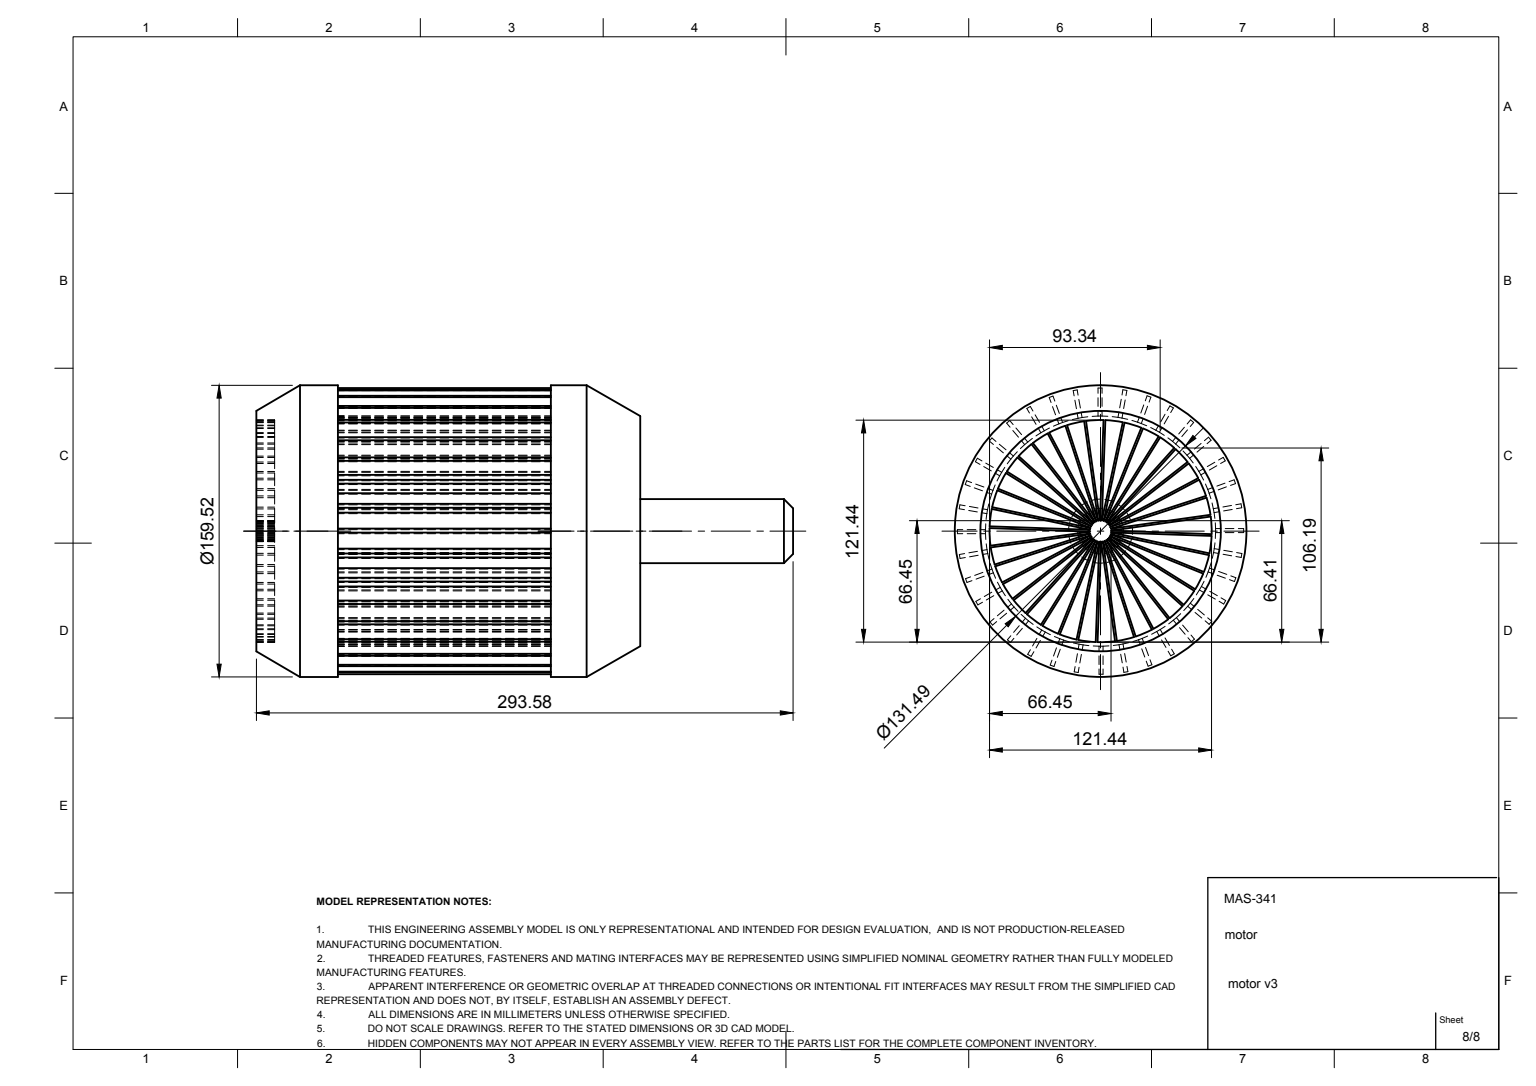
ISO-10303-21;
HEADER;
FILE_DESCRIPTION (('STEP AP214'),
    '1' );
FILE_NAME ('MOTOR.step',
    '2026-10-08T00:39:10',
    ( '' ),
    ( '' ),
    'SwSTEP 2.0',
    'SolidWorks 2025',
    '' );
FILE_SCHEMA (( 'AUTOMOTIVE_DESIGN' ));
ENDSEC;

DATA;
#1=VERTEX_POINT ( 'NONE', #4469 ) ;
#3=DIRECTION ( 'NONE',  ( 0.000000000000000000, 0.000000000000000000, 1.000000000000000000 ) ) ;
#6=EDGE_CURVE ( 'NONE', #9325, #3604, #16957, .T. ) ;
#8=AXIS2_PLACEMENT_3D ( 'NONE', #20241, #7754, #6443 ) ;
#11=LINE ( 'NONE', #3084, #15099 ) ;
#13=DIRECTION ( 'NONE',  ( 1.000000000000000000, 0.000000000000000000, 0.000000000000000000 ) ) ;
#14=CARTESIAN_POINT ( 'NONE',  ( 1.379293853801755176, -58.69016442926522359, 112.7772637782949943 ) ) ;
#17=VERTEX_POINT ( 'NONE', #1406 ) ;
#18=LINE ( 'NONE', #19855, #18549 ) ;
#19=CARTESIAN_POINT ( 'NONE',  ( -47.56244194535165803, -37.78198917157333625, 283.5832628385307999 ) ) ;
#20=ORIENTED_EDGE ( 'NONE', *, *, #18426, .T. ) ;
#21=ORIENTED_EDGE ( 'NONE', *, *, #3297, .T. ) ;
#23=EDGE_CURVE ( 'NONE', #17780, #6819, #12333, .T. ) ;
#27=FACE_BOUND ( 'NONE', #13868, .T. ) ;
#28=ORIENTED_EDGE ( 'NONE', *, *, #7214, .F. ) ;
#34=EDGE_CURVE ( 'NONE', #17780, #13430, #14084, .T. ) ;
#36=DIRECTION ( 'NONE',  ( 1.000000000000000000, 0.000000000000000000, 0.000000000000000000 ) ) ;
#37=EDGE_CURVE ( 'NONE', #15836, #9172, #3251, .T. ) ;
#40=DIRECTION ( 'NONE',  ( -0.9396926207859104263, 0.3420201433256630508, 0.000000000000000000 ) ) ;
#43=ADVANCED_FACE ( 'NONE', ( #7739 ), #8149, .F. ) ;
#45=VECTOR ( 'NONE', #980, 1000.000000000000000 ) ;
#48=VERTEX_POINT ( 'NONE', #12848 ) ;
#50=ORIENTED_EDGE ( 'NONE', *, *, #6042, .F. ) ;
#52=CYLINDRICAL_SURFACE ( 'NONE', #15157, 62.91752772691707207 ) ;
#53=CARTESIAN_POINT ( 'NONE',  ( 19.23677882349201695, -57.61823435390814296, 283.5832628385307999 ) ) ;
#54=DIRECTION ( 'NONE',  ( -0.3747554100459959403, -0.9271237148521535021, 0.000000000000000000 ) ) ;
#55=VERTEX_POINT ( 'NONE', #19106 ) ;
#60=DIRECTION ( 'NONE',  ( -0.000000000000000000, -0.000000000000000000, 1.000000000000000000 ) ) ;
#61=EDGE_CURVE ( 'NONE', #5572, #2811, #1813, .T. ) ;
#67=ORIENTED_EDGE ( 'NONE', *, *, #294, .F. ) ;
#71=ORIENTED_EDGE ( 'NONE', *, *, #11636, .F. ) ;
#72=PLANE ( 'NONE',  #545 ) ;
#73=DIRECTION ( 'NONE',  ( 1.000000000000000000, 0.000000000000000000, 0.000000000000000000 ) ) ;
#75=LINE ( 'NONE', #4042, #2106 ) ;
#77=ORIENTED_EDGE ( 'NONE', *, *, #15533, .T. ) ;
#79=LINE ( 'NONE', #15635, #4891 ) ;
#81=UNCERTAINTY_MEASURE_WITH_UNIT (LENGTH_MEASURE( 1.000000000000000082E-05 ), #12072, 'distance_accuracy_value', 'NONE');
#91=ORIENTED_EDGE ( 'NONE', *, *, #10595, .F. ) ;
#93=VERTEX_POINT ( 'NONE', #12647 ) ;
#94=VECTOR ( 'NONE', #4205, 1000.000000000000000 ) ;
#96=FACE_OUTER_BOUND ( 'NONE', #8145, .T. ) ;
#97=EDGE_CURVE ( 'NONE', #13695, #10750, #5094, .T. ) ;
#99=FACE_OUTER_BOUND ( 'NONE', #15672, .T. ) ;
#101=ORIENTED_EDGE ( 'NONE', *, *, #14389, .F. ) ;
#103=CARTESIAN_POINT ( 'NONE',  ( 0.000000000000000000, 0.000000000000000000, 283.5832628385307999 ) ) ;
#108=VERTEX_POINT ( 'NONE', #3347 ) ;
#109=CARTESIAN_POINT ( 'NONE',  ( 79.75827554147308263, 0.000000000000000000, 112.9440587442963562 ) ) ;
#110=CYLINDRICAL_SURFACE ( 'NONE', #6774, 62.91752772691707207 ) ;
#113=ORIENTED_EDGE ( 'NONE', *, *, #2779, .F. ) ;
#116=AXIS2_PLACEMENT_3D ( 'NONE', #3572, #14207, #6645 ) ;
#118=EDGE_LOOP ( 'NONE', ( #19896, #4440, #15908, #1948 ) ) ;
#122=AXIS2_PLACEMENT_3D ( 'NONE', #14861, #16210, #14669 ) ;
#123=EDGE_LOOP ( 'NONE', ( #19058, #8519, #18483, #4308 ) ) ;
#124=ADVANCED_FACE ( 'NONE', ( #3050 ), #72, .T. ) ;
#125=CARTESIAN_POINT ( 'NONE',  ( 28.06680738835026290, -53.87178215532764369, 293.5832628385307999 ) ) ;
#126=LINE ( 'NONE', #5341, #13935 ) ;
#129=FACE_OUTER_BOUND ( 'NONE', #6146, .T. ) ;
#133=LINE ( 'NONE', #6488, #17538 ) ;
#137=VECTOR ( 'NONE', #8001, 1000.000000000000000 ) ;
#139=PLANE ( 'NONE',  #10813 ) ;
#142=DIRECTION ( 'NONE',  ( -0.000000000000000000, -0.000000000000000000, 1.000000000000000000 ) ) ;
#144=ORIENTED_EDGE ( 'NONE', *, *, #11299, .F. ) ;
#145=EDGE_CURVE ( 'NONE', #10155, #5152, #9485, .T. ) ;
#146=ADVANCED_FACE ( 'NONE', ( #6627 ), #17167, .F. ) ;
#148=ADVANCED_FACE ( 'NONE', ( #7839 ), #6224, .F. ) ;
#151=AXIS2_PLACEMENT_3D ( 'NONE', #5744, #3184, #10529 ) ;
#154=LINE ( 'NONE', #15601, #13008 ) ;
#155=DIRECTION ( 'NONE',  ( 0.000000000000000000, 0.000000000000000000, 1.000000000000000000 ) ) ;
#157=EDGE_CURVE ( 'NONE', #11944, #5361, #6437, .T. ) ;
#158=LINE ( 'NONE', #9470, #15417 ) ;
#159=DIRECTION ( 'NONE',  ( -0.000000000000000000, -0.000000000000000000, 1.000000000000000000 ) ) ;
#161=AXIS2_PLACEMENT_3D ( 'NONE', #19945, #4400, #6050 ) ;
#162=CARTESIAN_POINT ( 'NONE',  ( 0.000000000000000000, 0.000000000000000000, 283.5832628385307999 ) ) ;
#163=ORIENTED_EDGE ( 'NONE', *, *, #16525, .F. ) ;
#168=EDGE_CURVE ( 'NONE', #13542, #6667, #19206, .T. ) ;
#169=ORIENTED_EDGE ( 'NONE', *, *, #10850, .T. ) ;
#170=LINE ( 'NONE', #6528, #17757 ) ;
#171=ORIENTED_EDGE ( 'NONE', *, *, #16914, .T. ) ;
#172=CARTESIAN_POINT ( 'NONE',  ( 51.23821591265094355, 28.63313560863489471, 132.4711112102474146 ) ) ;
#174=EDGE_CURVE ( 'NONE', #2962, #5478, #10345, .T. ) ;
#175=DIRECTION ( 'NONE',  ( -0.000000000000000000, -0.000000000000000000, 1.000000000000000000 ) ) ;
#177=CARTESIAN_POINT ( 'NONE',  ( 44.79940644582654841, -41.02350267428983699, 293.5832628385307999 ) ) ;
#179=ORIENTED_EDGE ( 'NONE', *, *, #8168, .F. ) ;
#181=CARTESIAN_POINT ( 'NONE',  ( -57.92514141135452377, -18.28503710798565152, 293.5832628385307999 ) ) ;
#182=VERTEX_POINT ( 'NONE', #8245 ) ;
#184=DIRECTION ( 'NONE',  ( -0.000000000000000000, -0.000000000000000000, 1.000000000000000000 ) ) ;
#185=VECTOR ( 'NONE', #17338, 999.9999999999998863 ) ;
#186=DIRECTION ( 'NONE',  ( 0.4999999999999978906, 0.8660254037844397068, 0.000000000000000000 ) ) ;
#192=ORIENTED_EDGE ( 'NONE', *, *, #7035, .T. ) ;
#194=DIRECTION ( 'NONE',  ( 0.000000000000000000, 0.000000000000000000, -1.000000000000000000 ) ) ;
#195=VERTEX_POINT ( 'NONE', #2590 ) ;
#197=DIRECTION ( 'NONE',  ( -0.000000000000000000, -0.000000000000000000, 1.000000000000000000 ) ) ;
#198=CARTESIAN_POINT ( 'NONE',  ( 25.99419088092191643, -73.82206860051539365, 248.9926560891072143 ) ) ;
#199=EDGE_LOOP ( 'NONE', ( #8551, #11635, #6168 ) ) ;
#200=DIRECTION ( 'NONE',  ( 0.000000000000000000, 0.000000000000000000, 1.000000000000000000 ) ) ;
#201=DIRECTION ( 'NONE',  ( -0.000000000000000000, -0.000000000000000000, 1.000000000000000000 ) ) ;
#202=DIRECTION ( 'NONE',  ( -0.6427876096865458022, 0.7660444431189726844, 0.000000000000000000 ) ) ;
#203=LINE ( 'NONE', #14432, #8189 ) ;
#207=FACE_OUTER_BOUND ( 'NONE', #7256, .T. ) ;
#209=LINE ( 'NONE', #17715, #417 ) ;
#210=ORIENTED_EDGE ( 'NONE', *, *, #884, .F. ) ;
#211=VECTOR ( 'NONE', #4896, 1000.000000000000114 ) ;
#214=ORIENTED_EDGE ( 'NONE', *, *, #634, .F. ) ;
#216=VECTOR ( 'NONE', #7323, 999.9999999999998863 ) ;
#217=ORIENTED_EDGE ( 'NONE', *, *, #13252, .T. ) ;
#219=VERTEX_POINT ( 'NONE', #7381 ) ;
#221=LINE ( 'NONE', #125, #3582 ) ;
#223=ORIENTED_EDGE ( 'NONE', *, *, #17123, .T. ) ;
#229=FACE_OUTER_BOUND ( 'NONE', #16622, .T. ) ;
#233=CIRCLE ( 'NONE', #865, 60.74260934110282051 ) ;
#234=EDGE_CURVE ( 'NONE', #6701, #18758, #15059, .T. ) ;
#238=PLANE ( 'NONE',  #10473 ) ;
#241=VERTEX_POINT ( 'NONE', #4112 ) ;
#243=CARTESIAN_POINT ( 'NONE',  ( -55.43188410062182925, -19.30071112029661151, 248.9926560891072143 ) ) ;
#244=VERTEX_POINT ( 'NONE', #16407 ) ;
#246=ORIENTED_EDGE ( 'NONE', *, *, #6218, .F. ) ;
#247=EDGE_CURVE ( 'NONE', #18829, #4599, #4215, .T. ) ;
#249=AXIS2_PLACEMENT_3D ( 'NONE', #15715, #7622, #7927 ) ;
#252=CARTESIAN_POINT ( 'NONE',  ( 0.000000000000000000, 0.000000000000000000, 293.5832628385307999 ) ) ;
#253=CARTESIAN_POINT ( 'NONE',  ( -3.911853314815645799, 4.196299268919075232, 293.5832628385307999 ) ) ;
#255=DIRECTION ( 'NONE',  ( 1.000000000000000000, 0.000000000000000000, 0.000000000000000000 ) ) ;
#256=DIRECTION ( 'NONE',  ( -0.000000000000000000, -0.000000000000000000, 1.000000000000000000 ) ) ;
#257=FACE_OUTER_BOUND ( 'NONE', #10692, .T. ) ;
#261=AXIS2_PLACEMENT_3D ( 'NONE', #5388, #13050, #3942 ) ;
#263=ORIENTED_EDGE ( 'NONE', *, *, #10525, .T. ) ;
#264=AXIS2_PLACEMENT_3D ( 'NONE', #15615, #1602, #16694 ) ;
#268=ORIENTED_EDGE ( 'NONE', *, *, #10367, .T. ) ;
#271=DIRECTION ( 'NONE',  ( -0.9511061040868794558, -0.3088643371590157338, 0.000000000000000000 ) ) ;
#273=VECTOR ( 'NONE', #15752, 1000.000000000000000 ) ;
#274=VERTEX_POINT ( 'NONE', #2392 ) ;
#276=VECTOR ( 'NONE', #14469, 1000.000000000000000 ) ;
#279=PLANE ( 'NONE',  #19707 ) ;
#280=CARTESIAN_POINT ( 'NONE',  ( 57.61823435390807902, 19.23677882349220880, 293.5832628385307999 ) ) ;
#285=CARTESIAN_POINT ( 'NONE',  ( -0.8220851292435327196, -62.91215678473957240, 132.4711112102474146 ) ) ;
#286=DIRECTION ( 'NONE',  ( -0.8660254037844345998, -0.5000000000000069944, 0.000000000000000000 ) ) ;
#288=CARTESIAN_POINT ( 'NONE',  ( 62.09913334491125170, 10.11498556985180208, 132.4711112102474146 ) ) ;
#289=LINE ( 'NONE', #19024, #1463 ) ;
#290=CARTESIAN_POINT ( 'NONE',  ( 55.43188410062170135, 19.30071112029698455, 248.9926560891072143 ) ) ;
#292=FACE_OUTER_BOUND ( 'NONE', #9039, .T. ) ;
#294=EDGE_CURVE ( 'NONE', #11013, #2211, #842, .T. ) ;
#296=VECTOR ( 'NONE', #6808, 1000.000000000000114 ) ;
#297=DIRECTION ( 'NONE',  ( 1.000000000000000000, 0.000000000000000000, 0.000000000000000000 ) ) ;
#298=ORIENTED_EDGE ( 'NONE', *, *, #10704, .T. ) ;
#299=ORIENTED_EDGE ( 'NONE', *, *, #9841, .T. ) ;
#305=EDGE_LOOP ( 'NONE', ( #2327, #8715, #1443, #6118 ) ) ;
#311=LINE ( 'NONE', #12579, #10853 ) ;
#312=CARTESIAN_POINT ( 'NONE',  ( 57.61823435390807902, 19.23677882349220880, 293.5832628385307999 ) ) ;
#319=AXIS2_PLACEMENT_3D ( 'NONE', #17195, #12465, #6453 ) ;
#320=VECTOR ( 'NONE', #3029, 1000.000000000000000 ) ;
#321=VERTEX_POINT ( 'NONE', #7094 ) ;
#325=CARTESIAN_POINT ( 'NONE',  ( -19.23614321207235278, 57.61627707419557964, 283.5832628385307999 ) ) ;
#327=ORIENTED_EDGE ( 'NONE', *, *, #9501, .F. ) ;
#329=DIRECTION ( 'NONE',  ( -0.3420201433256601087, -0.9396926207859114255, 0.000000000000000000 ) ) ;
#332=CIRCLE ( 'NONE', #12417, 60.74260934110282051 ) ;
#337=LINE ( 'NONE', #14255, #1684 ) ;
#338=DIRECTION ( 'NONE',  ( 1.000000000000000000, 0.000000000000000000, 0.000000000000000000 ) ) ;
#340=EDGE_CURVE ( 'NONE', #18152, #7860, #943, .T. ) ;
#341=ORIENTED_EDGE ( 'NONE', *, *, #8132, .T. ) ;
#342=DIRECTION ( 'NONE',  ( -0.000000000000000000, -0.000000000000000000, 1.000000000000000000 ) ) ;
#343=ORIENTED_EDGE ( 'NONE', *, *, #631, .F. ) ;
#347=VERTEX_POINT ( 'NONE', #3651 ) ;
#348=EDGE_CURVE ( 'NONE', #14755, #3199, #18041, .T. ) ;
#350=LINE ( 'NONE', #4765, #14650 ) ;
#351=DIRECTION ( 'NONE',  ( -0.000000000000000000, -0.000000000000000000, 1.000000000000000000 ) ) ;
#355=CARTESIAN_POINT ( 'NONE',  ( 68.18670162478805707, 38.41834839689404646, 248.9926560891072143 ) ) ;
#357=CARTESIAN_POINT ( 'NONE',  ( 44.79787735033391272, -41.02212542604626577, 293.5832628385307999 ) ) ;
#360=EDGE_CURVE ( 'NONE', #2215, #19198, #19663, .T. ) ;
#361=ORIENTED_EDGE ( 'NONE', *, *, #7399, .T. ) ;
#363=DIRECTION ( 'NONE',  ( -0.9511061040868794558, -0.3088643371590157338, 0.000000000000000000 ) ) ;
#364=ORIENTED_EDGE ( 'NONE', *, *, #5614, .T. ) ;
#366=ORIENTED_EDGE ( 'NONE', *, *, #2785, .T. ) ;
#369=VECTOR ( 'NONE', #15962, 1000.000000000000000 ) ;
#370=EDGE_CURVE ( 'NONE', #6318, #12537, #20174, .T. ) ;
#374=AXIS2_PLACEMENT_3D ( 'NONE', #8108, #8211, #6887 ) ;
#376=EDGE_CURVE ( 'NONE', #12874, #17522, #10545, .T. ) ;
#382=CARTESIAN_POINT ( 'NONE',  ( -61.81362617575094021, 11.73417718768112294, 132.4711112102474146 ) ) ;
#384=CARTESIAN_POINT ( 'NONE',  ( 54.07248341783252954, -32.16802499836759921, 293.5832628385307999 ) ) ;
#385=CARTESIAN_POINT ( 'NONE',  ( 0.000000000000000000, 0.000000000000000000, 112.9440587442963562 ) ) ;
#386=DIRECTION ( 'NONE',  ( 1.000000000000000000, 0.000000000000000000, 0.000000000000000000 ) ) ;
#391=CARTESIAN_POINT ( 'NONE',  ( 0.000000000000000000, 0.000000000000000000, 283.5832628385307999 ) ) ;
#396=ORIENTED_EDGE ( 'NONE', *, *, #18390, .F. ) ;
#399=VERTEX_POINT ( 'NONE', #1458 ) ;
#400=ADVANCED_FACE ( 'NONE', ( #1248, #13721, #13823, #16903, #5862, #12074, #18338, #2794, #5963, #1667, #7484, #27, #3201, #9331, #6177, #16802, #18542, #15470, #12492, #4312, #4420, #19964, #12394, #18653, #4632, #18756, #12183, #7687, #7894, #10650, #10757, #18441, #7798, #9121, #15363, #1355, #7582 ), #17011, .F. ) ;
#401=EDGE_CURVE ( 'NONE', #5555, #4348, #6279, .T. ) ;
#404=ORIENTED_EDGE ( 'NONE', *, *, #17763, .T. ) ;
#407=DIRECTION ( 'NONE',  ( 0.5300553768524375320, 0.8479630283625697595, 0.000000000000000000 ) ) ;
#408=CARTESIAN_POINT ( 'NONE',  ( 49.07263256785952876, -39.37628763770437956, 248.9926560891072143 ) ) ;
#412=DIRECTION ( 'NONE',  ( 0.3420201433256790380, -0.9396926207859046531, 0.000000000000000000 ) ) ;
#413=ORIENTED_EDGE ( 'NONE', *, *, #34, .T. ) ;
#416=CARTESIAN_POINT ( 'NONE',  ( -11.73417718768092399, -61.81362617575098994, 132.4711112102474146 ) ) ;
#417=VECTOR ( 'NONE', #16178, 1000.000000000000227 ) ;
#421=ORIENTED_EDGE ( 'NONE', *, *, #14487, .F. ) ;
#425=ORIENTED_EDGE ( 'NONE', *, *, #14850, .T. ) ;
#426=ORIENTED_EDGE ( 'NONE', *, *, #9892, .F. ) ;
#430=EDGE_CURVE ( 'NONE', #13898, #11413, #14350, .T. ) ;
#432=CARTESIAN_POINT ( 'NONE',  ( -68.18670162478832708, -38.41834839689356329, 248.9926560891072143 ) ) ;
#434=ORIENTED_EDGE ( 'NONE', *, *, #4227, .F. ) ;
#439=VECTOR ( 'NONE', #2770, 1000.000000000000114 ) ;
#444=VECTOR ( 'NONE', #7066, 1000.000000000000000 ) ;
#445=VECTOR ( 'NONE', #5247, 1000.000000000000000 ) ;
#449=ORIENTED_EDGE ( 'NONE', *, *, #634, .T. ) ;
#452=ORIENTED_EDGE ( 'NONE', *, *, #4347, .T. ) ;
#454=ORIENTED_EDGE ( 'NONE', *, *, #3182, .F. ) ;
#457=EDGE_CURVE ( 'NONE', #4545, #10038, #17552, .T. ) ;
#459=LINE ( 'NONE', #2301, #5504 ) ;
#461=CARTESIAN_POINT ( 'NONE',  ( -47.66508197439445382, 41.06890862491522398, 132.4711112102474146 ) ) ;
#462=CARTESIAN_POINT ( 'NONE',  ( 22.81000261549368346, -58.63718168490493099, 132.4711112102474146 ) ) ;
#463=DIRECTION ( 'NONE',  ( -0.000000000000000000, -0.000000000000000000, 1.000000000000000000 ) ) ;
#467=FACE_OUTER_BOUND ( 'NONE', #12951, .T. ) ;
#468=ORIENTED_EDGE ( 'NONE', *, *, #8040, .F. ) ;
#469=ADVANCED_FACE ( 'NONE', ( #4843 ), #3306, .F. ) ;
#470=DIRECTION ( 'NONE',  ( 0.000000000000000000, 0.000000000000000000, 1.000000000000000000 ) ) ;
#472=EDGE_LOOP ( 'NONE', ( #15073, #6600, #4290, #1623 ) ) ;
#474=ORIENTED_EDGE ( 'NONE', *, *, #16234, .F. ) ;
#475=VECTOR ( 'NONE', #10571, 1000.000000000000114 ) ;
#477=DIRECTION ( 'NONE',  ( 0.000000000000000000, 0.000000000000000000, -1.000000000000000000 ) ) ;
#479=LINE ( 'NONE', #10910, #17442 ) ;
#480=EDGE_CURVE ( 'NONE', #10080, #12789, #2077, .T. ) ;
#481=CARTESIAN_POINT ( 'NONE',  ( 39.84224160888901167, 67.36461649554546227, 110.9660488491356887 ) ) ;
#486=ORIENTED_EDGE ( 'NONE', *, *, #8858, .T. ) ;
#487=CARTESIAN_POINT ( 'NONE',  ( 0.000000000000000000, 0.000000000000000000, 293.5832628385307999 ) ) ;
#488=CARTESIAN_POINT ( 'NONE',  ( 12.78021302872850562, -77.21438937758507848, 112.0427633081291816 ) ) ;
#490=DIRECTION ( 'NONE',  ( 0.000000000000000000, 0.000000000000000000, -1.000000000000000000 ) ) ;
#492=EDGE_CURVE ( 'NONE', #11539, #4753, #17531, .T. ) ;
#493=EDGE_CURVE ( 'NONE', #14511, #9172, #1973, .T. ) ;
#495=DIRECTION ( 'NONE',  ( -0.000000000000000000, -0.000000000000000000, 1.000000000000000000 ) ) ;
#498=EDGE_CURVE ( 'NONE', #18312, #4139, #126, .T. ) ;
#499=FACE_OUTER_BOUND ( 'NONE', #8497, .T. ) ;
#500=ORIENTED_EDGE ( 'NONE', *, *, #7011, .T. ) ;
#503=CARTESIAN_POINT ( 'NONE',  ( 0.000000000000000000, 0.000000000000000000, 132.4711112102474146 ) ) ;
#506=EDGE_CURVE ( 'NONE', #2560, #13065, #10425, .T. ) ;
#507=CARTESIAN_POINT ( 'NONE',  ( 1.379293853801755176, -78.26059000578311498, 112.7772637782949943 ) ) ;
#508=EDGE_CURVE ( 'NONE', #5829, #10038, #8601, .T. ) ;
#509=CARTESIAN_POINT ( 'NONE',  ( 0.000000000000000000, 0.000000000000000000, 283.5832628385307999 ) ) ;
#512=DIRECTION ( 'NONE',  ( 0.000000000000000000, 0.000000000000000000, 1.000000000000000000 ) ) ;
#515=AXIS2_PLACEMENT_3D ( 'NONE', #5608, #10400, #8772 ) ;
#516=DIRECTION ( 'NONE',  ( -0.000000000000000000, -0.000000000000000000, 1.000000000000000000 ) ) ;
#518=FACE_OUTER_BOUND ( 'NONE', #7990, .T. ) ;
#521=CARTESIAN_POINT ( 'NONE',  ( 0.000000000000000000, 0.000000000000000000, 283.5832628385307999 ) ) ;
#522=LINE ( 'NONE', #8082, #10202 ) ;
#523=ADVANCED_FACE ( 'NONE', ( #18020 ), #15040, .F. ) ;
#524=ORIENTED_EDGE ( 'NONE', *, *, #19307, .F. ) ;
#525=EDGE_CURVE ( 'NONE', #10391, #7427, #10330, .T. ) ;
#526=DIRECTION ( 'NONE',  ( 0.000000000000000000, 1.000000000000000000, 0.000000000000000000 ) ) ;
#530=EDGE_LOOP ( 'NONE', ( #18918, #10030, #2836 ) ) ;
#534=LINE ( 'NONE', #13094, #8143 ) ;
#535=EDGE_CURVE ( 'NONE', #93, #1238, #12637, .T. ) ;
#537=EDGE_LOOP ( 'NONE', ( #14888, #16258 ) ) ;
#539=DIRECTION ( 'NONE',  ( 0.9396926207859082059, 0.3420201433256694901, 0.000000000000000000 ) ) ;
#542=AXIS2_PLACEMENT_3D ( 'NONE', #2718, #18574, #10474 ) ;
#543=DIRECTION ( 'NONE',  ( 0.1390141521205946196, -0.9902903945359624593, 0.000000000000000000 ) ) ;
#544=DIRECTION ( 'NONE',  ( -0.6692498792541777819, -0.7430374143461878633, 0.000000000000000000 ) ) ;
#545=AXIS2_PLACEMENT_3D ( 'NONE', #9683, #1507, #12750 ) ;
#547=EDGE_CURVE ( 'NONE', #14566, #10313, #13391, .T. ) ;
#549=CARTESIAN_POINT ( 'NONE',  ( 47.56406379474552182, 37.78325588002191893, 293.5832628385307999 ) ) ;
#550=CARTESIAN_POINT ( 'NONE',  ( 0.000000000000000000, 0.000000000000000000, 293.5832628385307999 ) ) ;
#551=FACE_OUTER_BOUND ( 'NONE', #9374, .T. ) ;
#553=AXIS2_PLACEMENT_3D ( 'NONE', #18898, #14285, #12937 ) ;
#554=CARTESIAN_POINT ( 'NONE',  ( -41.06890862491505345, -47.66508197439457462, 248.9926560891072143 ) ) ;
#558=EDGE_LOOP ( 'NONE', ( #486, #1812, #16928, #3761 ) ) ;
#559=AXIS2_PLACEMENT_3D ( 'NONE', #821, #3898, #19644 ) ;
#560=ORIENTED_EDGE ( 'NONE', *, *, #15092, .F. ) ;
#561=AXIS2_PLACEMENT_3D ( 'NONE', #312, #4936, #6361 ) ;
#563=CARTESIAN_POINT ( 'NONE',  ( 59.51724408343574879, -12.14957802882732452, 283.5832628385307999 ) ) ;
#569=LINE ( 'NONE', #8032, #16267 ) ;
#570=ORIENTED_EDGE ( 'NONE', *, *, #11345, .F. ) ;
#572=AXIS2_PLACEMENT_3D ( 'NONE', #19392, #3830, #12091 ) ;
#574=ORIENTED_EDGE ( 'NONE', *, *, #37, .T. ) ;
#576=DIRECTION ( 'NONE',  ( -0.6427876096865328126, -0.7660444431189835646, 0.000000000000000000 ) ) ;
#577=DIRECTION ( 'NONE',  ( -0.5000000000000101030, 0.8660254037844328234, 0.000000000000000000 ) ) ;
#579=ORIENTED_EDGE ( 'NONE', *, *, #19467, .F. ) ;
#580=LINE ( 'NONE', #2325, #4763 ) ;
#581=LINE ( 'NONE', #8155, #8466 ) ;
#585=LINE ( 'NONE', #17782, #14674 ) ;
#586=DIRECTION ( 'NONE',  ( 1.000000000000000000, 0.000000000000000000, 0.000000000000000000 ) ) ;
#587=LINE ( 'NONE', #10456, #10288 ) ;
#589=LINE ( 'NONE', #11628, #17406 ) ;
#591=ORIENTED_EDGE ( 'NONE', *, *, #10844, .T. ) ;
#594=ORIENTED_EDGE ( 'NONE', *, *, #16874, .F. ) ;
#595=AXIS2_PLACEMENT_3D ( 'NONE', #1167, #16828, #19689 ) ;
#596=ORIENTED_EDGE ( 'NONE', *, *, #14234, .T. ) ;
#597=LINE ( 'NONE', #3867, #11838 ) ;
#601=EDGE_CURVE ( 'NONE', #16327, #219, #6106, .T. ) ;
#603=ADVANCED_FACE ( 'NONE', ( #10043 ), #11851, .T. ) ;
#604=CARTESIAN_POINT ( 'NONE',  ( 0.000000000000000000, 0.000000000000000000, 132.4711112102474146 ) ) ;
#605=EDGE_CURVE ( 'NONE', #13307, #14163, #11759, .T. ) ;
#606=CARTESIAN_POINT ( 'NONE',  ( -45.46712722958807973, 40.27908801170008957, 283.5832628385307999 ) ) ;
#607=DIRECTION ( 'NONE',  ( -0.3420201433256601642, -0.9396926207859114255, 0.000000000000000000 ) ) ;
#611=VECTOR ( 'NONE', #4918, 1000.000000000000000 ) ;
#617=DIRECTION ( 'NONE',  ( 1.000000000000000000, 0.000000000000000000, 0.000000000000000000 ) ) ;
#621=LINE ( 'NONE', #8495, #13010 ) ;
#623=ORIENTED_EDGE ( 'NONE', *, *, #12748, .F. ) ;
#624=EDGE_LOOP ( 'NONE', ( #7544, #7506, #16288, #12643 ) ) ;
#627=VECTOR ( 'NONE', #3562, 1000.000000000000000 ) ;
#628=AXIS2_PLACEMENT_3D ( 'NONE', #13240, #7026, #19693 ) ;
#629=DIRECTION ( 'NONE',  ( -0.9511061040868804550, -0.3088643371590125697, 0.000000000000000000 ) ) ;
#630=VECTOR ( 'NONE', #14767, 1000.000000000000114 ) ;
#631=EDGE_CURVE ( 'NONE', #14818, #6254, #14743, .T. ) ;
#633=EDGE_LOOP ( 'NONE', ( #11208, #14397, #3955, #8739 ) ) ;
#634=EDGE_CURVE ( 'NONE', #17381, #14953, #13488, .T. ) ;
#635=LINE ( 'NONE', #17826, #1419 ) ;
#636=CARTESIAN_POINT ( 'NONE',  ( 60.68773558783009747, -2.629322876227576433, 283.5832628385307999 ) ) ;
#639=EDGE_CURVE ( 'NONE', #4730, #9351, #19739, .T. ) ;
#644=CARTESIAN_POINT ( 'NONE',  ( -0.8220851292435327196, -78.26059000578311498, 248.9926560891072143 ) ) ;
#646=LINE ( 'NONE', #6889, #1478 ) ;
#647=VECTOR ( 'NONE', #10889, 1000.000000000000114 ) ;
#651=ORIENTED_EDGE ( 'NONE', *, *, #11384, .F. ) ;
#652=ORIENTED_EDGE ( 'NONE', *, *, #1769, .F. ) ;
#653=ORIENTED_EDGE ( 'NONE', *, *, #1354, .F. ) ;
#658=CARTESIAN_POINT ( 'NONE',  ( -20.84572577951200500, -54.86954475316249358, 132.4711112102474146 ) ) ;
#661=ORIENTED_EDGE ( 'NONE', *, *, #1097, .F. ) ;
#662=DIRECTION ( 'NONE',  ( -0.000000000000000000, -0.000000000000000000, 1.000000000000000000 ) ) ;
#665=PLANE ( 'NONE',  #18608 ) ;
#667=PLANE ( 'NONE',  #2202 ) ;
#673=ORIENTED_EDGE ( 'NONE', *, *, #8391, .F. ) ;
#675=VERTEX_POINT ( 'NONE', #13593 ) ;
#677=DIRECTION ( 'NONE',  ( -0.9848077530122097967, 0.1736481776669207000, 0.000000000000000000 ) ) ;
#678=AXIS2_PLACEMENT_3D ( 'NONE', #19949, #2979, #9000 ) ;
#680=DIRECTION ( 'NONE',  ( -1.000000000000000000, 0.000000000000000000, 0.000000000000000000 ) ) ;
#683=LINE ( 'NONE', #6927, #6077 ) ;
#684=CARTESIAN_POINT ( 'NONE',  ( 39.84224160888901167, 67.36461649554546227, 132.4711112102474146 ) ) ;
#685=EDGE_CURVE ( 'NONE', #3831, #739, #15136, .T. ) ;
#687=DIRECTION ( 'NONE',  ( -0.3420201433256757073, 0.9396926207859057634, 0.000000000000000000 ) ) ;
#688=LINE ( 'NONE', #5693, #18512 ) ;
#689=DIRECTION ( 'NONE',  ( -0.000000000000000000, -0.000000000000000000, 1.000000000000000000 ) ) ;
#690=DIRECTION ( 'NONE',  ( -0.000000000000000000, -0.000000000000000000, 1.000000000000000000 ) ) ;
#693=DIRECTION ( 'NONE',  ( -0.03505990758545545621, -0.9993852124581888985, 0.000000000000000000 ) ) ;
#694=ORIENTED_EDGE ( 'NONE', *, *, #7836, .T. ) ;
#695=VECTOR ( 'NONE', #18044, 1000.000000000000114 ) ;
#697=ORIENTED_EDGE ( 'NONE', *, *, #18645, .T. ) ;
#703=PLANE ( 'NONE',  #4090 ) ;
#704=LINE ( 'NONE', #17603, #2792 ) ;
#705=EDGE_CURVE ( 'NONE', #182, #6905, #10519, .T. ) ;
#707=LINE ( 'NONE', #5926, #14264 ) ;
#709=DIRECTION ( 'NONE',  ( 0.1736481776669273336, 0.9848077530122085754, 0.000000000000000000 ) ) ;
#710=CARTESIAN_POINT ( 'NONE',  ( 54.86954475316255042, -20.84572577951183092, 111.4180192758974499 ) ) ;
#712=CARTESIAN_POINT ( 'NONE',  ( 51.24245927909996112, -32.62092819947974220, 293.5832628385307999 ) ) ;
#715=CARTESIAN_POINT ( 'NONE',  ( 3.123743752084377601, -4.811834253409482010, 293.5832628385307999 ) ) ;
#716=ORIENTED_EDGE ( 'NONE', *, *, #9383, .F. ) ;
#717=ADVANCED_FACE ( 'NONE', ( #15338 ), #19942, .F. ) ;
#719=LINE ( 'NONE', #8496, #5976 ) ;
#720=VERTEX_POINT ( 'NONE', #7362 ) ;
#721=ORIENTED_EDGE ( 'NONE', *, *, #8886, .T. ) ;
#723=DIRECTION ( 'NONE',  ( 0.7660444431189707970, 0.6427876096865481337, 0.000000000000000000 ) ) ;
#726=VECTOR ( 'NONE', #11409, 999.9999999999998863 ) ;
#728=CARTESIAN_POINT ( 'NONE',  ( 58.63718168490485283, 22.81000261549389307, 248.9926560891072143 ) ) ;
#730=ORIENTED_EDGE ( 'NONE', *, *, #1243, .F. ) ;
#731=EDGE_CURVE ( 'NONE', #19514, #5793, #7459, .T. ) ;
#736=CARTESIAN_POINT ( 'NONE',  ( -31.86742755225479584, 24.93940645478156526, 248.9926560891072143 ) ) ;
#739=VERTEX_POINT ( 'NONE', #18318 ) ;
#744=VECTOR ( 'NONE', #7674, 1000.000000000000114 ) ;
#750=EDGE_CURVE ( 'NONE', #5911, #17872, #1330, .T. ) ;
#756=DIRECTION ( 'NONE',  ( 0.9396926207859114255, -0.3420201433256601642, 0.000000000000000000 ) ) ;
#758=VECTOR ( 'NONE', #990, 1000.000000000000000 ) ;
#761=EDGE_LOOP ( 'NONE', ( #20006, #19054, #13041 ) ) ;
#763=EDGE_CURVE ( 'NONE', #9877, #8052, #9249, .T. ) ;
#764=EDGE_CURVE ( 'NONE', #14186, #1114, #6047, .T. ) ;
#765=ORIENTED_EDGE ( 'NONE', *, *, #6498, .T. ) ;
#767=ORIENTED_EDGE ( 'NONE', *, *, #1905, .T. ) ;
#769=CARTESIAN_POINT ( 'NONE',  ( 14.39940464655707331, 76.92888220842492331, 112.0427633081292953 ) ) ;
#770=EDGE_LOOP ( 'NONE', ( #15637, #2166, #12568, #2461 ) ) ;
#772=EDGE_CURVE ( 'NONE', #1021, #8910, #10828, .T. ) ;
#774=CARTESIAN_POINT ( 'NONE',  ( -36.99387960884161686, 48.17797692984174773, 283.5832628385307999 ) ) ;
#779=PLANE ( 'NONE',  #17644 ) ;
#782=PLANE ( 'NONE',  #19179 ) ;
#783=DIRECTION ( 'NONE',  ( 1.000000000000000000, 0.000000000000000000, 0.000000000000000000 ) ) ;
#784=AXIS2_PLACEMENT_3D ( 'NONE', #1960, #6363, #6465 ) ;
#785=LINE ( 'NONE', #7034, #12769 ) ;
#786=EDGE_CURVE ( 'NONE', #18064, #15547, #13824, .T. ) ;
#787=CARTESIAN_POINT ( 'NONE',  ( 2.240720816136066773, -5.281164089014820817, 293.5832628385307999 ) ) ;
#788=DIRECTION ( 'NONE',  ( -0.8660254037844328234, -0.5000000000000101030, 0.000000000000000000 ) ) ;
#791=VECTOR ( 'NONE', #6303, 1000.000000000000000 ) ;
#793=ADVANCED_FACE ( 'NONE', ( #9201 ), #15445, .T. ) ;
#794=ORIENTED_EDGE ( 'NONE', *, *, #4681, .F. ) ;
#795=DIRECTION ( 'NONE',  ( -0.000000000000000000, -0.000000000000000000, 1.000000000000000000 ) ) ;
#802=ORIENTED_EDGE ( 'NONE', *, *, #15206, .F. ) ;
#805=CARTESIAN_POINT ( 'NONE',  ( 60.72279549541555355, -1.629937663769388090, 293.5832628385307999 ) ) ;
#806=LINE ( 'NONE', #906, #1790 ) ;
#809=CARTESIAN_POINT ( 'NONE',  ( 56.12853591711344592, -23.22718332831461652, 283.5832628385307999 ) ) ;
#812=PLANE ( 'NONE',  #20001 ) ;
#814=PLANE ( 'NONE',  #7143 ) ;
#816=ORIENTED_EDGE ( 'NONE', *, *, #10481, .T. ) ;
#819=ORIENTED_EDGE ( 'NONE', *, *, #12411, .T. ) ;
#820=DIRECTION ( 'NONE',  ( 1.000000000000000000, 0.000000000000000000, -0.000000000000000000 ) ) ;
#821=CARTESIAN_POINT ( 'NONE',  ( 0.000000000000000000, 0.000000000000000000, 283.5832628385307999 ) ) ;
#822=ORIENTED_EDGE ( 'NONE', *, *, #13054, .T. ) ;
#828=CARTESIAN_POINT ( 'NONE',  ( 0.000000000000000000, 0.000000000000000000, 283.5832628385307999 ) ) ;
#829=CARTESIAN_POINT ( 'NONE',  ( 51.51682027493064453, -28.15057869795607459, 110.9660488491357455 ) ) ;
#832=DIRECTION ( 'NONE',  ( -0.000000000000000000, -0.000000000000000000, 1.000000000000000000 ) ) ;
#835=CARTESIAN_POINT ( 'NONE',  ( -28.94886449118902760, 53.40063514825087765, 293.5832628385307999 ) ) ;
#837=( GEOMETRIC_REPRESENTATION_CONTEXT ( 3 ) GLOBAL_UNCERTAINTY_ASSIGNED_CONTEXT ( ( #2726 ) ) GLOBAL_UNIT_ASSIGNED_CONTEXT ( ( #7973, #15755, #14217 ) ) REPRESENTATION_CONTEXT ( 'NONE', 'WORKASPACE' ) );
#838=EDGE_CURVE ( 'NONE', #12583, #959, #9515, .T. ) ;
#841=ADVANCED_FACE ( 'NONE', ( #8070 ), #14323, .T. ) ;
#842=LINE ( 'NONE', #11976, #13920 ) ;
#843=ORIENTED_EDGE ( 'NONE', *, *, #14946, .T. ) ;
#844=EDGE_CURVE ( 'NONE', #15222, #12174, #8270, .T. ) ;
#846=LINE ( 'NONE', #3630, #15499 ) ;
#848=LINE ( 'NONE', #17748, #13020 ) ;
#849=ADVANCED_FACE ( 'NONE', ( #11448 ), #1947, .T. ) ;
#852=CARTESIAN_POINT ( 'NONE',  ( 59.30917539369505675, -13.12769224524051559, 293.5832628385307999 ) ) ;
#854=VECTOR ( 'NONE', #363, 1000.000000000000114 ) ;
#857=DIRECTION ( 'NONE',  ( 0.9902903945359623483, 0.1390141521205945918, 0.000000000000000000 ) ) ;
#858=VERTEX_POINT ( 'NONE', #1838 ) ;
#859=VECTOR ( 'NONE', #3356, 1000.000000000000000 ) ;
#860=EDGE_CURVE ( 'NONE', #1086, #5730, #18086, .T. ) ;
#861=ORIENTED_EDGE ( 'NONE', *, *, #5577, .F. ) ;
#864=EDGE_LOOP ( 'NONE', ( #14206, #12029, #8456, #17907 ) ) ;
#865=AXIS2_PLACEMENT_3D ( 'NONE', #9927, #3687, #11837 ) ;
#867=DIRECTION ( 'NONE',  ( -0.5300553768524375320, -0.8479630283625697595, 0.000000000000000000 ) ) ;
#868=DIRECTION ( 'NONE',  ( -0.000000000000000000, -0.000000000000000000, 1.000000000000000000 ) ) ;
#872=DIRECTION ( 'NONE',  ( -0.000000000000000000, -0.000000000000000000, 1.000000000000000000 ) ) ;
#873=CARTESIAN_POINT ( 'NONE',  ( 49.07263256785952166, -39.37628763770437956, 132.4711112102474146 ) ) ;
#874=EDGE_CURVE ( 'NONE', #11852, #7829, #14215, .T. ) ;
#876=DIRECTION ( 'NONE',  ( 1.000000000000000000, 0.000000000000000000, -0.000000000000000000 ) ) ;
#877=DIRECTION ( 'NONE',  ( 0.1736481776669307198, -0.9848077530122080203, -0.000000000000000000 ) ) ;
#878=DIRECTION ( 'NONE',  ( -1.000000000000000000, -3.491481338843133355E-15, 0.000000000000000000 ) ) ;
#879=PLANE ( 'NONE',  #11470 ) ;
#880=VECTOR ( 'NONE', #8878, 1000.000000000000114 ) ;
#884=EDGE_CURVE ( 'NONE', #6667, #10541, #9611, .T. ) ;
#887=ORIENTED_EDGE ( 'NONE', *, *, #9369, .T. ) ;
#890=ORIENTED_EDGE ( 'NONE', *, *, #13792, .T. ) ;
#892=CARTESIAN_POINT ( 'NONE',  ( -67.36461649554505016, 39.84224160888970800, 248.9926560891072143 ) ) ;
#898=PLANE ( 'NONE',  #9640 ) ;
#901=ADVANCED_FACE ( 'NONE', ( #16065 ), #3476, .F. ) ;
#903=CARTESIAN_POINT ( 'NONE',  ( 0.000000000000000000, 0.000000000000000000, 283.5832628385307999 ) ) ;
#905=CARTESIAN_POINT ( 'NONE',  ( 59.42266395395790823, -50.93469132750283279, 132.4711112102474146 ) ) ;
#906=CARTESIAN_POINT ( 'NONE',  ( 57.92709869106709419, 18.28567271940532990, 293.5832628385307999 ) ) ;
#910=DIRECTION ( 'NONE',  ( 0.1736481776669273336, 0.9848077530122085754, 0.000000000000000000 ) ) ;
#911=VECTOR ( 'NONE', #6305, 1000.000000000000114 ) ;
#914=DIRECTION ( 'NONE',  ( 0.9902903945359623483, 0.1390141521205945918, 0.000000000000000000 ) ) ;
#915=DIRECTION ( 'NONE',  ( -0.000000000000000000, -0.000000000000000000, 1.000000000000000000 ) ) ;
#917=ORIENTED_EDGE ( 'NONE', *, *, #11590, .T. ) ;
#920=DIRECTION ( 'NONE',  ( 1.000000000000000000, 0.000000000000000000, 0.000000000000000000 ) ) ;
#921=ORIENTED_EDGE ( 'NONE', *, *, #3637, .F. ) ;
#924=DIRECTION ( 'NONE',  ( 1.000000000000000000, 0.000000000000000000, 0.000000000000000000 ) ) ;
#925=AXIS2_PLACEMENT_3D ( 'NONE', #4318, #13517, #1146 ) ;
#926=CIRCLE ( 'NONE', #13326, 62.91752772691707207 ) ;
#927=AXIS2_PLACEMENT_3D ( 'NONE', #5331, #11563, #17816 ) ;
#930=LINE ( 'NONE', #5643, #11229 ) ;
#932=CARTESIAN_POINT ( 'NONE',  ( -14.39940464655760799, -76.92888220842480962, 112.0427633081292385 ) ) ;
#934=VERTEX_POINT ( 'NONE', #19618 ) ;
#937=VERTEX_POINT ( 'NONE', #7048 ) ;
#938=AXIS2_PLACEMENT_3D ( 'NONE', #11223, #184, #17485 ) ;
#939=AXIS2_PLACEMENT_3D ( 'NONE', #7315, #2621, #4246 ) ;
#940=VECTOR ( 'NONE', #2427, 1000.000000000000000 ) ;
#942=ORIENTED_EDGE ( 'NONE', *, *, #18405, .T. ) ;
#943=LINE ( 'NONE', #5760, #13587 ) ;
#944=ORIENTED_EDGE ( 'NONE', *, *, #13641, .T. ) ;
#945=DIRECTION ( 'NONE',  ( -0.5000000000000069944, 0.8660254037844344888, 0.000000000000000000 ) ) ;
#946=LINE ( 'NONE', #10255, #14428 ) ;
#947=DIRECTION ( 'NONE',  ( -0.000000000000000000, -0.000000000000000000, 1.000000000000000000 ) ) ;
#948=CARTESIAN_POINT ( 'NONE',  ( -2.629322876227788264, -60.68773558783006905, 293.5832628385307999 ) ) ;
#950=AXIS2_PLACEMENT_3D ( 'NONE', #14173, #155, #18468 ) ;
#951=ADVANCED_FACE ( 'NONE', ( #19331 ), #19432, .T. ) ;
#952=PLANE ( 'NONE',  #2586 ) ;
#955=DIRECTION ( 'NONE',  ( -0.000000000000000000, -0.000000000000000000, 1.000000000000000000 ) ) ;
#957=CARTESIAN_POINT ( 'NONE',  ( -51.23821591265114961, -28.63313560863453944, 132.4711112102474146 ) ) ;
#959=VERTEX_POINT ( 'NONE', #5412 ) ;
#963=ORIENTED_EDGE ( 'NONE', *, *, #10639, .F. ) ;
#966=CARTESIAN_POINT ( 'NONE',  ( 0.8220851292435327196, 58.69016442926522359, 132.4711112102474146 ) ) ;
#967=CARTESIAN_POINT ( 'NONE',  ( 58.83691981461634413, -22.28973221005101735, 132.4711112102474146 ) ) ;
#968=FACE_OUTER_BOUND ( 'NONE', #199, .T. ) ;
#971=CARTESIAN_POINT ( 'NONE',  ( 0.000000000000000000, 0.000000000000000000, 293.5832628385307999 ) ) ;
#972=ADVANCED_FACE ( 'NONE', ( #2343 ), #3769, .F. ) ;
#974=PLANE ( 'NONE',  #11706 ) ;
#978=VECTOR ( 'NONE', #19555, 1000.000000000000114 ) ;
#980=DIRECTION ( 'NONE',  ( -0.000000000000000000, -0.000000000000000000, 1.000000000000000000 ) ) ;
#982=DIRECTION ( 'NONE',  ( 0.9396926207859092051, -0.3420201433256662704, 0.000000000000000000 ) ) ;
#985=CARTESIAN_POINT ( 'NONE',  ( 76.92888220842486646, -14.39940464655733976, 248.9926560891072143 ) ) ;
#988=EDGE_LOOP ( 'NONE', ( #14488, #4292, #13951, #14059 ) ) ;
#989=EDGE_CURVE ( 'NONE', #321, #1451, #11869, .T. ) ;
#990=DIRECTION ( 'NONE',  ( -0.000000000000000000, -0.000000000000000000, 1.000000000000000000 ) ) ;
#991=ORIENTED_EDGE ( 'NONE', *, *, #1968, .F. ) ;
#993=AXIS2_PLACEMENT_3D ( 'NONE', #10794, #3035, #4454 ) ;
#995=DIRECTION ( 'NONE',  ( 0.6155349844899687950, -0.7881095627315619634, 0.000000000000000000 ) ) ;
#997=CARTESIAN_POINT ( 'NONE',  ( -38.41834839689332171, 68.18670162478844077, 110.9660488491356887 ) ) ;
#998=VERTEX_POINT ( 'NONE', #10205 ) ;
#999=EDGE_CURVE ( 'NONE', #17522, #8815, #1085, .T. ) ;
#1000=FACE_OUTER_BOUND ( 'NONE', #8542, .T. ) ;
#1001=FACE_OUTER_BOUND ( 'NONE', #11846, .T. ) ;
#1004=VECTOR ( 'NONE', #8659, 1000.000000000000114 ) ;
#1005=DIRECTION ( 'NONE',  ( -0.000000000000000000, -0.000000000000000000, 1.000000000000000000 ) ) ;
#1006=DIRECTION ( 'NONE',  ( 0.1736481776669172583, 0.9848077530122103518, 0.000000000000000000 ) ) ;
#1007=AXIS2_PLACEMENT_3D ( 'NONE', #5673, #3929, #11694 ) ;
#1013=ADVANCED_FACE ( 'NONE', ( #13365 ), #20019, .F. ) ;
#1014=EDGE_LOOP ( 'NONE', ( #1546, #3324, #12514, #214 ) ) ;
#1016=ADVANCED_FACE ( 'NONE', ( #6021 ), #16749, .T. ) ;
#1019=DIRECTION ( 'NONE',  ( 0.3747554100459959958, 0.9271237148521535021, 0.000000000000000000 ) ) ;
#1020=CARTESIAN_POINT ( 'NONE',  ( 5.485913980968211590, -1.678175111358135130, 293.5832628385307999 ) ) ;
#1021=VERTEX_POINT ( 'NONE', #1409 ) ;
#1022=DIRECTION ( 'NONE',  ( 1.000000000000000000, 0.000000000000000000, 0.000000000000000000 ) ) ;
#1025=FACE_OUTER_BOUND ( 'NONE', #18895, .T. ) ;
#1026=PLANE ( 'NONE',  #15842 ) ;
#1027=CARTESIAN_POINT ( 'NONE',  ( 0.000000000000000000, 0.000000000000000000, 248.9926560891072143 ) ) ;
#1029=CARTESIAN_POINT ( 'NONE',  ( 56.12662799072089115, -23.22641211976270270, 283.5832628385307999 ) ) ;
#1031=FACE_OUTER_BOUND ( 'NONE', #3018, .T. ) ;
#1034=VERTEX_POINT ( 'NONE', #19814 ) ;
#1035=ORIENTED_EDGE ( 'NONE', *, *, #16277, .T. ) ;
#1037=ORIENTED_EDGE ( 'NONE', *, *, #15249, .T. ) ;
#1042=DIRECTION ( 'NONE',  ( 0.9396926207859093161, -0.3420201433256663259, 0.000000000000000000 ) ) ;
#1044=CARTESIAN_POINT ( 'NONE',  ( -19.30071112029641967, 55.43188410062188609, 132.4711112102474146 ) ) ;
#1049=AXIS2_PLACEMENT_3D ( 'NONE', #3014, #142, #17237 ) ;
#1050=DIRECTION ( 'NONE',  ( 1.000000000000000000, 0.000000000000000000, 0.000000000000000000 ) ) ;
#1053=ORIENTED_EDGE ( 'NONE', *, *, #2363, .T. ) ;
#1055=CARTESIAN_POINT ( 'NONE',  ( 19.23614321207236699, -57.61627707419557964, 283.5832628385307999 ) ) ;
#1057=ORIENTED_EDGE ( 'NONE', *, *, #1482, .T. ) ;
#1058=ORIENTED_EDGE ( 'NONE', *, *, #376, .F. ) ;
#1059=VERTEX_POINT ( 'NONE', #16959 ) ;
#1062=DIRECTION ( 'NONE',  ( -0.2080686897406911207, -0.9781142164131917394, 0.000000000000000000 ) ) ;
#1064=ORIENTED_EDGE ( 'NONE', *, *, #6051, .F. ) ;
#1068=ORIENTED_EDGE ( 'NONE', *, *, #13216, .T. ) ;
#1076=FACE_OUTER_BOUND ( 'NONE', #1916, .T. ) ;
#1077=ORIENTED_EDGE ( 'NONE', *, *, #6165, .F. ) ;
#1078=ORIENTED_EDGE ( 'NONE', *, *, #10747, .F. ) ;
#1082=DIRECTION ( 'NONE',  ( 0.000000000000000000, 0.000000000000000000, 1.000000000000000000 ) ) ;
#1083=EDGE_CURVE ( 'NONE', #7829, #10900, #7741, .T. ) ;
#1085=CIRCLE ( 'NONE', #9280, 60.74260934110282051 ) ;
#1086=VERTEX_POINT ( 'NONE', #8151 ) ;
#1087=ORIENTED_EDGE ( 'NONE', *, *, #9983, .T. ) ;
#1089=CYLINDRICAL_SURFACE ( 'NONE', #11995, 60.74260934110282051 ) ;
#1090=ORIENTED_EDGE ( 'NONE', *, *, #6919, .F. ) ;
#1093=ORIENTED_EDGE ( 'NONE', *, *, #4109, .F. ) ;
#1095=DIRECTION ( 'NONE',  ( 1.000000000000000000, 0.000000000000000000, 0.000000000000000000 ) ) ;
#1097=EDGE_CURVE ( 'NONE', #12671, #18381, #3555, .T. ) ;
#1098=AXIS2_PLACEMENT_3D ( 'NONE', #19361, #16095, #3508 ) ;
#1101=ORIENTED_EDGE ( 'NONE', *, *, #14424, .T. ) ;
#1103=CARTESIAN_POINT ( 'NONE',  ( 48.17797692984161984, 36.99387960884179449, 283.5832628385307999 ) ) ;
#1106=ORIENTED_EDGE ( 'NONE', *, *, #7531, .F. ) ;
#1109=ORIENTED_EDGE ( 'NONE', *, *, #3534, .T. ) ;
#1111=EDGE_CURVE ( 'NONE', #10388, #2638, #12548, .T. ) ;
#1112=DIRECTION ( 'NONE',  ( -0.000000000000000000, -0.000000000000000000, 1.000000000000000000 ) ) ;
#1114=VERTEX_POINT ( 'NONE', #14495 ) ;
#1115=DIRECTION ( 'NONE',  ( 1.000000000000000000, 0.000000000000000000, -0.000000000000000000 ) ) ;
#1116=DIRECTION ( 'NONE',  ( -0.9993852124581887875, 0.03505990758545545621, 0.000000000000000000 ) ) ;
#1117=AXIS2_PLACEMENT_3D ( 'NONE', #16706, #4119, #16807 ) ;
#1118=EDGE_LOOP ( 'NONE', ( #11292, #9512, #14988, #2323 ) ) ;
#1119=CARTESIAN_POINT ( 'NONE',  ( 20.84572577951164618, 54.86954475316263569, 132.4711112102474146 ) ) ;
#1120=DIRECTION ( 'NONE',  ( -0.000000000000000000, -0.000000000000000000, 1.000000000000000000 ) ) ;
#1122=ADVANCED_FACE ( 'NONE', ( #11215 ), #16037, .T. ) ;
#1125=FACE_OUTER_BOUND ( 'NONE', #123, .T. ) ;
#1127=ADVANCED_FACE ( 'NONE', ( #14298 ), #279, .T. ) ;
#1128=FACE_OUTER_BOUND ( 'NONE', #10179, .T. ) ;
#1130=DIRECTION ( 'NONE',  ( 0.7660444431189835646, -0.6427876096865328126, 0.000000000000000000 ) ) ;
#1132=LINE ( 'NONE', #4304, #3995 ) ;
#1135=FACE_OUTER_BOUND ( 'NONE', #17367, .T. ) ;
#1137=ORIENTED_EDGE ( 'NONE', *, *, #1083, .F. ) ;
#1139=( NAMED_UNIT ( * ) SI_UNIT ( $, .STERADIAN. ) SOLID_ANGLE_UNIT ( ) );
#1143=ORIENTED_EDGE ( 'NONE', *, *, #23, .T. ) ;
#1145=DIRECTION ( 'NONE',  ( -0.000000000000000000, -0.000000000000000000, 1.000000000000000000 ) ) ;
#1146=DIRECTION ( 'NONE',  ( 1.000000000000000000, 0.000000000000000000, 0.000000000000000000 ) ) ;
#1148=CARTESIAN_POINT ( 'NONE',  ( -12.14957802882752524, -59.51724408343569905, 283.5832628385307999 ) ) ;
#1149=CARTESIAN_POINT ( 'NONE',  ( 5.111158570922254896, -2.605298826210304064, 283.5832628385307999 ) ) ;
#1156=DIRECTION ( 'NONE',  ( -0.000000000000000000, -0.000000000000000000, 1.000000000000000000 ) ) ;
#1158=ADVANCED_FACE ( 'NONE', ( #10912 ), #12853, .F. ) ;
#1159=ORIENTED_EDGE ( 'NONE', *, *, #15092, .T. ) ;
#1162=ORIENTED_EDGE ( 'NONE', *, *, #10042, .F. ) ;
#1163=VECTOR ( 'NONE', #5970, 1000.000000000000000 ) ;
#1166=CARTESIAN_POINT ( 'NONE',  ( 13.12726406102079224, 59.30716253403178939, 293.5832628385307999 ) ) ;
#1167=CARTESIAN_POINT ( 'NONE',  ( 0.8220851292435327196, 78.26059000578311498, 112.7772637782949943 ) ) ;
#1169=CARTESIAN_POINT ( 'NONE',  ( 0.000000000000000000, 0.000000000000000000, 293.5832628385307999 ) ) ;
#1171=ORIENTED_EDGE ( 'NONE', *, *, #13037, .F. ) ;
#1176=VECTOR ( 'NONE', #16733, 1000.000000000000000 ) ;
#1183=ORIENTED_EDGE ( 'NONE', *, *, #97, .F. ) ;
#1185=DIRECTION ( 'NONE',  ( 0.000000000000000000, 0.000000000000000000, -1.000000000000000000 ) ) ;
#1188=ORIENTED_EDGE ( 'NONE', *, *, #12282, .T. ) ;
#1190=LINE ( 'NONE', #5606, #6171 ) ;
#1196=DIRECTION ( 'NONE',  ( -0.000000000000000000, -0.000000000000000000, 1.000000000000000000 ) ) ;
#1201=EDGE_CURVE ( 'NONE', #10024, #16800, #75, .T. ) ;
#1202=FACE_OUTER_BOUND ( 'NONE', #10914, .T. ) ;
#1204=CARTESIAN_POINT ( 'NONE',  ( 51.24245927909996112, -32.62092819947974220, 293.5832628385307999 ) ) ;
#1205=CARTESIAN_POINT ( 'NONE',  ( 51.24245927909996112, -32.62092819947974220, 283.5832628385307999 ) ) ;
#1207=ORIENTED_EDGE ( 'NONE', *, *, #3241, .F. ) ;
#1210=CARTESIAN_POINT ( 'NONE',  ( -73.25972925305609351, 27.53920554013712874, 132.4711112102474146 ) ) ;
#1211=ORIENTED_EDGE ( 'NONE', *, *, #9158, .T. ) ;
#1213=VERTEX_POINT ( 'NONE', #19208 ) ;
#1216=ADVANCED_FACE ( 'NONE', ( #5483 ), #2122, .F. ) ;
#1218=EDGE_CURVE ( 'NONE', #8668, #14953, #17771, .T. ) ;
#1219=EDGE_LOOP ( 'NONE', ( #8699, #14779, #11738, #17366 ) ) ;
#1221=PLANE ( 'NONE',  #11085 ) ;
#1226=CIRCLE ( 'NONE', #9067, 60.74260934110282051 ) ;
#1227=ADVANCED_FACE ( 'NONE', ( #11615 ), #14692, .F. ) ;
#1233=LINE ( 'NONE', #18432, #11402 ) ;
#1237=CARTESIAN_POINT ( 'NONE',  ( -23.22718332831480481, -56.12853591711337486, 293.5832628385307999 ) ) ;
#1238=VERTEX_POINT ( 'NONE', #14592 ) ;
#1239=ORIENTED_EDGE ( 'NONE', *, *, #8863, .T. ) ;
#1241=ADVANCED_FACE ( 'NONE', ( #13235 ), #3941, .F. ) ;
#1243=EDGE_CURVE ( 'NONE', #1901, #16780, #3744, .T. ) ;
#1245=ORIENTED_EDGE ( 'NONE', *, *, #7902, .F. ) ;
#1246=ADVANCED_FACE ( 'NONE', ( #16335 ), #2419, .F. ) ;
#1248=FACE_BOUND ( 'NONE', #5298, .T. ) ;
#1251=DIRECTION ( 'NONE',  ( -0.7660444431189707970, -0.6427876096865481337, 0.000000000000000000 ) ) ;
#1252=PLANE ( 'NONE',  #7327 ) ;
#1259=EDGE_CURVE ( 'NONE', #7835, #16054, #5293, .T. ) ;
#1267=ORIENTED_EDGE ( 'NONE', *, *, #13772, .F. ) ;
#1268=AXIS2_PLACEMENT_3D ( 'NONE', #8457, #16834, #9263 ) ;
#1269=CARTESIAN_POINT ( 'NONE',  ( 5.281164089014827923, 2.240720816136096083, 293.5832628385307999 ) ) ;
#1272=EDGE_CURVE ( 'NONE', #19563, #3694, #14883, .T. ) ;
#1273=EDGE_CURVE ( 'NONE', #14920, #11567, #3842, .T. ) ;
#1274=VERTEX_POINT ( 'NONE', #7120 ) ;
#1276=EDGE_CURVE ( 'NONE', #9351, #9578, #12949, .T. ) ;
#1280=AXIS2_PLACEMENT_3D ( 'NONE', #7644, #4795, #12243 ) ;
#1281=CARTESIAN_POINT ( 'NONE',  ( 59.51724408343574879, -12.14957802882732452, 293.5832628385307999 ) ) ;
#1282=CARTESIAN_POINT ( 'NONE',  ( 53.78543575132128751, 32.64570716507559922, 248.9926560891072143 ) ) ;
#1283=ORIENTED_EDGE ( 'NONE', *, *, #13160, .T. ) ;
#1285=PLANE ( 'NONE',  #17322 ) ;
#1287=DIRECTION ( 'NONE',  ( 1.000000000000000000, 0.000000000000000000, 0.000000000000000000 ) ) ;
#1288=LINE ( 'NONE', #13756, #1176 ) ;
#1292=CARTESIAN_POINT ( 'NONE',  ( 9.381844291199747943, -57.94128254008187184, 132.4711112102474146 ) ) ;
#1293=DIRECTION ( 'NONE',  ( 0.6427876096865404731, -0.7660444431189771253, 0.000000000000000000 ) ) ;
#1295=VECTOR ( 'NONE', #19771, 1000.000000000000114 ) ;
#1297=EDGE_LOOP ( 'NONE', ( #8065, #1927, #6457, #944 ) ) ;
#1298=CARTESIAN_POINT ( 'NONE',  ( 0.000000000000000000, 0.000000000000000000, 283.5832628385307999 ) ) ;
#1302=VERTEX_POINT ( 'NONE', #11799 ) ;
#1303=VERTEX_POINT ( 'NONE', #18065 ) ;
#1309=AXIS2_PLACEMENT_3D ( 'NONE', #17020, #1571, #5973 ) ;
#1310=FACE_OUTER_BOUND ( 'NONE', #18191, .T. ) ;
#1312=ORIENTED_EDGE ( 'NONE', *, *, #4808, .T. ) ;
#1314=FACE_OUTER_BOUND ( 'NONE', #4391, .T. ) ;
#1315=DIRECTION ( 'NONE',  ( 0.6427876096865353661, 0.7660444431189813441, 0.000000000000000000 ) ) ;
#1318=LINE ( 'NONE', #12252, #18375 ) ;
#1320=VECTOR ( 'NONE', #18741, 1000.000000000000000 ) ;
#1322=DIRECTION ( 'NONE',  ( -0.6692498792541753394, -0.7430374143461900838, 0.000000000000000000 ) ) ;
#1325=ORIENTED_EDGE ( 'NONE', *, *, #10747, .T. ) ;
#1330=LINE ( 'NONE', #18727, #3389 ) ;
#1333=CARTESIAN_POINT ( 'NONE',  ( -51.23821591265114961, -28.63313560863453944, 248.9926560891072143 ) ) ;
#1337=CARTESIAN_POINT ( 'NONE',  ( -61.70726652483826058, -12.28122767885825084, 132.4711112102474146 ) ) ;
#1341=DIRECTION ( 'NONE',  ( 0.6427876096865458022, -0.7660444431189726844, 0.000000000000000000 ) ) ;
#1342=CARTESIAN_POINT ( 'NONE',  ( -5.485913980968087245, 1.678175111358129801, 283.5832628385307999 ) ) ;
#1344=ORIENTED_EDGE ( 'NONE', *, *, #17094, .T. ) ;
#1346=CARTESIAN_POINT ( 'NONE',  ( -12.14957802882752524, -59.51724408343569905, 293.5832628385307999 ) ) ;
#1347=DIRECTION ( 'NONE',  ( -0.000000000000000000, -0.000000000000000000, 1.000000000000000000 ) ) ;
#1348=ORIENTED_EDGE ( 'NONE', *, *, #401, .F. ) ;
#1350=ORIENTED_EDGE ( 'NONE', *, *, #2790, .T. ) ;
#1352=AXIS2_PLACEMENT_3D ( 'NONE', #11177, #3211, #9451 ) ;
#1354=EDGE_CURVE ( 'NONE', #8307, #6254, #12104, .T. ) ;
#1355=FACE_BOUND ( 'NONE', #9430, .T. ) ;
#1356=VERTEX_POINT ( 'NONE', #12005 ) ;
#1357=CARTESIAN_POINT ( 'NONE',  ( 0.000000000000000000, 0.000000000000000000, 4.999999999999948486 ) ) ;
#1359=CARTESIAN_POINT ( 'NONE',  ( 0.000000000000000000, 0.000000000000000000, 283.5832628385307999 ) ) ;
#1360=LINE ( 'NONE', #4427, #16225 ) ;
#1362=ORIENTED_EDGE ( 'NONE', *, *, #17062, .T. ) ;
#1365=EDGE_CURVE ( 'NONE', #11921, #6772, #2714, .T. ) ;
#1370=ORIENTED_EDGE ( 'NONE', *, *, #10229, .T. ) ;
#1372=FACE_OUTER_BOUND ( 'NONE', #9523, .T. ) ;
#1373=CIRCLE ( 'NONE', #19355, 60.74260934110282051 ) ;
#1374=VERTEX_POINT ( 'NONE', #5994 ) ;
#1375=VERTEX_POINT ( 'NONE', #4555 ) ;
#1379=CIRCLE ( 'NONE', #3344, 79.75827554147308263 ) ;
#1383=CARTESIAN_POINT ( 'NONE',  ( -0.2993243175131910516, 5.729042578294293975, 283.5832628385307999 ) ) ;
#1389=EDGE_CURVE ( 'NONE', #19700, #2129, #4445, .T. ) ;
#1392=CARTESIAN_POINT ( 'NONE',  ( 41.02350267428969488, 44.79940644582669051, 293.5832628385307999 ) ) ;
#1393=EDGE_CURVE ( 'NONE', #12098, #7664, #16631, .T. ) ;
#1396=ORIENTED_EDGE ( 'NONE', *, *, #13762, .T. ) ;
#1397=EDGE_LOOP ( 'NONE', ( #6065, #18802, #5539, #5111 ) ) ;
#1403=DIRECTION ( 'NONE',  ( -0.000000000000000000, -0.000000000000000000, 1.000000000000000000 ) ) ;
#1404=ADVANCED_FACE ( 'NONE', ( #16931 ), #2617, .F. ) ;
#1405=ORIENTED_EDGE ( 'NONE', *, *, #14893, .F. ) ;
#1406=CARTESIAN_POINT ( 'NONE',  ( 67.08601213326539892, 40.32479851956840378, 248.9926560891072143 ) ) ;
#1408=CARTESIAN_POINT ( 'NONE',  ( -0.4239815141812765531, 0.2650276884262135479, 283.5832628385307999 ) ) ;
#1409=CARTESIAN_POINT ( 'NONE',  ( -39.84224160888947353, -67.36461649554524911, 132.4711112102474146 ) ) ;
#1410=CARTESIAN_POINT ( 'NONE',  ( 0.000000000000000000, 0.000000000000000000, 283.5832628385307999 ) ) ;
#1412=LINE ( 'NONE', #12242, #6082 ) ;
#1413=FACE_OUTER_BOUND ( 'NONE', #530, .T. ) ;
#1414=VERTEX_POINT ( 'NONE', #10470 ) ;
#1416=CARTESIAN_POINT ( 'NONE',  ( -12.14957802882752524, -59.51724408343569905, 293.5832628385307999 ) ) ;
#1417=CARTESIAN_POINT ( 'NONE',  ( 0.000000000000000000, 0.000000000000000000, 132.4711112102474146 ) ) ;
#1419=VECTOR ( 'NONE', #19266, 999.9999999999998863 ) ;
#1420=EDGE_CURVE ( 'NONE', #1786, #11921, #13852, .T. ) ;
#1421=LINE ( 'NONE', #4278, #2460 ) ;
#1422=CARTESIAN_POINT ( 'NONE',  ( 67.36461649554532016, -39.84224160888924615, 248.9926560891072143 ) ) ;
#1426=EDGE_CURVE ( 'NONE', #4586, #15527, #20094, .T. ) ;
#1429=DIRECTION ( 'NONE',  ( 1.000000000000000000, 0.000000000000000000, 0.000000000000000000 ) ) ;
#1430=ORIENTED_EDGE ( 'NONE', *, *, #6776, .F. ) ;
#1432=LINE ( 'NONE', #7662, #6172 ) ;
#1434=LINE ( 'NONE', #7665, #9081 ) ;
#1435=DIRECTION ( 'NONE',  ( 0.000000000000000000, 0.000000000000000000, 1.000000000000000000 ) ) ;
#1436=ORIENTED_EDGE ( 'NONE', *, *, #6559, .F. ) ;
#1439=FACE_OUTER_BOUND ( 'NONE', #17566, .T. ) ;
#1442=CARTESIAN_POINT ( 'NONE',  ( 11.73417718768049056, 61.81362617575106810, 248.9926560891072143 ) ) ;
#1443=ORIENTED_EDGE ( 'NONE', *, *, #1629, .F. ) ;
#1444=FACE_OUTER_BOUND ( 'NONE', #9113, .T. ) ;
#1446=CARTESIAN_POINT ( 'NONE',  ( 12.78021302872850562, -77.21438937758507848, 248.9926560891072143 ) ) ;
#1448=ORIENTED_EDGE ( 'NONE', *, *, #3247, .F. ) ;
#1449=LINE ( 'NONE', #5852, #9070 ) ;
#1451=VERTEX_POINT ( 'NONE', #1166 ) ;
#1452=AXIS2_PLACEMENT_3D ( 'NONE', #11252, #11149, #5031 ) ;
#1453=ORIENTED_EDGE ( 'NONE', *, *, #13485, .F. ) ;
#1455=VECTOR ( 'NONE', #8627, 1000.000000000000000 ) ;
#1456=ORIENTED_EDGE ( 'NONE', *, *, #12727, .T. ) ;
#1458=CARTESIAN_POINT ( 'NONE',  ( 31.77187437101505907, 51.77076963420835654, 283.5832628385307999 ) ) ;
#1459=ORIENTED_EDGE ( 'NONE', *, *, #17351, .F. ) ;
#1460=CARTESIAN_POINT ( 'NONE',  ( 12.14914984460760827, 59.51523122377248853, 283.5832628385307999 ) ) ;
#1463=VECTOR ( 'NONE', #9695, 1000.000000000000000 ) ;
#1465=CARTESIAN_POINT ( 'NONE',  ( 0.000000000000000000, 0.000000000000000000, 293.5832628385307999 ) ) ;
#1466=DIRECTION ( 'NONE',  ( -0.000000000000000000, -0.000000000000000000, 1.000000000000000000 ) ) ;
#1469=CARTESIAN_POINT ( 'NONE',  ( -2.629250726500700353, -60.68567895461850981, 283.5832628385307999 ) ) ;
#1470=CARTESIAN_POINT ( 'NONE',  ( 4.196299268919053915, 3.911853314815666671, 293.5832628385307999 ) ) ;
#1473=ORIENTED_EDGE ( 'NONE', *, *, #16771, .T. ) ;
#1474=PRODUCT ( 'MOTOR', 'MOTOR', '', ( #6680 ) ) ;
#1475=LINE ( 'NONE', #18773, #12818 ) ;
#1477=VERTEX_POINT ( 'NONE', #16724 ) ;
#1478=VECTOR ( 'NONE', #14562, 1000.000000000000000 ) ;
#1479=VERTEX_POINT ( 'NONE', #967 ) ;
#1481=ORIENTED_EDGE ( 'NONE', *, *, #16634, .T. ) ;
#1482=EDGE_CURVE ( 'NONE', #15468, #2215, #15287, .T. ) ;
#1485=DIRECTION ( 'NONE',  ( 0.1736481776669241694, 0.9848077530122092416, -0.000000000000000000 ) ) ;
#1486=LINE ( 'NONE', #10885, #16280 ) ;
#1487=VERTEX_POINT ( 'NONE', #17141 ) ;
#1488=VECTOR ( 'NONE', #19524, 1000.000000000000000 ) ;
#1490=CARTESIAN_POINT ( 'NONE',  ( 8.939227532413712041, -60.08331549348429235, 283.5832628385307999 ) ) ;
#1491=ORIENTED_EDGE ( 'NONE', *, *, #4117, .F. ) ;
#1493=CARTESIAN_POINT ( 'NONE',  ( -58.69016442926522359, 0.8220851292433277724, 132.4711112102474146 ) ) ;
#1496=CARTESIAN_POINT ( 'NONE',  ( 18.28567271940513450, -57.92709869106715814, 283.5832628385307999 ) ) ;
#1497=ADVANCED_FACE ( 'NONE', ( #11088 ), #6603, .T. ) ;
#1499=DIRECTION ( 'NONE',  ( 0.7660444431189771253, 0.6427876096865404731, 0.000000000000000000 ) ) ;
#1503=ORIENTED_EDGE ( 'NONE', *, *, #5665, .F. ) ;
#1505=CARTESIAN_POINT ( 'NONE',  ( 5.729042578294149202, 0.2993243175132214717, 283.5832628385307999 ) ) ;
#1507=DIRECTION ( 'NONE',  ( -0.9781142164131910732, 0.2080686897406944236, 0.000000000000000000 ) ) ;
#1508=EDGE_CURVE ( 'NONE', #13730, #17780, #4871, .T. ) ;
#1510=DIRECTION ( 'NONE',  ( 0.000000000000000000, 0.000000000000000000, 1.000000000000000000 ) ) ;
#1513=LINE ( 'NONE', #10810, #17528 ) ;
#1516=ORIENTED_EDGE ( 'NONE', *, *, #8040, .T. ) ;
#1518=PRODUCT_DEFINITION_CONTEXT ( 'detailed design', #14040, 'design' ) ;
#1520=FACE_OUTER_BOUND ( 'NONE', #4411, .T. ) ;
#1521=CARTESIAN_POINT ( 'NONE',  ( 4.581103194070519358, -3.453261854573403067, 293.5832628385307999 ) ) ;
#1522=VECTOR ( 'NONE', #10585, 1000.000000000000000 ) ;
#1523=EDGE_CURVE ( 'NONE', #3549, #1972, #14271, .T. ) ;
#1526=ORIENTED_EDGE ( 'NONE', *, *, #1659, .T. ) ;
#1527=CARTESIAN_POINT ( 'NONE',  ( 0.000000000000000000, 0.000000000000000000, 132.4711112102474146 ) ) ;
#1528=ORIENTED_EDGE ( 'NONE', *, *, #8607, .T. ) ;
#1530=ORIENTED_EDGE ( 'NONE', *, *, #4656, .F. ) ;
#1531=CARTESIAN_POINT ( 'NONE',  ( -22.81000261549328911, 58.63718168490508020, 132.4711112102474146 ) ) ;
#1535=EDGE_CURVE ( 'NONE', #11442, #8543, #15600, .T. ) ;
#1537=VECTOR ( 'NONE', #15562, 1000.000000000000114 ) ;
#1538=CARTESIAN_POINT ( 'NONE',  ( 37.09555676056997697, -45.48770046196272432, 110.7293897666001214 ) ) ;
#1541=LINE ( 'NONE', #7974, #8014 ) ;
#1546=ORIENTED_EDGE ( 'NONE', *, *, #2756, .F. ) ;
#1547=FACE_OUTER_BOUND ( 'NONE', #3646, .T. ) ;
#1548=DIRECTION ( 'NONE',  ( 1.000000000000000000, 0.000000000000000000, 0.000000000000000000 ) ) ;
#1549=FACE_OUTER_BOUND ( 'NONE', #20139, .T. ) ;
#1551=VERTEX_POINT ( 'NONE', #1792 ) ;
#1554=DIRECTION ( 'NONE',  ( -0.3747554100459959403, -0.9271237148521535021, 0.000000000000000000 ) ) ;
#1555=EDGE_LOOP ( 'NONE', ( #4358, #10280, #171, #524 ) ) ;
#1556=ORIENTED_EDGE ( 'NONE', *, *, #10730, .F. ) ;
#1557=ORIENTED_EDGE ( 'NONE', *, *, #18119, .T. ) ;
#1559=ORIENTED_EDGE ( 'NONE', *, *, #10321, .T. ) ;
#1560=CARTESIAN_POINT ( 'NONE',  ( -32.62092819947992695, -51.24245927909985454, 293.5832628385307999 ) ) ;
#1563=PLANE ( 'NONE',  #16759 ) ;
#1565=DIRECTION ( 'NONE',  ( 0.03505990758545895342, 0.9993852124581886764, 0.000000000000000000 ) ) ;
#1566=VECTOR ( 'NONE', #7488, 1000.000000000000000 ) ;
#1567=AXIS2_PLACEMENT_3D ( 'NONE', #1346, #18647, #7680 ) ;
#1569=CARTESIAN_POINT ( 'NONE',  ( 12.28122767885846223, -61.70726652483821084, 132.4711112102474146 ) ) ;
#1571=DIRECTION ( 'NONE',  ( -0.000000000000000000, -0.000000000000000000, 1.000000000000000000 ) ) ;
#1574=LINE ( 'NONE', #9031, #2977 ) ;
#1575=CARTESIAN_POINT ( 'NONE',  ( 30.05702882063027914, 50.41613078340812848, 110.9660488491356887 ) ) ;
#1580=ORIENTED_EDGE ( 'NONE', *, *, #1259, .F. ) ;
#1585=DIRECTION ( 'NONE',  ( 0.3420201433256694901, -0.9396926207859082059, 0.000000000000000000 ) ) ;
#1586=DIRECTION ( 'NONE',  ( -0.9848077530122066880, -0.1736481776669374644, 0.000000000000000000 ) ) ;
#1587=ORIENTED_EDGE ( 'NONE', *, *, #12086, .F. ) ;
#1588=VECTOR ( 'NONE', #17796, 1000.000000000000000 ) ;
#1591=AXIS2_PLACEMENT_3D ( 'NONE', #18205, #10727, #2968 ) ;
#1592=AXIS2_PLACEMENT_3D ( 'NONE', #14625, #6663, #9920 ) ;
#1595=AXIS2_PLACEMENT_3D ( 'NONE', #2928, #14068, #6309 ) ;
#1596=PLANE ( 'NONE',  #15083 ) ;
#1599=DIRECTION ( 'NONE',  ( 0.3088643371590125142, -0.9511061040868803440, 0.000000000000000000 ) ) ;
#1601=EDGE_CURVE ( 'NONE', #18954, #8910, #6203, .T. ) ;
#1602=DIRECTION ( 'NONE',  ( 0.6427876096865430267, -0.7660444431189749048, 0.000000000000000000 ) ) ;
#1605=ADVANCED_FACE ( 'NONE', ( #9257 ), #52, .T. ) ;
#1606=ORIENTED_EDGE ( 'NONE', *, *, #16687, .F. ) ;
#1607=ORIENTED_EDGE ( 'NONE', *, *, #17136, .F. ) ;
#1608=VECTOR ( 'NONE', #12347, 1000.000000000000000 ) ;
#1609=CIRCLE ( 'NONE', #9455, 60.74260934110282051 ) ;
#1615=EDGE_CURVE ( 'NONE', #7758, #11142, #3427, .T. ) ;
#1618=DIRECTION ( 'NONE',  ( -0.8660254037844363761, -0.5000000000000039968, 0.000000000000000000 ) ) ;
#1619=DIRECTION ( 'NONE',  ( -0.000000000000000000, -0.000000000000000000, 1.000000000000000000 ) ) ;
#1620=ORIENTED_EDGE ( 'NONE', *, *, #8861, .F. ) ;
#1621=CARTESIAN_POINT ( 'NONE',  ( 53.40063514825076396, 28.94886449118923721, 283.5832628385307999 ) ) ;
#1623=ORIENTED_EDGE ( 'NONE', *, *, #5733, .T. ) ;
#1625=DIRECTION ( 'NONE',  ( -0.8830229359480271656, -0.4693298356057563625, 0.000000000000000000 ) ) ;
#1629=EDGE_CURVE ( 'NONE', #19246, #9958, #15910, .T. ) ;
#1631=ADVANCED_FACE ( 'NONE', ( #12521 ), #18783, .F. ) ;
#1634=VERTEX_POINT ( 'NONE', #10986 ) ;
#1635=ADVANCED_FACE ( 'NONE', ( #17245 ), #13312, .F. ) ;
#1636=DIRECTION ( 'NONE',  ( -0.1736481776669206722, -0.9848077530122096857, 0.000000000000000000 ) ) ;
#1637=EDGE_LOOP ( 'NONE', ( #6576, #3214, #91, #19853 ) ) ;
#1638=ORIENTED_EDGE ( 'NONE', *, *, #989, .T. ) ;
#1639=CARTESIAN_POINT ( 'NONE',  ( 0.000000000000000000, 0.000000000000000000, 248.9926560891072143 ) ) ;
#1646=DIRECTION ( 'NONE',  ( 1.000000000000000000, 0.000000000000000000, 0.000000000000000000 ) ) ;
#1649=ORIENTED_EDGE ( 'NONE', *, *, #15735, .T. ) ;
#1650=DIRECTION ( 'NONE',  ( 0.000000000000000000, 0.000000000000000000, -1.000000000000000000 ) ) ;
#1652=CARTESIAN_POINT ( 'NONE',  ( 0.000000000000000000, 0.000000000000000000, 293.5832628385307999 ) ) ;
#1653=EDGE_CURVE ( 'NONE', #9691, #10395, #16414, .T. ) ;
#1658=EDGE_CURVE ( 'NONE', #13976, #15168, #5364, .T. ) ;
#1659=EDGE_CURVE ( 'NONE', #7429, #1375, #8429, .T. ) ;
#1660=CARTESIAN_POINT ( 'NONE',  ( 56.50329132715945235, -22.30005961346246579, 293.5832628385307999 ) ) ;
#1662=ORIENTED_EDGE ( 'NONE', *, *, #11670, .T. ) ;
#1663=ORIENTED_EDGE ( 'NONE', *, *, #7409, .T. ) ;
#1665=EDGE_LOOP ( 'NONE', ( #14610, #8264, #5272, #7279 ) ) ;
#1667=FACE_BOUND ( 'NONE', #10726, .T. ) ;
#1669=VECTOR ( 'NONE', #12429, 1000.000000000000000 ) ;
#1677=EDGE_CURVE ( 'NONE', #17774, #1634, #12213, .T. ) ;
#1679=DIRECTION ( 'NONE',  ( 1.000000000000000000, 0.000000000000000000, 0.000000000000000000 ) ) ;
#1684=VECTOR ( 'NONE', #15696, 1000.000000000000000 ) ;
#1685=EDGE_CURVE ( 'NONE', #16315, #16184, #6704, .T. ) ;
#1689=CARTESIAN_POINT ( 'NONE',  ( 26.04958516073451236, 47.87779272208936021, 248.9926560891072143 ) ) ;
#1692=ORIENTED_EDGE ( 'NONE', *, *, #9501, .T. ) ;
#1693=DIRECTION ( 'NONE',  ( 1.000000000000000000, 0.000000000000000000, 0.000000000000000000 ) ) ;
#1701=EDGE_LOOP ( 'NONE', ( #3307, #2684, #15104 ) ) ;
#1703=EDGE_LOOP ( 'NONE', ( #9563, #5259, #2824, #1057 ) ) ;
#1705=CARTESIAN_POINT ( 'NONE',  ( -23.22718332831480481, -56.12853591711337486, 293.5832628385307999 ) ) ;
#1706=VECTOR ( 'NONE', #463, 1000.000000000000000 ) ;
#1709=DIRECTION ( 'NONE',  ( -0.7660444431189835646, 0.6427876096865328126, 0.000000000000000000 ) ) ;
#1710=DIRECTION ( 'NONE',  ( -0.5300553768524376430, -0.8479630283625698706, 0.000000000000000000 ) ) ;
#1712=ORIENTED_EDGE ( 'NONE', *, *, #11528, .F. ) ;
#1713=CARTESIAN_POINT ( 'NONE',  ( -55.16472960512350454, 30.25670013172272732, 248.9926560891072143 ) ) ;
#1714=LINE ( 'NONE', #18815, #19892 ) ;
#1717=LINE ( 'NONE', #20130, #18249 ) ;
#1718=DIRECTION ( 'NONE',  ( 1.000000000000000000, 0.000000000000000000, 0.000000000000000000 ) ) ;
#1719=VECTOR ( 'NONE', #11438, 999.9999999999998863 ) ;
#1720=DIRECTION ( 'NONE',  ( -0.000000000000000000, -0.000000000000000000, 1.000000000000000000 ) ) ;
#1723=ORIENTED_EDGE ( 'NONE', *, *, #1272, .F. ) ;
#1724=EDGE_CURVE ( 'NONE', #13875, #15125, #846, .T. ) ;
#1725=PLANE ( 'NONE',  #116 ) ;
#1726=ORIENTED_EDGE ( 'NONE', *, *, #13356, .F. ) ;
#1729=DIRECTION ( 'NONE',  ( -0.000000000000000000, -0.000000000000000000, 1.000000000000000000 ) ) ;
#1731=CYLINDRICAL_SURFACE ( 'NONE', #17927, 62.91752772691707207 ) ;
#1732=EDGE_CURVE ( 'NONE', #17702, #7714, #16013, .T. ) ;
#1734=CIRCLE ( 'NONE', #18728, 60.74260934110282051 ) ;
#1737=ADVANCED_FACE ( 'NONE', ( #3921 ), #14862, .T. ) ;
#1739=CARTESIAN_POINT ( 'NONE',  ( 0.000000000000000000, 0.000000000000000000, 293.5832628385307999 ) ) ;
#1742=AXIS2_PLACEMENT_3D ( 'NONE', #15415, #10698, #16954 ) ;
#1744=LINE ( 'NONE', #17711, #4727 ) ;
#1746=DIRECTION ( 'NONE',  ( 1.000000000000000000, 0.000000000000000000, 0.000000000000000000 ) ) ;
#1747=AXIS2_PLACEMENT_3D ( 'NONE', #1538, #15551, #12055 ) ;
#1749=CARTESIAN_POINT ( 'NONE',  ( -56.12662799072088404, 23.22641211976270625, 283.5832628385307999 ) ) ;
#1751=ORIENTED_EDGE ( 'NONE', *, *, #989, .F. ) ;
#1753=DIRECTION ( 'NONE',  ( -0.000000000000000000, -0.000000000000000000, 1.000000000000000000 ) ) ;
#1755=VECTOR ( 'NONE', #18931, 1000.000000000000000 ) ;
#1757=ORIENTED_EDGE ( 'NONE', *, *, #7286, .F. ) ;
#1758=ORIENTED_EDGE ( 'NONE', *, *, #4080, .F. ) ;
#1759=VECTOR ( 'NONE', #16906, 1000.000000000000000 ) ;
#1764=ORIENTED_EDGE ( 'NONE', *, *, #10036, .F. ) ;
#1766=LINE ( 'NONE', #6282, #14801 ) ;
#1767=LINE ( 'NONE', #18967, #10903 ) ;
#1769=EDGE_CURVE ( 'NONE', #7001, #4216, #2900, .T. ) ;
#1772=LINE ( 'NONE', #17336, #18832 ) ;
#1773=CARTESIAN_POINT ( 'NONE',  ( 25.99419088092191643, -73.82206860051539365, 132.4711112102474146 ) ) ;
#1775=PLANE ( 'NONE',  #19420 ) ;
#1776=CARTESIAN_POINT ( 'NONE',  ( 36.99514631729018532, -48.17959877923561862, 293.5832628385307999 ) ) ;
#1779=LINE ( 'NONE', #3514, #8208 ) ;
#1781=ORIENTED_EDGE ( 'NONE', *, *, #844, .F. ) ;
#1783=LINE ( 'NONE', #17548, #15777 ) ;
#1785=EDGE_LOOP ( 'NONE', ( #14903, #9584 ) ) ;
#1786=VERTEX_POINT ( 'NONE', #9126 ) ;
#1787=VERTEX_POINT ( 'NONE', #2594 ) ;
#1789=EDGE_CURVE ( 'NONE', #2612, #7835, #16170, .T. ) ;
#1790=VECTOR ( 'NONE', #8875, 1000.000000000000114 ) ;
#1791=ADVANCED_FACE ( 'NONE', ( #5662 ), #9021, .F. ) ;
#1792=CARTESIAN_POINT ( 'NONE',  ( 32.64570716507540737, -53.78543575132140830, 132.4711112102474146 ) ) ;
#1793=DIRECTION ( 'NONE',  ( -0.1736481776669207000, -0.9848077530122097967, 0.000000000000000000 ) ) ;
#1794=DIRECTION ( 'NONE',  ( 0.9848077530122091305, -0.1736481776669241417, 0.000000000000000000 ) ) ;
#1800=VECTOR ( 'NONE', #17404, 1000.000000000000114 ) ;
#1802=ORIENTED_EDGE ( 'NONE', *, *, #17084, .T. ) ;
#1804=CIRCLE ( 'NONE', #13210, 60.74260934110282051 ) ;
#1808=ORIENTED_EDGE ( 'NONE', *, *, #7146, .T. ) ;
#1812=ORIENTED_EDGE ( 'NONE', *, *, #15557, .T. ) ;
#1813=LINE ( 'NONE', #4685, #1854 ) ;
#1815=DIRECTION ( 'NONE',  ( -0.5300553768524346454, -0.8479630283625717579, 0.000000000000000000 ) ) ;
#1819=DIRECTION ( 'NONE',  ( -0.5000000000000009992, 0.8660254037844380415, 0.000000000000000000 ) ) ;
#1821=DIRECTION ( 'NONE',  ( 0.000000000000000000, 0.000000000000000000, -1.000000000000000000 ) ) ;
#1825=FACE_OUTER_BOUND ( 'NONE', #5481, .T. ) ;
#1826=FACE_OUTER_BOUND ( 'NONE', #7645, .T. ) ;
#1831=CARTESIAN_POINT ( 'NONE',  ( 49.67518383744835120, -60.47951622432767493, 110.7293897666001214 ) ) ;
#1832=ORIENTED_EDGE ( 'NONE', *, *, #3155, .F. ) ;
#1833=ORIENTED_EDGE ( 'NONE', *, *, #8359, .T. ) ;
#1834=LINE ( 'NONE', #17082, #18907 ) ;
#1835=ORIENTED_EDGE ( 'NONE', *, *, #6218, .T. ) ;
#1836=AXIS2_PLACEMENT_3D ( 'NONE', #1169, #4245, #7414 ) ;
#1837=DIRECTION ( 'NONE',  ( -0.7660444431189835646, 0.6427876096865328126, 0.000000000000000000 ) ) ;
#1838=CARTESIAN_POINT ( 'NONE',  ( 37.93579148621461883, 68.46530598706809201, 132.4711112102474146 ) ) ;
#1841=CARTESIAN_POINT ( 'NONE',  ( -9.381844291199351815, 57.94128254008192158, 112.0427633081291816 ) ) ;
#1842=ADVANCED_FACE ( 'NONE', ( #5765 ), #1252, .T. ) ;
#1844=AXIS2_PLACEMENT_3D ( 'NONE', #15301, #1293, #1499 ) ;
#1845=CARTESIAN_POINT ( 'NONE',  ( 0.8220851292435327196, 62.91215678473957240, 248.9926560891072143 ) ) ;
#1848=FACE_OUTER_BOUND ( 'NONE', #17236, .T. ) ;
#1849=CARTESIAN_POINT ( 'NONE',  ( 0.000000000000000000, 0.000000000000000000, 83.57543755549745867 ) ) ;
#1853=ORIENTED_EDGE ( 'NONE', *, *, #2497, .F. ) ;
#1854=VECTOR ( 'NONE', #18702, 1000.000000000000114 ) ;
#1855=EDGE_CURVE ( 'NONE', #858, #9602, #7389, .T. ) ;
#1860=EDGE_CURVE ( 'NONE', #11048, #19503, #12189, .T. ) ;
#1861=AXIS2_PLACEMENT_3D ( 'NONE', #16348, #17885, #10103 ) ;
#1864=LINE ( 'NONE', #325, #3263 ) ;
#1865=CARTESIAN_POINT ( 'NONE',  ( 0.000000000000000000, 0.000000000000000000, 293.5832628385307999 ) ) ;
#1866=VERTEX_POINT ( 'NONE', #8919 ) ;
#1870=EDGE_CURVE ( 'NONE', #8891, #15066, #11880, .T. ) ;
#1872=FACE_OUTER_BOUND ( 'NONE', #3737, .T. ) ;
#1875=DIRECTION ( 'NONE',  ( 1.000000000000000000, 0.000000000000000000, 0.000000000000000000 ) ) ;
#1876=DIRECTION ( 'NONE',  ( 1.000000000000000000, 0.000000000000000000, 0.000000000000000000 ) ) ;
#1879=ORIENTED_EDGE ( 'NONE', *, *, #168, .T. ) ;
#1880=EDGE_CURVE ( 'NONE', #10402, #19514, #946, .T. ) ;
#1882=ADVANCED_FACE ( 'NONE', ( #5866 ), #7198, .F. ) ;
#1883=EDGE_CURVE ( 'NONE', #17498, #9484, #13516, .T. ) ;
#1884=ORIENTED_EDGE ( 'NONE', *, *, #12889, .F. ) ;
#1886=AXIS2_PLACEMENT_3D ( 'NONE', #9686, #1923, #16038 ) ;
#1889=AXIS2_PLACEMENT_3D ( 'NONE', #8232, #4882, #12736 ) ;
#1892=CARTESIAN_POINT ( 'NONE',  ( -11.00103590902911499, -57.65577537092155325, 248.9926560891072143 ) ) ;
#1893=CARTESIAN_POINT ( 'NONE',  ( -62.91752772691707207, 8.736373289420574370E-15, 83.57543755549745867 ) ) ;
#1894=CARTESIAN_POINT ( 'NONE',  ( -14.39940464655760799, -76.92888220842476699, 132.4711112102474146 ) ) ;
#1895=EDGE_LOOP ( 'NONE', ( #421, #9874, #17551 ) ) ;
#1896=DIRECTION ( 'NONE',  ( -0.000000000000000000, -0.000000000000000000, 1.000000000000000000 ) ) ;
#1899=CARTESIAN_POINT ( 'NONE',  ( -59.30716253403183202, 13.12726406102060217, 283.5832628385307999 ) ) ;
#1901=VERTEX_POINT ( 'NONE', #18945 ) ;
#1905=EDGE_CURVE ( 'NONE', #10931, #8624, #14525, .T. ) ;
#1906=LINE ( 'NONE', #9776, #5771 ) ;
#1908=EDGE_LOOP ( 'NONE', ( #144, #18042, #3141, #15618 ) ) ;
#1909=ADVANCED_FACE ( 'NONE', ( #5227 ), #6562, .T. ) ;
#1910=ORIENTED_EDGE ( 'NONE', *, *, #6373, .F. ) ;
#1912=ORIENTED_EDGE ( 'NONE', *, *, #6675, .F. ) ;
#1913=DIRECTION ( 'NONE',  ( -0.9993852124581887875, 0.03505990758545545621, 0.000000000000000000 ) ) ;
#1916=EDGE_LOOP ( 'NONE', ( #9131, #3969, #19888, #11350 ) ) ;
#1919=AXIS2_PLACEMENT_3D ( 'NONE', #13938, #13832, #15479 ) ;
#1920=CARTESIAN_POINT ( 'NONE',  ( 51.24245927909996112, -32.62092819947974220, 293.5832628385307999 ) ) ;
#1923=DIRECTION ( 'NONE',  ( -0.1736481776669404620, 0.9848077530122062440, 0.000000000000000000 ) ) ;
#1924=VERTEX_POINT ( 'NONE', #17605 ) ;
#1927=ORIENTED_EDGE ( 'NONE', *, *, #18850, .F. ) ;
#1930=CARTESIAN_POINT ( 'NONE',  ( 0.8220851292435327196, 78.26059000578311498, 248.9926560891072143 ) ) ;
#1931=LINE ( 'NONE', #17282, #6702 ) ;
#1933=CARTESIAN_POINT ( 'NONE',  ( -2.629322876227788264, -60.68773558783006905, 293.5832628385307999 ) ) ;
#1934=CARTESIAN_POINT ( 'NONE',  ( 59.58067424803626011, -20.21777810286696564, 132.4711112102474146 ) ) ;
#1935=LINE ( 'NONE', #14410, #12622 ) ;
#1936=VECTOR ( 'NONE', #14201, 1000.000000000000000 ) ;
#1938=ORIENTED_EDGE ( 'NONE', *, *, #1997, .T. ) ;
#1939=AXIS2_PLACEMENT_3D ( 'NONE', #17249, #15813, #1693 ) ;
#1940=CARTESIAN_POINT ( 'NONE',  ( 78.26059000578312919, -0.8220851292427129309, 112.7772637782949516 ) ) ;
#1942=EDGE_CURVE ( 'NONE', #3127, #12874, #11451, .T. ) ;
#1943=VERTEX_POINT ( 'NONE', #19041 ) ;
#1947=PLANE ( 'NONE',  #2408 ) ;
#1948=ORIENTED_EDGE ( 'NONE', *, *, #15789, .F. ) ;
#1949=LINE ( 'NONE', #14425, #18148 ) ;
#1950=DIRECTION ( 'NONE',  ( -0.9902903945359624593, -0.1390141521205945918, 0.000000000000000000 ) ) ;
#1951=CIRCLE ( 'NONE', #16000, 62.91752772691707207 ) ;
#1952=AXIS2_PLACEMENT_3D ( 'NONE', #3657, #8252, #9890 ) ;
#1954=CARTESIAN_POINT ( 'NONE',  ( -54.07248341783231638, 32.16802499836798290, 132.4711112102474146 ) ) ;
#1958=DIRECTION ( 'NONE',  ( -0.9781142164131910732, 0.2080686897406944236, 0.000000000000000000 ) ) ;
#1959=CARTESIAN_POINT ( 'NONE',  ( 67.36461649554529174, -39.84224160888925326, 132.4711112102474146 ) ) ;
#1960=CARTESIAN_POINT ( 'NONE',  ( 0.000000000000000000, 0.000000000000000000, 283.5832628385307999 ) ) ;
#1961=DIRECTION ( 'NONE',  ( -0.000000000000000000, -0.000000000000000000, 1.000000000000000000 ) ) ;
#1962=EDGE_LOOP ( 'NONE', ( #15435, #18285, #9262, #7046 ) ) ;
#1965=VERTEX_POINT ( 'NONE', #6755 ) ;
#1968=EDGE_CURVE ( 'NONE', #5595, #19503, #9232, .T. ) ;
#1969=VERTEX_POINT ( 'NONE', #12679 ) ;
#1970=VERTEX_POINT ( 'NONE', #7975 ) ;
#1972=VERTEX_POINT ( 'NONE', #2153 ) ;
#1973=LINE ( 'NONE', #9940, #18862 ) ;
#1974=ORIENTED_EDGE ( 'NONE', *, *, #19282, .T. ) ;
#1977=CARTESIAN_POINT ( 'NONE',  ( 0.000000000000000000, 0.000000000000000000, 283.5832628385307999 ) ) ;
#1978=AXIS2_PLACEMENT_3D ( 'NONE', #521, #2355, #13178 ) ;
#1982=LINE ( 'NONE', #19169, #185 ) ;
#1983=CARTESIAN_POINT ( 'NONE',  ( 51.36153797460909232, -59.06449708980182578, 248.9926560891072143 ) ) ;
#1984=CARTESIAN_POINT ( 'NONE',  ( -11.54977938102048007, 57.55901709132182731, 132.4711112102474146 ) ) ;
#1985=FACE_OUTER_BOUND ( 'NONE', #19871, .T. ) ;
#1988=EDGE_LOOP ( 'NONE', ( #8084, #8409, #2017, #10586 ) ) ;
#1992=ORIENTED_EDGE ( 'NONE', *, *, #9300, .F. ) ;
#1993=VECTOR ( 'NONE', #19337, 1000.000000000000227 ) ;
#1995=ORIENTED_EDGE ( 'NONE', *, *, #2272, .F. ) ;
#1996=DIRECTION ( 'NONE',  ( 0.000000000000000000, 0.000000000000000000, -1.000000000000000000 ) ) ;
#1997=EDGE_CURVE ( 'NONE', #4838, #6246, #3584, .T. ) ;
#2001=EDGE_CURVE ( 'NONE', #10388, #19150, #8181, .T. ) ;
#2002=CARTESIAN_POINT ( 'NONE',  ( -79.75827554147308263, 9.767571684737763671E-15, 269.6944534026102360 ) ) ;
#2005=DIRECTION ( 'NONE',  ( -0.9902903945359630145, -0.1390141521205912334, 0.000000000000000000 ) ) ;
#2008=DIRECTION ( 'NONE',  ( 0.9781142164131917394, -0.2080686897406911207, 0.000000000000000000 ) ) ;
#2010=CARTESIAN_POINT ( 'NONE',  ( 60.08127757648377099, 8.938941455415205795, 283.5832628385307999 ) ) ;
#2011=VERTEX_POINT ( 'NONE', #606 ) ;
#2012=EDGE_CURVE ( 'NONE', #1477, #3588, #6661, .T. ) ;
#2013=VECTOR ( 'NONE', #3418, 1000.000000000000000 ) ;
#2016=EDGE_LOOP ( 'NONE', ( #13062, #1109, #19889, #3041 ) ) ;
#2017=ORIENTED_EDGE ( 'NONE', *, *, #9353, .T. ) ;
#2019=ORIENTED_EDGE ( 'NONE', *, *, #9001, .T. ) ;
#2020=CARTESIAN_POINT ( 'NONE',  ( 39.37628763770420903, 49.07263256785967087, 293.5832628385307999 ) ) ;
#2025=ADVANCED_FACE ( 'NONE', ( #17933 ), #16199, .F. ) ;
#2028=ADVANCED_FACE ( 'NONE', ( #16395 ), #4096, .T. ) ;
#2031=CARTESIAN_POINT ( 'NONE',  ( -53.40063514825077107, -28.94886449118923011, 293.5832628385307999 ) ) ;
#2033=DIRECTION ( 'NONE',  ( 1.000000000000000000, 0.000000000000000000, -0.000000000000000000 ) ) ;
#2039=ADVANCED_FACE ( 'NONE', ( #18524 ), #15242, .F. ) ;
#2040=DIRECTION ( 'NONE',  ( -0.000000000000000000, -0.000000000000000000, 1.000000000000000000 ) ) ;
#2041=CIRCLE ( 'NONE', #17726, 60.74260934110282051 ) ;
#2044=LINE ( 'NONE', #19612, #16763 ) ;
#2045=ORIENTED_EDGE ( 'NONE', *, *, #3986, .T. ) ;
#2048=ORIENTED_EDGE ( 'NONE', *, *, #14538, .F. ) ;
#2049=ADVANCED_FACE ( 'NONE', ( #13600 ), #19846, .F. ) ;
#2057=EDGE_CURVE ( 'NONE', #13334, #14067, #16787, .T. ) ;
#2059=CARTESIAN_POINT ( 'NONE',  ( -18.28503710798546678, 57.92514141135459482, 283.5832628385307999 ) ) ;
#2062=PLANE ( 'NONE',  #7087 ) ;
#2063=AXIS2_PLACEMENT_3D ( 'NONE', #5235, #6862, #9720 ) ;
#2065=FACE_OUTER_BOUND ( 'NONE', #633, .T. ) ;
#2067=LINE ( 'NONE', #4834, #13328 ) ;
#2070=ORIENTED_EDGE ( 'NONE', *, *, #15491, .F. ) ;
#2071=VERTEX_POINT ( 'NONE', #8804 ) ;
#2074=VECTOR ( 'NONE', #15472, 999.9999999999998863 ) ;
#2076=DIRECTION ( 'NONE',  ( -0.9902903945359624593, -0.1390141521205945918, 0.000000000000000000 ) ) ;
#2077=LINE ( 'NONE', #11065, #10031 ) ;
#2079=VECTOR ( 'NONE', #9482, 1000.000000000000000 ) ;
#2090=VERTEX_POINT ( 'NONE', #1337 ) ;
#2095=ORIENTED_EDGE ( 'NONE', *, *, #1769, .T. ) ;
#2099=CARTESIAN_POINT ( 'NONE',  ( -58.63718168490499494, -22.81000261549348807, 293.5832628385307999 ) ) ;
#2102=EDGE_CURVE ( 'NONE', #15527, #19079, #4609, .T. ) ;
#2104=CARTESIAN_POINT ( 'NONE',  ( 1.289614712049185874, -5.590028426173808462, 283.5832628385307999 ) ) ;
#2106=VECTOR ( 'NONE', #11427, 1000.000000000000114 ) ;
#2112=ADVANCED_FACE ( 'NONE', ( #1025 ), #2572, .T. ) ;
#2114=ADVANCED_FACE ( 'NONE', ( #10629 ), #7271, .T. ) ;
#2116=EDGE_LOOP ( 'NONE', ( #18057, #19985, #17004, #1580 ) ) ;
#2117=ADVANCED_FACE ( 'NONE', ( #1125 ), #12060, .F. ) ;
#2118=DIRECTION ( 'NONE',  ( 0.000000000000000000, 1.000000000000000000, 0.000000000000000000 ) ) ;
#2119=AXIS2_PLACEMENT_3D ( 'NONE', #18139, #19667, #10551 ) ;
#2120=ORIENTED_EDGE ( 'NONE', *, *, #18776, .F. ) ;
#2121=FACE_OUTER_BOUND ( 'NONE', #16081, .T. ) ;
#2122=CYLINDRICAL_SURFACE ( 'NONE', #8302, 60.74260934110282051 ) ;
#2123=CARTESIAN_POINT ( 'NONE',  ( 0.000000000000000000, 0.000000000000000000, 269.6944534026102360 ) ) ;
#2124=EDGE_LOOP ( 'NONE', ( #8641, #17677, #10547, #9555 ) ) ;
#2128=EDGE_CURVE ( 'NONE', #18905, #12093, #8842, .T. ) ;
#2129=VERTEX_POINT ( 'NONE', #6933 ) ;
#2132=AXIS2_PLACEMENT_3D ( 'NONE', #2703, #10267, #8358 ) ;
#2134=CARTESIAN_POINT ( 'NONE',  ( 47.56406379474552182, 37.78325588002191893, 283.5832628385307999 ) ) ;
#2141=ORIENTED_EDGE ( 'NONE', *, *, #4483, .F. ) ;
#2142=EDGE_CURVE ( 'NONE', #18256, #16743, #5301, .T. ) ;
#2144=ORIENTED_EDGE ( 'NONE', *, *, #8858, .F. ) ;
#2145=EDGE_CURVE ( 'NONE', #6039, #10395, #7534, .T. ) ;
#2148=ORIENTED_EDGE ( 'NONE', *, *, #2258, .F. ) ;
#2149=CARTESIAN_POINT ( 'NONE',  ( 44.43084819159276577, -38.35506425062471436, 110.7293897666001214 ) ) ;
#2153=CARTESIAN_POINT ( 'NONE',  ( 37.93579148621461172, 68.46530598706807780, 248.9926560891072143 ) ) ;
#2154=EDGE_CURVE ( 'NONE', #18469, #16270, #19417, .T. ) ;
#2160=LINE ( 'NONE', #14628, #17800 ) ;
#2162=DIRECTION ( 'NONE',  ( -0.8479630283625716469, 0.5300553768524345344, 0.000000000000000000 ) ) ;
#2166=ORIENTED_EDGE ( 'NONE', *, *, #2145, .F. ) ;
#2176=EDGE_LOOP ( 'NONE', ( #12386, #890, #5115, #11167 ) ) ;
#2178=VECTOR ( 'NONE', #8074, 1000.000000000000000 ) ;
#2180=ORIENTED_EDGE ( 'NONE', *, *, #5365, .T. ) ;
#2182=DIRECTION ( 'NONE',  ( -0.6427876096865430267, 0.7660444431189749048, 0.000000000000000000 ) ) ;
#2187=VECTOR ( 'NONE', #15931, 1000.000000000000000 ) ;
#2189=LINE ( 'NONE', #5747, #15992 ) ;
#2192=CIRCLE ( 'NONE', #12945, 62.91752772691707207 ) ;
#2196=VERTEX_POINT ( 'NONE', #288 ) ;
#2197=EDGE_CURVE ( 'NONE', #4838, #15800, #3754, .T. ) ;
#2200=CIRCLE ( 'NONE', #13267, 62.91752772691707207 ) ;
#2201=DIRECTION ( 'NONE',  ( 1.000000000000000000, 0.000000000000000000, 0.000000000000000000 ) ) ;
#2202=AXIS2_PLACEMENT_3D ( 'NONE', #11602, #11695, #16325 ) ;
#2205=CARTESIAN_POINT ( 'NONE',  ( 60.68773558783009747, -2.629322876227576433, 283.5832628385307999 ) ) ;
#2207=CARTESIAN_POINT ( 'NONE',  ( -49.67518383744793908, 60.47951622432801599, 132.4711112102474146 ) ) ;
#2208=CARTESIAN_POINT ( 'NONE',  ( 11.73417718768048701, 61.81362617575105389, 132.4711112102474146 ) ) ;
#2210=CYLINDRICAL_SURFACE ( 'NONE', #11021, 60.74260934110282051 ) ;
#2211=VERTEX_POINT ( 'NONE', #11225 ) ;
#2215=VERTEX_POINT ( 'NONE', #1930 ) ;
#2216=VECTOR ( 'NONE', #15404, 1000.000000000000000 ) ;
#2219=ADVANCED_FACE ( 'NONE', ( #8160, #3563 ), #14406, .F. ) ;
#2221=LINE ( 'NONE', #6824, #4008 ) ;
#2222=CARTESIAN_POINT ( 'NONE',  ( -58.69016442926522359, 0.8220851292433277724, 112.7772637782949516 ) ) ;
#2223=DIRECTION ( 'NONE',  ( 1.000000000000000000, 0.000000000000000000, -0.000000000000000000 ) ) ;
#2224=ORIENTED_EDGE ( 'NONE', *, *, #4993, .F. ) ;
#2225=DIRECTION ( 'NONE',  ( -0.8830229359480271656, -0.4693298356057563625, 0.000000000000000000 ) ) ;
#2226=DIRECTION ( 'NONE',  ( 0.000000000000000000, 0.000000000000000000, -1.000000000000000000 ) ) ;
#2228=DIRECTION ( 'NONE',  ( -0.9396926207859114255, 0.3420201433256601642, 0.000000000000000000 ) ) ;
#2229=ADVANCED_FACE ( 'NONE', ( #12862 ), #19118, .T. ) ;
#2230=DIRECTION ( 'NONE',  ( 0.000000000000000000, 0.000000000000000000, -1.000000000000000000 ) ) ;
#2232=DIRECTION ( 'NONE',  ( -0.000000000000000000, -0.000000000000000000, 1.000000000000000000 ) ) ;
#2236=ORIENTED_EDGE ( 'NONE', *, *, #6635, .T. ) ;
#2241=EDGE_CURVE ( 'NONE', #11142, #16800, #8256, .T. ) ;
#2244=VECTOR ( 'NONE', #7986, 1000.000000000000000 ) ;
#2248=CARTESIAN_POINT ( 'NONE',  ( -0.8220851292435327196, -58.69016442926522359, 132.4711112102474146 ) ) ;
#2249=DIRECTION ( 'NONE',  ( 1.000000000000000000, 0.000000000000000000, 0.000000000000000000 ) ) ;
#2252=LINE ( 'NONE', #7901, #9997 ) ;
#2254=VECTOR ( 'NONE', #1710, 999.9999999999998863 ) ;
#2258=EDGE_CURVE ( 'NONE', #3545, #1477, #10380, .T. ) ;
#2263=CARTESIAN_POINT ( 'NONE',  ( 59.30917539369505675, -13.12769224524051559, 293.5832628385307999 ) ) ;
#2264=CARTESIAN_POINT ( 'NONE',  ( 30.25670013172214468, 55.16472960512381718, 248.9926560891072143 ) ) ;
#2265=CARTESIAN_POINT ( 'NONE',  ( 56.12662799072089115, -23.22641211976269915, 283.5832628385307999 ) ) ;
#2266=VERTEX_POINT ( 'NONE', #2331 ) ;
#2267=CARTESIAN_POINT ( 'NONE',  ( 0.000000000000000000, 0.000000000000000000, 283.5832628385307999 ) ) ;
#2268=DIRECTION ( 'NONE',  ( 0.000000000000000000, 0.000000000000000000, 1.000000000000000000 ) ) ;
#2272=EDGE_CURVE ( 'NONE', #10094, #5816, #16345, .T. ) ;
#2275=CARTESIAN_POINT ( 'NONE',  ( 18.28567271940513450, -57.92709869106715814, 293.5832628385307999 ) ) ;
#2276=DIRECTION ( 'NONE',  ( 0.9511061040868794558, 0.3088643371590157338, 0.000000000000000000 ) ) ;
#2277=EDGE_LOOP ( 'NONE', ( #15901, #13040, #15804, #4684 ) ) ;
#2278=LINE ( 'NONE', #17634, #4022 ) ;
#2283=EDGE_CURVE ( 'NONE', #1965, #14511, #6892, .T. ) ;
#2285=DIRECTION ( 'NONE',  ( -1.000000000000000000, -3.491481338843133355E-15, 0.000000000000000000 ) ) ;
#2289=VECTOR ( 'NONE', #6610, 999.9999999999998863 ) ;
#2290=DIRECTION ( 'NONE',  ( 0.7881095627315598540, 0.6155349844899715706, 0.000000000000000000 ) ) ;
#2291=AXIS2_PLACEMENT_3D ( 'NONE', #12830, #1794, #19383 ) ;
#2296=EDGE_LOOP ( 'NONE', ( #15493, #6815, #15055 ) ) ;
#2297=VERTEX_POINT ( 'NONE', #7421 ) ;
#2299=DIRECTION ( 'NONE',  ( -0.000000000000000000, -0.000000000000000000, 1.000000000000000000 ) ) ;
#2301=CARTESIAN_POINT ( 'NONE',  ( 40.28046525994349736, 45.46865632508086463, 293.5832628385307999 ) ) ;
#2303=LINE ( 'NONE', #6999, #13247 ) ;
#2304=CARTESIAN_POINT ( 'NONE',  ( 40.32479851956816930, -67.08601213326552681, 110.9660488491356887 ) ) ;
#2305=LINE ( 'NONE', #8535, #630 ) ;
#2309=FACE_OUTER_BOUND ( 'NONE', #7114, .T. ) ;
#2310=EDGE_CURVE ( 'NONE', #6039, #2071, #7226, .T. ) ;
#2313=CIRCLE ( 'NONE', #14729, 62.91752772691707207 ) ;
#2314=ORIENTED_EDGE ( 'NONE', *, *, #5915, .F. ) ;
#2315=VERTEX_POINT ( 'NONE', #16448 ) ;
#2316=VERTEX_POINT ( 'NONE', #5797 ) ;
#2317=CARTESIAN_POINT ( 'NONE',  ( -22.28973221005119854, -58.83691981461626597, 132.4711112102474146 ) ) ;
#2318=ORIENTED_EDGE ( 'NONE', *, *, #14758, .F. ) ;
#2320=VECTOR ( 'NONE', #4053, 1000.000000000000000 ) ;
#2321=CARTESIAN_POINT ( 'NONE',  ( 0.000000000000000000, 0.000000000000000000, 283.5832628385307999 ) ) ;
#2322=LINE ( 'NONE', #6827, #10687 ) ;
#2323=ORIENTED_EDGE ( 'NONE', *, *, #16512, .F. ) ;
#2325=CARTESIAN_POINT ( 'NONE',  ( -60.08127757648377809, -8.938941455415188031, 283.5832628385307999 ) ) ;
#2326=FACE_OUTER_BOUND ( 'NONE', #14080, .T. ) ;
#2327=ORIENTED_EDGE ( 'NONE', *, *, #17123, .F. ) ;
#2329=PLANE ( 'NONE',  #11328 ) ;
#2331=CARTESIAN_POINT ( 'NONE',  ( 53.78543575132128751, 32.64570716507559212, 132.4711112102474146 ) ) ;
#2332=DIRECTION ( 'NONE',  ( -0.03505990758545895342, -0.9993852124581886764, 0.000000000000000000 ) ) ;
#2338=VECTOR ( 'NONE', #15590, 1000.000000000000000 ) ;
#2343=FACE_OUTER_BOUND ( 'NONE', #8614, .T. ) ;
#2346=EDGE_LOOP ( 'NONE', ( #12795, #11604, #8860 ) ) ;
#2347=FACE_OUTER_BOUND ( 'NONE', #11343, .T. ) ;
#2348=DIRECTION ( 'NONE',  ( 0.000000000000000000, 0.000000000000000000, -1.000000000000000000 ) ) ;
#2349=EDGE_CURVE ( 'NONE', #15754, #10590, #17356, .T. ) ;
#2350=DIRECTION ( 'NONE',  ( 0.000000000000000000, 0.000000000000000000, -1.000000000000000000 ) ) ;
#2351=DIRECTION ( 'NONE',  ( 0.000000000000000000, 0.000000000000000000, 1.000000000000000000 ) ) ;
#2352=DIRECTION ( 'NONE',  ( 1.000000000000000000, 0.000000000000000000, 0.000000000000000000 ) ) ;
#2353=VECTOR ( 'NONE', #15401, 999.9999999999998863 ) ;
#2354=DIRECTION ( 'NONE',  ( -0.000000000000000000, -0.000000000000000000, 1.000000000000000000 ) ) ;
#2355=DIRECTION ( 'NONE',  ( -0.000000000000000000, -0.000000000000000000, 1.000000000000000000 ) ) ;
#2358=FACE_OUTER_BOUND ( 'NONE', #6365, .T. ) ;
#2363=EDGE_CURVE ( 'NONE', #7427, #6858, #4254, .T. ) ;
#2364=EDGE_CURVE ( 'NONE', #12693, #13684, #2725, .T. ) ;
#2365=EDGE_CURVE ( 'NONE', #6701, #14795, #785, .T. ) ;
#2369=VECTOR ( 'NONE', #1650, 1000.000000000000000 ) ;
#2373=AXIS2_PLACEMENT_3D ( 'NONE', #14, #6162, #13605 ) ;
#2374=ADVANCED_FACE ( 'NONE', ( #5495 ), #879, .F. ) ;
#2376=DIRECTION ( 'NONE',  ( -0.9848077530122069101, -0.1736481776669374644, 0.000000000000000000 ) ) ;
#2377=DIRECTION ( 'NONE',  ( -0.000000000000000000, -0.000000000000000000, 1.000000000000000000 ) ) ;
#2380=DIRECTION ( 'NONE',  ( -0.6427876096865328126, -0.7660444431189835646, 0.000000000000000000 ) ) ;
#2381=ORIENTED_EDGE ( 'NONE', *, *, #13160, .F. ) ;
#2382=CARTESIAN_POINT ( 'NONE',  ( -47.29944656917786006, -41.48948842197101783, 132.4711112102474146 ) ) ;
#2383=LINE ( 'NONE', #13505, #4989 ) ;
#2386=ORIENTED_EDGE ( 'NONE', *, *, #11638, .F. ) ;
#2389=CIRCLE ( 'NONE', #9248, 60.74260934110282051 ) ;
#2391=EDGE_CURVE ( 'NONE', #11413, #3145, #18075, .T. ) ;
#2392=CARTESIAN_POINT ( 'NONE',  ( 41.48948842197120257, -47.29944656917771795, 248.9926560891072143 ) ) ;
#2393=EDGE_LOOP ( 'NONE', ( #8249, #12308, #8871, #7667 ) ) ;
#2394=CARTESIAN_POINT ( 'NONE',  ( -12.28122767885804301, 61.70726652483831032, 293.5832628385307999 ) ) ;
#2395=VECTOR ( 'NONE', #1636, 1000.000000000000114 ) ;
#2396=DIRECTION ( 'NONE',  ( -0.8660254037844397068, 0.4999999999999978906, 0.000000000000000000 ) ) ;
#2397=VECTOR ( 'NONE', #10548, 999.9999999999998863 ) ;
#2398=PLANE ( 'NONE',  #7187 ) ;
#2399=ORIENTED_EDGE ( 'NONE', *, *, #639, .T. ) ;
#2406=DIRECTION ( 'NONE',  ( 0.1390141521205946196, -0.9902903945359624593, 0.000000000000000000 ) ) ;
#2407=ORIENTED_EDGE ( 'NONE', *, *, #11939, .T. ) ;
#2408=AXIS2_PLACEMENT_3D ( 'NONE', #8178, #15859, #11038 ) ;
#2411=EDGE_LOOP ( 'NONE', ( #15328, #17475, #19860 ) ) ;
#2412=ADVANCED_FACE ( 'NONE', ( #16837 ), #10580, .F. ) ;
#2413=ADVANCED_FACE ( 'NONE', ( #20106 ), #12320, .F. ) ;
#2414=VERTEX_POINT ( 'NONE', #6213 ) ;
#2415=ORIENTED_EDGE ( 'NONE', *, *, #14270, .F. ) ;
#2416=AXIS2_PLACEMENT_3D ( 'NONE', #829, #4097, #2675 ) ;
#2417=EDGE_CURVE ( 'NONE', #15008, #14612, #3136, .T. ) ;
#2418=FACE_OUTER_BOUND ( 'NONE', #11261, .T. ) ;
#2419=PLANE ( 'NONE',  #7311 ) ;
#2420=AXIS2_PLACEMENT_3D ( 'NONE', #12570, #15958, #6752 ) ;
#2423=EDGE_CURVE ( 'NONE', #16849, #2942, #4352, .T. ) ;
#2427=DIRECTION ( 'NONE',  ( -0.000000000000000000, -0.000000000000000000, 1.000000000000000000 ) ) ;
#2428=CARTESIAN_POINT ( 'NONE',  ( 56.12853591711344592, -23.22718332831461652, 293.5832628385307999 ) ) ;
#2433=ORIENTED_EDGE ( 'NONE', *, *, #5628, .T. ) ;
#2434=LINE ( 'NONE', #14806, #18076 ) ;
#2435=VECTOR ( 'NONE', #8325, 1000.000000000000000 ) ;
#2436=ORIENTED_EDGE ( 'NONE', *, *, #1365, .T. ) ;
#2441=LINE ( 'NONE', #18291, #10714 ) ;
#2442=DIRECTION ( 'NONE',  ( 0.000000000000000000, 0.000000000000000000, 1.000000000000000000 ) ) ;
#2443=CIRCLE ( 'NONE', #11896, 60.74260934110282051 ) ;
#2447=PLANE ( 'NONE',  #2829 ) ;
#2451=ORIENTED_EDGE ( 'NONE', *, *, #19518, .F. ) ;
#2453=FACE_OUTER_BOUND ( 'NONE', #19304, .T. ) ;
#2454=VECTOR ( 'NONE', #10499, 1000.000000000000000 ) ;
#2455=DIRECTION ( 'NONE',  ( -1.047444401652940164E-14, 1.000000000000000000, 0.000000000000000000 ) ) ;
#2460=VECTOR ( 'NONE', #7444, 1000.000000000000114 ) ;
#2461=ORIENTED_EDGE ( 'NONE', *, *, #4643, .T. ) ;
#2463=ORIENTED_EDGE ( 'NONE', *, *, #12973, .T. ) ;
#2465=LINE ( 'NONE', #16778, #7493 ) ;
#2467=ORIENTED_EDGE ( 'NONE', *, *, #14472, .T. ) ;
#2468=CIRCLE ( 'NONE', #20097, 62.91752772691707207 ) ;
#2469=CARTESIAN_POINT ( 'NONE',  ( -28.06281046684226155, 73.06915264522029929, 132.4711112102474146 ) ) ;
#2470=CYLINDRICAL_SURFACE ( 'NONE', #11588, 60.74260934110282051 ) ;
#2472=DIRECTION ( 'NONE',  ( 0.000000000000000000, 0.000000000000000000, 1.000000000000000000 ) ) ;
#2473=DIRECTION ( 'NONE',  ( 0.000000000000000000, 0.000000000000000000, 1.000000000000000000 ) ) ;
#2478=DIRECTION ( 'NONE',  ( -0.9848077530122096857, 0.1736481776669206722, -0.000000000000000000 ) ) ;
#2480=ADVANCED_FACE ( 'NONE', ( #18584 ), #15299, .F. ) ;
#2483=CIRCLE ( 'NONE', #13907, 62.91752772691707207 ) ;
#2484=ORIENTED_EDGE ( 'NONE', *, *, #786, .F. ) ;
#2487=DIRECTION ( 'NONE',  ( -1.000000000000000000, 0.000000000000000000, 0.000000000000000000 ) ) ;
#2488=EDGE_LOOP ( 'NONE', ( #16772, #13380, #16877, #18182 ) ) ;
#2489=LINE ( 'NONE', #2592, #1759 ) ;
#2491=VECTOR ( 'NONE', #8817, 1000.000000000000000 ) ;
#2497=EDGE_CURVE ( 'NONE', #9731, #10444, #20002, .T. ) ;
#2498=LINE ( 'NONE', #4027, #11802 ) ;
#2500=CYLINDRICAL_SURFACE ( 'NONE', #14085, 60.74260934110282051 ) ;
#2507=EDGE_LOOP ( 'NONE', ( #426, #4398, #13594, #12738 ) ) ;
#2510=EDGE_CURVE ( 'NONE', #13906, #6775, #15510, .T. ) ;
#2511=ORIENTED_EDGE ( 'NONE', *, *, #5394, .T. ) ;
#2514=DIRECTION ( 'NONE',  ( 0.000000000000000000, 0.000000000000000000, 1.000000000000000000 ) ) ;
#2515=VERTEX_POINT ( 'NONE', #12431 ) ;
#2518=ORIENTED_EDGE ( 'NONE', *, *, #13762, .F. ) ;
#2519=FACE_OUTER_BOUND ( 'NONE', #19627, .T. ) ;
#2521=CARTESIAN_POINT ( 'NONE',  ( 19.23614321207236699, -57.61627707419557964, 283.5832628385307999 ) ) ;
#2522=ADVANCED_FACE ( 'NONE', ( #6314 ), #14073, .F. ) ;
#2523=EDGE_CURVE ( 'NONE', #9872, #2821, #17153, .T. ) ;
#2524=DIRECTION ( 'NONE',  ( 0.7660444431189749048, 0.6427876096865430267, 0.000000000000000000 ) ) ;
#2526=EDGE_CURVE ( 'NONE', #19300, #241, #9056, .T. ) ;
#2527=VECTOR ( 'NONE', #13993, 1000.000000000000000 ) ;
#2530=ORIENTED_EDGE ( 'NONE', *, *, #1259, .T. ) ;
#2534=LINE ( 'NONE', #19706, #14792 ) ;
#2536=ORIENTED_EDGE ( 'NONE', *, *, #17351, .T. ) ;
#2537=ORIENTED_EDGE ( 'NONE', *, *, #874, .T. ) ;
#2539=DIRECTION ( 'NONE',  ( -0.4999999999999950040, -0.8660254037844415942, -0.000000000000000000 ) ) ;
#2544=ORIENTED_EDGE ( 'NONE', *, *, #14981, .T. ) ;
#2546=DIRECTION ( 'NONE',  ( 0.000000000000000000, 0.000000000000000000, -1.000000000000000000 ) ) ;
#2549=DIRECTION ( 'NONE',  ( 0.000000000000000000, 0.000000000000000000, 1.000000000000000000 ) ) ;
#2552=DIRECTION ( 'NONE',  ( 1.000000000000000000, 1.047444401652940164E-14, 0.000000000000000000 ) ) ;
#2554=ADVANCED_FACE ( 'NONE', ( #3334 ), #9574, .F. ) ;
#2557=FACE_OUTER_BOUND ( 'NONE', #18623, .T. ) ;
#2560=VERTEX_POINT ( 'NONE', #5184 ) ;
#2561=DIRECTION ( 'NONE',  ( -0.000000000000000000, -0.000000000000000000, 1.000000000000000000 ) ) ;
#2563=DIRECTION ( 'NONE',  ( -0.000000000000000000, -0.000000000000000000, 1.000000000000000000 ) ) ;
#2564=ORIENTED_EDGE ( 'NONE', *, *, #4298, .T. ) ;
#2570=CIRCLE ( 'NONE', #19562, 60.74260934110282051 ) ;
#2572=PLANE ( 'NONE',  #4263 ) ;
#2573=CARTESIAN_POINT ( 'NONE',  ( 0.000000000000000000, 0.000000000000000000, 293.5832628385307999 ) ) ;
#2574=DIRECTION ( 'NONE',  ( -0.6427876096865379196, -0.7660444431189792347, 0.000000000000000000 ) ) ;
#2575=LINE ( 'NONE', #9952, #2949 ) ;
#2581=CARTESIAN_POINT ( 'NONE',  ( 9.564549117045078930, 62.18629025319817316, 293.5832628385307999 ) ) ;
#2586=AXIS2_PLACEMENT_3D ( 'NONE', #852, #7202, #14865 ) ;
#2590=CARTESIAN_POINT ( 'NONE',  ( -49.24833719034228352, -60.83768308848361528, 248.9926560891072143 ) ) ;
#2591=ORIENTED_EDGE ( 'NONE', *, *, #9613, .F. ) ;
#2592=CARTESIAN_POINT ( 'NONE',  ( 13.12726406102080112, 59.30716253403179650, 283.5832628385307999 ) ) ;
#2594=CARTESIAN_POINT ( 'NONE',  ( 17.50000000000001066, 0.000000000000000000, 4.999999999999948486 ) ) ;
#2599=VECTOR ( 'NONE', #20201, 1000.000000000000000 ) ;
#2602=CARTESIAN_POINT ( 'NONE',  ( 12.78021302872850562, -77.21438937758507848, 132.4711112102474146 ) ) ;
#2603=CARTESIAN_POINT ( 'NONE',  ( -2.605298826210324936, -5.111158570922258448, 283.5832628385307999 ) ) ;
#2604=FACE_OUTER_BOUND ( 'NONE', #5188, .T. ) ;
#2605=CARTESIAN_POINT ( 'NONE',  ( 36.99514631729018532, -48.17959877923561862, 293.5832628385307999 ) ) ;
#2607=EDGE_CURVE ( 'NONE', #14365, #6558, #9772, .T. ) ;
#2608=ORIENTED_EDGE ( 'NONE', *, *, #12902, .T. ) ;
#2609=EDGE_CURVE ( 'NONE', #12970, #8067, #17759, .T. ) ;
#2610=ORIENTED_EDGE ( 'NONE', *, *, #19884, .F. ) ;
#2611=VERTEX_POINT ( 'NONE', #5280 ) ;
#2612=VERTEX_POINT ( 'NONE', #3436 ) ;
#2613=EDGE_CURVE ( 'NONE', #12685, #17, #6713, .T. ) ;
#2615=EDGE_CURVE ( 'NONE', #6960, #12583, #569, .T. ) ;
#2617=PLANE ( 'NONE',  #4715 ) ;
#2620=LINE ( 'NONE', #14595, #9339 ) ;
#2621=DIRECTION ( 'NONE',  ( 0.1736481776669340504, -0.9848077530122074652, 0.000000000000000000 ) ) ;
#2622=ORIENTED_EDGE ( 'NONE', *, *, #15684, .T. ) ;
#2633=ORIENTED_EDGE ( 'NONE', *, *, #12260, .T. ) ;
#2635=VERTEX_POINT ( 'NONE', #16023 ) ;
#2638=VERTEX_POINT ( 'NONE', #11506 ) ;
#2639=ORIENTED_EDGE ( 'NONE', *, *, #16795, .F. ) ;
#2640=EDGE_CURVE ( 'NONE', #108, #15181, #12632, .T. ) ;
#2641=VECTOR ( 'NONE', #8283, 1000.000000000000000 ) ;
#2642=ADVANCED_FACE ( 'NONE', ( #12835 ), #19094, .F. ) ;
#2646=CARTESIAN_POINT ( 'NONE',  ( -20.21777810286715749, -59.58067424803620327, 248.9926560891072143 ) ) ;
#2647=CARTESIAN_POINT ( 'NONE',  ( -1.629865514042508456, -60.72073886220396588, 283.5832628385307999 ) ) ;
#2650=CARTESIAN_POINT ( 'NONE',  ( -55.62246070845768031, 18.77710619359134725, 111.4180192758973931 ) ) ;
#2653=AXIS2_PLACEMENT_3D ( 'NONE', #6003, #20209, #1599 ) ;
#2655=ADVANCED_FACE ( 'NONE', ( #17565 ), #18998, .T. ) ;
#2656=DIRECTION ( 'NONE',  ( -0.000000000000000000, -0.000000000000000000, 1.000000000000000000 ) ) ;
#2658=CARTESIAN_POINT ( 'NONE',  ( -73.82206860051547892, -25.99419088092166774, 248.9926560891072143 ) ) ;
#2661=PLANE ( 'NONE',  #20031 ) ;
#2662=ORIENTED_EDGE ( 'NONE', *, *, #17555, .F. ) ;
#2664=CARTESIAN_POINT ( 'NONE',  ( 62.09913334491123038, 10.11498556985180208, 248.9926560891072143 ) ) ;
#2666=ADVANCED_FACE ( 'NONE', ( #467 ), #2210, .F. ) ;
#2669=DIRECTION ( 'NONE',  ( 0.5300553768524375320, 0.8479630283625697595, 0.000000000000000000 ) ) ;
#2675=DIRECTION ( 'NONE',  ( 0.8660254037844432595, -0.4999999999999919509, 0.000000000000000000 ) ) ;
#2684=ORIENTED_EDGE ( 'NONE', *, *, #18277, .T. ) ;
#2686=ORIENTED_EDGE ( 'NONE', *, *, #874, .F. ) ;
#2687=DIRECTION ( 'NONE',  ( -0.000000000000000000, -0.000000000000000000, 1.000000000000000000 ) ) ;
#2690=CARTESIAN_POINT ( 'NONE',  ( 57.92709869106709419, 18.28567271940532990, 293.5832628385307999 ) ) ;
#2691=CARTESIAN_POINT ( 'NONE',  ( 39.84224160888901167, 67.36461649554546227, 132.4711112102474146 ) ) ;
#2693=DIRECTION ( 'NONE',  ( 0.6155349844899687950, -0.7881095627315619634, 0.000000000000000000 ) ) ;
#2694=LINE ( 'NONE', #16611, #1295 ) ;
#2695=EDGE_LOOP ( 'NONE', ( #5244, #10996, #7052, #10335 ) ) ;
#2696=LINE ( 'NONE', #7496, #3249 ) ;
#2699=VECTOR ( 'NONE', #9999, 1000.000000000000114 ) ;
#2701=DIRECTION ( 'NONE',  ( 0.7430374143461878633, -0.6692498792541777819, 0.000000000000000000 ) ) ;
#2703=CARTESIAN_POINT ( 'NONE',  ( 0.000000000000000000, 0.000000000000000000, 132.4711112102474146 ) ) ;
#2705=DIRECTION ( 'NONE',  ( 0.000000000000000000, 0.000000000000000000, 1.000000000000000000 ) ) ;
#2706=AXIS2_PLACEMENT_3D ( 'NONE', #11654, #2455, #16573 ) ;
#2709=ORIENTED_EDGE ( 'NONE', *, *, #9711, .T. ) ;
#2710=VECTOR ( 'NONE', #10438, 1000.000000000000114 ) ;
#2711=VECTOR ( 'NONE', #19308, 1000.000000000000114 ) ;
#2713=ADVANCED_FACE ( 'NONE', ( #2309 ), #11990, .T. ) ;
#2714=LINE ( 'NONE', #18463, #10907 ) ;
#2715=DIRECTION ( 'NONE',  ( 0.000000000000000000, 0.000000000000000000, 1.000000000000000000 ) ) ;
#2718=CARTESIAN_POINT ( 'NONE',  ( 0.000000000000000000, 0.000000000000000000, 283.5832628385307999 ) ) ;
#2723=CARTESIAN_POINT ( 'NONE',  ( 32.16802499836741447, 54.07248341783265033, 132.4711112102474146 ) ) ;
#2724=VECTOR ( 'NONE', #18519, 1000.000000000000000 ) ;
#2725=LINE ( 'NONE', #14894, #19946 ) ;
#2726=UNCERTAINTY_MEASURE_WITH_UNIT (LENGTH_MEASURE( 1.000000000000000082E-05 ), #7973, 'distance_accuracy_value', 'NONE');
#2728=CIRCLE ( 'NONE', #10226, 60.74260934110282051 ) ;
#2729=EDGE_CURVE ( 'NONE', #17, #6819, #11889, .T. ) ;
#2731=DIRECTION ( 'NONE',  ( 0.8830229359480271656, 0.4693298356057563625, 0.000000000000000000 ) ) ;
#2732=ORIENTED_EDGE ( 'NONE', *, *, #16984, .F. ) ;
#2733=ADVANCED_FACE ( 'NONE', ( #8541 ), #5674, .F. ) ;
#2734=CARTESIAN_POINT ( 'NONE',  ( 0.000000000000000000, 0.000000000000000000, 293.5832628385307999 ) ) ;
#2736=VECTOR ( 'NONE', #5458, 1000.000000000000227 ) ;
#2737=ORIENTED_EDGE ( 'NONE', *, *, #2001, .F. ) ;
#2740=EDGE_LOOP ( 'NONE', ( #9606, #6657, #17889, #14634 ) ) ;
#2742=ADVANCED_FACE ( 'NONE', ( #18149 ), #667, .F. ) ;
#2743=PLANE ( 'NONE',  #15642 ) ;
#2745=ORIENTED_EDGE ( 'NONE', *, *, #17241, .F. ) ;
#2746=CARTESIAN_POINT ( 'NONE',  ( 60.22029172860436574, 7.948651060879242003, 283.5832628385307999 ) ) ;
#2748=EDGE_LOOP ( 'NONE', ( #5728, #2433, #15269, #10800 ) ) ;
#2750=CARTESIAN_POINT ( 'NONE',  ( 51.24071425735604635, -32.61983739937743820, 283.5832628385307999 ) ) ;
#2751=DIRECTION ( 'NONE',  ( 1.000000000000000000, 0.000000000000000000, 0.000000000000000000 ) ) ;
#2754=VECTOR ( 'NONE', #9964, 1000.000000000000000 ) ;
#2755=DIRECTION ( 'NONE',  ( -0.4999999999999919509, -0.8660254037844432595, 0.000000000000000000 ) ) ;
#2756=EDGE_CURVE ( 'NONE', #6696, #17381, #14774, .T. ) ;
#2758=DIRECTION ( 'NONE',  ( 0.000000000000000000, 0.000000000000000000, 1.000000000000000000 ) ) ;
#2759=VERTEX_POINT ( 'NONE', #16425 ) ;
#2763=EDGE_LOOP ( 'NONE', ( #13219, #15319, #17788, #14443 ) ) ;
#2770=DIRECTION ( 'NONE',  ( 0.3747554100459959958, 0.9271237148521535021, 0.000000000000000000 ) ) ;
#2772=LINE ( 'NONE', #17198, #6405 ) ;
#2773=CARTESIAN_POINT ( 'NONE',  ( -41.06890862491506056, -47.66508197439456751, 293.5832628385307999 ) ) ;
#2774=VECTOR ( 'NONE', #12270, 999.9999999999998863 ) ;
#2775=CARTESIAN_POINT ( 'NONE',  ( 30.05702882063027914, 50.41613078340812848, 132.4711112102474146 ) ) ;
#2776=CARTESIAN_POINT ( 'NONE',  ( 73.25972925305627825, -27.53920554013664912, 111.4180192758974499 ) ) ;
#2777=CARTESIAN_POINT ( 'NONE',  ( 5.485913980968119219, -1.678175111358107374, 283.5832628385307999 ) ) ;
#2778=DIRECTION ( 'NONE',  ( 0.7660444431189792347, -0.6427876096865379196, 0.000000000000000000 ) ) ;
#2779=EDGE_CURVE ( 'NONE', #16780, #12002, #11792, .T. ) ;
#2781=CARTESIAN_POINT ( 'NONE',  ( 58.63718168490485283, 22.81000261549389307, 293.5832628385307999 ) ) ;
#2784=LINE ( 'NONE', #9005, #17741 ) ;
#2785=EDGE_CURVE ( 'NONE', #10983, #8668, #10673, .T. ) ;
#2787=DIRECTION ( 'NONE',  ( -0.5300553768524375320, -0.8479630283625697595, 0.000000000000000000 ) ) ;
#2788=CYLINDRICAL_SURFACE ( 'NONE', #8259, 60.74260934110282051 ) ;
#2789=ORIENTED_EDGE ( 'NONE', *, *, #1601, .T. ) ;
#2790=EDGE_CURVE ( 'NONE', #3549, #13282, #16580, .T. ) ;
#2792=VECTOR ( 'NONE', #3581, 1000.000000000000114 ) ;
#2794=FACE_BOUND ( 'NONE', #3280, .T. ) ;
#2795=ADVANCED_FACE ( 'NONE', ( #6914 ), #13123, .F. ) ;
#2796=ORIENTED_EDGE ( 'NONE', *, *, #6498, .F. ) ;
#2797=DIRECTION ( 'NONE',  ( -0.9271237148521547233, 0.3747554100459928872, 0.000000000000000000 ) ) ;
#2800=DIRECTION ( 'NONE',  ( 0.7660444431189858960, -0.6427876096865300370, 0.000000000000000000 ) ) ;
#2802=VECTOR ( 'NONE', #13870, 1000.000000000000114 ) ;
#2804=DIRECTION ( 'NONE',  ( 0.000000000000000000, 0.000000000000000000, -1.000000000000000000 ) ) ;
#2807=CARTESIAN_POINT ( 'NONE',  ( 14.39940464655707331, 76.92888220842492331, 248.9926560891072143 ) ) ;
#2808=COLOUR_RGB ( '', 0.08235294, 0.09019608, 0.10196078) ;
#2811=VERTEX_POINT ( 'NONE', #2908 ) ;
#2812=DIRECTION ( 'NONE',  ( -0.000000000000000000, -0.000000000000000000, 1.000000000000000000 ) ) ;
#2813=ADVANCED_FACE ( 'NONE', ( #18559 ), #4540, .F. ) ;
#2816=ORIENTED_EDGE ( 'NONE', *, *, #10850, .F. ) ;
#2821=VERTEX_POINT ( 'NONE', #1470 ) ;
#2824=ORIENTED_EDGE ( 'NONE', *, *, #14008, .F. ) ;
#2826=DIRECTION ( 'NONE',  ( -0.000000000000000000, -0.000000000000000000, 1.000000000000000000 ) ) ;
#2828=DIRECTION ( 'NONE',  ( 0.000000000000000000, 0.000000000000000000, -1.000000000000000000 ) ) ;
#2829=AXIS2_PLACEMENT_3D ( 'NONE', #2650, #11646, #4275 ) ;
#2830=AXIS2_PLACEMENT_3D ( 'NONE', #12441, #18906, #3149 ) ;
#2835=AXIS2_PLACEMENT_3D ( 'NONE', #14804, #788, #17986 ) ;
#2836=ORIENTED_EDGE ( 'NONE', *, *, #14143, .T. ) ;
#2837=CARTESIAN_POINT ( 'NONE',  ( 13.12726406102079224, 59.30716253403178939, 283.5832628385307999 ) ) ;
#2838=ORIENTED_EDGE ( 'NONE', *, *, #13359, .F. ) ;
#2841=ORIENTED_EDGE ( 'NONE', *, *, #9752, .F. ) ;
#2843=AXIS2_PLACEMENT_3D ( 'NONE', #10891, #18373, #13860 ) ;
#2844=DIRECTION ( 'NONE',  ( 1.000000000000000000, 0.000000000000000000, 0.000000000000000000 ) ) ;
#2845=EDGE_CURVE ( 'NONE', #10590, #12690, #3011, .T. ) ;
#2848=DIRECTION ( 'NONE',  ( 0.000000000000000000, 0.000000000000000000, -1.000000000000000000 ) ) ;
#2849=DIRECTION ( 'NONE',  ( 0.000000000000000000, 0.000000000000000000, 1.000000000000000000 ) ) ;
#2850=ORIENTED_EDGE ( 'NONE', *, *, #3861, .T. ) ;
#2853=LINE ( 'NONE', #10502, #19550 ) ;
#2854=LINE ( 'NONE', #15324, #8004 ) ;
#2855=DIRECTION ( 'NONE',  ( 0.000000000000000000, 0.000000000000000000, -1.000000000000000000 ) ) ;
#2862=EDGE_LOOP ( 'NONE', ( #14694, #5284, #9035, #19113 ) ) ;
#2865=VECTOR ( 'NONE', #17692, 1000.000000000000000 ) ;
#2867=ORIENTED_EDGE ( 'NONE', *, *, #5371, .T. ) ;
#2869=ADVANCED_FACE ( 'NONE', ( #5878 ), #12506, .F. ) ;
#2870=DIRECTION ( 'NONE',  ( 1.000000000000000000, 1.047444401652940164E-14, 0.000000000000000000 ) ) ;
#2871=ORIENTED_EDGE ( 'NONE', *, *, #19281, .F. ) ;
#2875=VECTOR ( 'NONE', #7513, 999.9999999999998863 ) ;
#2882=ORIENTED_EDGE ( 'NONE', *, *, #2729, .F. ) ;
#2884=DIRECTION ( 'NONE',  ( -0.000000000000000000, -0.000000000000000000, 1.000000000000000000 ) ) ;
#2885=DIRECTION ( 'NONE',  ( -0.6692498792541753394, -0.7430374143461900838, 0.000000000000000000 ) ) ;
#2886=VERTEX_POINT ( 'NONE', #7500 ) ;
#2887=VERTEX_POINT ( 'NONE', #9344 ) ;
#2890=VECTOR ( 'NONE', #15854, 1000.000000000000000 ) ;
#2891=EDGE_LOOP ( 'NONE', ( #19002, #5002, #4917, #11329 ) ) ;
#2892=AXIS2_PLACEMENT_3D ( 'NONE', #6574, #11259, #15770 ) ;
#2894=ORIENTED_EDGE ( 'NONE', *, *, #8297, .F. ) ;
#2895=EDGE_CURVE ( 'NONE', #18152, #959, #7397, .T. ) ;
#2896=FACE_OUTER_BOUND ( 'NONE', #11235, .T. ) ;
#2900=LINE ( 'NONE', #4219, #4732 ) ;
#2904=DIRECTION ( 'NONE',  ( -0.1736481776669172583, -0.9848077530122103518, -0.000000000000000000 ) ) ;
#2908=CARTESIAN_POINT ( 'NONE',  ( -58.83691981461619491, 22.28973221005138683, 248.9926560891072143 ) ) ;
#2911=AXIS2_PLACEMENT_3D ( 'NONE', #20183, #15963, #4534 ) ;
#2913=VECTOR ( 'NONE', #10890, 1000.000000000000000 ) ;
#2916=ORIENTED_EDGE ( 'NONE', *, *, #6756, .F. ) ;
#2922=DIRECTION ( 'NONE',  ( 1.000000000000000000, 0.000000000000000000, 0.000000000000000000 ) ) ;
#2924=LINE ( 'NONE', #18685, #6749 ) ;
#2925=CARTESIAN_POINT ( 'NONE',  ( 60.68773558783009747, -2.629322876227576433, 293.5832628385307999 ) ) ;
#2927=ORIENTED_EDGE ( 'NONE', *, *, #11824, .T. ) ;
#2928=CARTESIAN_POINT ( 'NONE',  ( 0.000000000000000000, 0.000000000000000000, 283.5832628385307999 ) ) ;
#2932=CARTESIAN_POINT ( 'NONE',  ( -22.30005961346265408, -56.50329132715937419, 283.5832628385307999 ) ) ;
#2933=DIRECTION ( 'NONE',  ( 0.9396926207859105373, -0.3420201433256631063, 0.000000000000000000 ) ) ;
#2934=DIRECTION ( 'NONE',  ( -0.8479630283625716469, 0.5300553768524345344, 0.000000000000000000 ) ) ;
#2938=ORIENTED_EDGE ( 'NONE', *, *, #7908, .F. ) ;
#2942=VERTEX_POINT ( 'NONE', #18453 ) ;
#2943=DIRECTION ( 'NONE',  ( 0.000000000000000000, 0.000000000000000000, 1.000000000000000000 ) ) ;
#2946=CARTESIAN_POINT ( 'NONE',  ( 55.43188410062170135, 19.30071112029698455, 132.4711112102474146 ) ) ;
#2949=VECTOR ( 'NONE', #15049, 1000.000000000000000 ) ;
#2950=DIRECTION ( 'NONE',  ( 0.8660254037844397068, -0.4999999999999979461, -0.000000000000000000 ) ) ;
#2951=ORIENTED_EDGE ( 'NONE', *, *, #9711, .F. ) ;
#2954=CARTESIAN_POINT ( 'NONE',  ( -12.11787020633453338, 60.78082026081703049, 248.9926560891072143 ) ) ;
#2962=VERTEX_POINT ( 'NONE', #12200 ) ;
#2963=CARTESIAN_POINT ( 'NONE',  ( -32.61983739937760873, -51.24071425735591134, 283.5832628385307999 ) ) ;
#2968=DIRECTION ( 'NONE',  ( 0.9511061040868794558, 0.3088643371590157338, 0.000000000000000000 ) ) ;
#2971=DIRECTION ( 'NONE',  ( 1.000000000000000000, 0.000000000000000000, 0.000000000000000000 ) ) ;
#2974=DIRECTION ( 'NONE',  ( 0.1736481776669306920, -0.9848077530122080203, 0.000000000000000000 ) ) ;
#2977=VECTOR ( 'NONE', #20187, 1000.000000000000000 ) ;
#2979=DIRECTION ( 'NONE',  ( 0.000000000000000000, 0.000000000000000000, 1.000000000000000000 ) ) ;
#2983=FACE_OUTER_BOUND ( 'NONE', #18034, .T. ) ;
#2984=CARTESIAN_POINT ( 'NONE',  ( 0.000000000000000000, 0.000000000000000000, 269.6944534026102360 ) ) ;
#2990=ADVANCED_FACE ( 'NONE', ( #9553 ), #17543, .T. ) ;
#2998=CARTESIAN_POINT ( 'NONE',  ( 0.000000000000000000, 65.74260934110282051, 293.5832628385307999 ) ) ;
#2999=ORIENTED_EDGE ( 'NONE', *, *, #17501, .T. ) ;
#3000=PLANE ( 'NONE',  #15796 ) ;
#3005=DIRECTION ( 'NONE',  ( -0.9848077530122097967, 0.1736481776669207000, 0.000000000000000000 ) ) ;
#3010=CARTESIAN_POINT ( 'NONE',  ( 31.86742755225487045, 24.93940645478198803, 248.9926560891072143 ) ) ;
#3011=LINE ( 'NONE', #6292, #19201 ) ;
#3013=ORIENTED_EDGE ( 'NONE', *, *, #17507, .F. ) ;
#3014=CARTESIAN_POINT ( 'NONE',  ( 0.000000000000000000, 0.000000000000000000, 248.9926560891072143 ) ) ;
#3018=EDGE_LOOP ( 'NONE', ( #7239, #4809, #7210, #12805 ) ) ;
#3020=ORIENTED_EDGE ( 'NONE', *, *, #14996, .T. ) ;
#3022=EDGE_CURVE ( 'NONE', #6905, #19150, #19274, .T. ) ;
#3023=DIRECTION ( 'NONE',  ( -0.000000000000000000, -0.000000000000000000, 1.000000000000000000 ) ) ;
#3029=DIRECTION ( 'NONE',  ( -0.1390141521205912334, 0.9902903945359629034, 0.000000000000000000 ) ) ;
#3033=CARTESIAN_POINT ( 'NONE',  ( -38.41834839689332171, 68.18670162478844077, 132.4711112102474146 ) ) ;
#3035=DIRECTION ( 'NONE',  ( -0.000000000000000000, -0.000000000000000000, 1.000000000000000000 ) ) ;
#3037=EDGE_CURVE ( 'NONE', #858, #1972, #9452, .T. ) ;
#3038=CARTESIAN_POINT ( 'NONE',  ( 14.39940464655707331, 76.92888220842492331, 132.4711112102474146 ) ) ;
#3039=PLANE ( 'NONE',  #1844 ) ;
#3040=ADVANCED_FACE ( 'NONE', ( #19077 ), #139, .F. ) ;
#3041=ORIENTED_EDGE ( 'NONE', *, *, #9659, .F. ) ;
#3042=ORIENTED_EDGE ( 'NONE', *, *, #12123, .T. ) ;
#3044=VECTOR ( 'NONE', #3203, 1000.000000000000227 ) ;
#3045=ORIENTED_EDGE ( 'NONE', *, *, #4288, .T. ) ;
#3050=FACE_OUTER_BOUND ( 'NONE', #13948, .T. ) ;
#3052=CARTESIAN_POINT ( 'NONE',  ( 0.000000000000000000, 0.000000000000000000, 283.5832628385307999 ) ) ;
#3055=ORIENTED_EDGE ( 'NONE', *, *, #5060, .F. ) ;
#3057=CARTESIAN_POINT ( 'NONE',  ( 0.000000000000000000, 0.000000000000000000, 293.5832628385307999 ) ) ;
#3059=CARTESIAN_POINT ( 'NONE',  ( 60.74260934110282051, 0.000000000000000000, 283.5832628385307999 ) ) ;
#3060=PLANE ( 'NONE',  #14982 ) ;
#3061=AXIS2_PLACEMENT_3D ( 'NONE', #19028, #12562, #19125 ) ;
#3064=VECTOR ( 'NONE', #19377, 999.9999999999998863 ) ;
#3070=EDGE_LOOP ( 'NONE', ( #18593, #11700, #19060 ) ) ;
#3071=ORIENTED_EDGE ( 'NONE', *, *, #8404, .T. ) ;
#3072=PLANE ( 'NONE',  #10075 ) ;
#3073=VERTEX_POINT ( 'NONE', #14561 ) ;
#3076=ORIENTED_EDGE ( 'NONE', *, *, #174, .F. ) ;
#3079=FACE_OUTER_BOUND ( 'NONE', #9975, .T. ) ;
#3080=VECTOR ( 'NONE', #17274, 1000.000000000000000 ) ;
#3081=DIRECTION ( 'NONE',  ( 0.6427876096865481337, -0.7660444431189707970, 0.000000000000000000 ) ) ;
#3083=EDGE_LOOP ( 'NONE', ( #10699, #7557, #17698, #16455 ) ) ;
#3084=CARTESIAN_POINT ( 'NONE',  ( -27.93373560431178149, 14.53487841505308253, 248.9926560891072143 ) ) ;
#3085=CARTESIAN_POINT ( 'NONE',  ( -55.62246070845768031, 18.77710619359134725, 132.4711112102474146 ) ) ;
#3086=DIRECTION ( 'NONE',  ( -0.9396926207859057634, -0.3420201433256757073, 0.000000000000000000 ) ) ;
#3090=PLANE ( 'NONE',  #19379 ) ;
#3091=ORIENTED_EDGE ( 'NONE', *, *, #13772, .T. ) ;
#3092=ADVANCED_FACE ( 'NONE', ( #6794 ), #14361, .F. ) ;
#3094=ORIENTED_EDGE ( 'NONE', *, *, #8335, .T. ) ;
#3096=VERTEX_POINT ( 'NONE', #15798 ) ;
#3098=DIRECTION ( 'NONE',  ( -1.000000000000000000, 0.000000000000000000, -0.000000000000000000 ) ) ;
#3102=CARTESIAN_POINT ( 'NONE',  ( 10.11498556985161201, -62.09913334491128012, 132.4711112102474146 ) ) ;
#3104=EDGE_CURVE ( 'NONE', #720, #4348, #1779, .T. ) ;
#3106=AXIS2_PLACEMENT_3D ( 'NONE', #5207, #11436, #17690 ) ;
#3107=CARTESIAN_POINT ( 'NONE',  ( -60.68567895461851691, 2.629250726500500956, 283.5832628385307999 ) ) ;
#3108=FACE_OUTER_BOUND ( 'NONE', #10710, .T. ) ;
#3110=FACE_OUTER_BOUND ( 'NONE', #6322, .T. ) ;
#3113=LINE ( 'NONE', #12090, #19962 ) ;
#3114=DIRECTION ( 'NONE',  ( -0.8660254037844450359, 0.4999999999999889533, 0.000000000000000000 ) ) ;
#3118=AXIS2_PLACEMENT_3D ( 'NONE', #6152, #16989, #11143 ) ;
#3120=ORIENTED_EDGE ( 'NONE', *, *, #14282, .T. ) ;
#3121=AXIS2_PLACEMENT_3D ( 'NONE', #12815, #9747, #11286 ) ;
#3122=VERTEX_POINT ( 'NONE', #16202 ) ;
#3123=ORIENTED_EDGE ( 'NONE', *, *, #18630, .T. ) ;
#3126=CARTESIAN_POINT ( 'NONE',  ( -48.72193424476477475, -39.80940113486002474, 293.5832628385307999 ) ) ;
#3127=VERTEX_POINT ( 'NONE', #3907 ) ;
#3130=CARTESIAN_POINT ( 'NONE',  ( 0.000000000000000000, 0.000000000000000000, 132.4711112102474146 ) ) ;
#3131=EDGE_CURVE ( 'NONE', #16066, #11398, #2189, .T. ) ;
#3133=CARTESIAN_POINT ( 'NONE',  ( 0.000000000000000000, 0.000000000000000000, 248.9926560891072143 ) ) ;
#3136=LINE ( 'NONE', #13863, #7215 ) ;
#3137=ORIENTED_EDGE ( 'NONE', *, *, #4494, .T. ) ;
#3138=CARTESIAN_POINT ( 'NONE',  ( 50.41613078340802190, -30.05702882063045678, 132.4711112102474146 ) ) ;
#3139=DIRECTION ( 'NONE',  ( 1.000000000000000000, 0.000000000000000000, 0.000000000000000000 ) ) ;
#3141=ORIENTED_EDGE ( 'NONE', *, *, #1905, .F. ) ;
#3142=ORIENTED_EDGE ( 'NONE', *, *, #234, .T. ) ;
#3143=EDGE_CURVE ( 'NONE', #10024, #7758, #13105, .T. ) ;
#3144=EDGE_LOOP ( 'NONE', ( #12259, #6178, #2436, #10219 ) ) ;
#3145=VERTEX_POINT ( 'NONE', #19652 ) ;
#3147=FACE_OUTER_BOUND ( 'NONE', #11028, .T. ) ;
#3148=ORIENTED_EDGE ( 'NONE', *, *, #14377, .T. ) ;
#3149=DIRECTION ( 'NONE',  ( -0.03505990758545895342, -0.9993852124581886764, 0.000000000000000000 ) ) ;
#3154=ORIENTED_EDGE ( 'NONE', *, *, #8387, .F. ) ;
#3155=EDGE_CURVE ( 'NONE', #18654, #14438, #11677, .T. ) ;
#3156=FACE_OUTER_BOUND ( 'NONE', #9656, .T. ) ;
#3161=VECTOR ( 'NONE', #11871, 1000.000000000000000 ) ;
#3164=CARTESIAN_POINT ( 'NONE',  ( -1.629937663769596368, -60.72279549541552512, 283.5832628385307999 ) ) ;
#3166=DIRECTION ( 'NONE',  ( 0.9511061040868794558, 0.3088643371590157338, 0.000000000000000000 ) ) ;
#3168=EDGE_LOOP ( 'NONE', ( #16357, #16408, #18289 ) ) ;
#3170=ORIENTED_EDGE ( 'NONE', *, *, #6606, .F. ) ;
#3173=LINE ( 'NONE', #9490, #2890 ) ;
#3175=ORIENTED_EDGE ( 'NONE', *, *, #7651, .T. ) ;
#3178=VERTEX_POINT ( 'NONE', #8612 ) ;
#3181=CYLINDRICAL_SURFACE ( 'NONE', #3762, 60.74260934110282051 ) ;
#3182=EDGE_CURVE ( 'NONE', #19763, #15222, #8517, .T. ) ;
#3183=FACE_OUTER_BOUND ( 'NONE', #6040, .T. ) ;
#3184=DIRECTION ( 'NONE',  ( -1.000000000000000000, 0.000000000000000000, 0.000000000000000000 ) ) ;
#3185=ORIENTED_EDGE ( 'NONE', *, *, #11384, .T. ) ;
#3186=DIRECTION ( 'NONE',  ( -0.2080686897406943958, -0.9781142164131909622, 0.000000000000000000 ) ) ;
#3187=DIRECTION ( 'NONE',  ( 1.000000000000000000, 0.000000000000000000, 0.000000000000000000 ) ) ;
#3188=CARTESIAN_POINT ( 'NONE',  ( 0.000000000000000000, 0.000000000000000000, 293.5832628385307999 ) ) ;
#3193=DIRECTION ( 'NONE',  ( -0.9396926207859082059, -0.3420201433256694901, 0.000000000000000000 ) ) ;
#3197=ORIENTED_EDGE ( 'NONE', *, *, #12775, .T. ) ;
#3199=VERTEX_POINT ( 'NONE', #644 ) ;
#3201=FACE_BOUND ( 'NONE', #761, .T. ) ;
#3203=DIRECTION ( 'NONE',  ( -0.4693298356057531429, 0.8830229359480288309, 0.000000000000000000 ) ) ;
#3204=CARTESIAN_POINT ( 'NONE',  ( -22.28973221005119854, -58.83691981461626597, 293.5832628385307999 ) ) ;
#3211=DIRECTION ( 'NONE',  ( -0.7660444431189858960, 0.6427876096865300370, 0.000000000000000000 ) ) ;
#3214=ORIENTED_EDGE ( 'NONE', *, *, #14917, .F. ) ;
#3215=DIRECTION ( 'NONE',  ( 0.000000000000000000, 0.000000000000000000, 1.000000000000000000 ) ) ;
#3216=VECTOR ( 'NONE', #15911, 1000.000000000000000 ) ;
#3217=VECTOR ( 'NONE', #7258, 1000.000000000000114 ) ;
#3218=ORIENTED_EDGE ( 'NONE', *, *, #12083, .F. ) ;
#3219=VERTEX_POINT ( 'NONE', #16306 ) ;
#3220=VERTEX_POINT ( 'NONE', #6888 ) ;
#3221=DIRECTION ( 'NONE',  ( -0.000000000000000000, -0.000000000000000000, 1.000000000000000000 ) ) ;
#3222=DIRECTION ( 'NONE',  ( -0.000000000000000000, -0.000000000000000000, 1.000000000000000000 ) ) ;
#3225=AXIS2_PLACEMENT_3D ( 'NONE', #18622, #18315, #4291 ) ;
#3232=CARTESIAN_POINT ( 'NONE',  ( -76.92888220842476699, 14.39940464655786201, 248.9926560891072143 ) ) ;
#3234=ORIENTED_EDGE ( 'NONE', *, *, #4154, .T. ) ;
#3240=ORIENTED_EDGE ( 'NONE', *, *, #7995, .T. ) ;
#3241=EDGE_CURVE ( 'NONE', #13065, #12180, #18124, .T. ) ;
#3244=AXIS2_PLACEMENT_3D ( 'NONE', #6130, #11124, #10920 ) ;
#3245=VECTOR ( 'NONE', #14198, 1000.000000000000000 ) ;
#3246=ORIENTED_EDGE ( 'NONE', *, *, #3297, .F. ) ;
#3247=EDGE_CURVE ( 'NONE', #11476, #244, #14944, .T. ) ;
#3248=CARTESIAN_POINT ( 'NONE',  ( -1.629937663769596368, -60.72279549541552512, 293.5832628385307999 ) ) ;
#3249=VECTOR ( 'NONE', #11986, 1000.000000000000000 ) ;
#3251=LINE ( 'NONE', #13977, #14909 ) ;
#3252=PLANE ( 'NONE',  #4338 ) ;
#3256=VERTEX_POINT ( 'NONE', #16591 ) ;
#3263=VECTOR ( 'NONE', #15575, 1000.000000000000000 ) ;
#3268=ORIENTED_EDGE ( 'NONE', *, *, #11842, .F. ) ;
#3269=FACE_OUTER_BOUND ( 'NONE', #11103, .T. ) ;
#3273=ORIENTED_EDGE ( 'NONE', *, *, #6591, .T. ) ;
#3276=FACE_OUTER_BOUND ( 'NONE', #2176, .T. ) ;
#3277=ORIENTED_EDGE ( 'NONE', *, *, #6383, .F. ) ;
#3280=EDGE_LOOP ( 'NONE', ( #17138, #15660, #19587 ) ) ;
#3283=EDGE_CURVE ( 'NONE', #10155, #10316, #18530, .T. ) ;
#3285=AXIS2_PLACEMENT_3D ( 'NONE', #3463, #5108, #15847 ) ;
#3287=ORIENTED_EDGE ( 'NONE', *, *, #9603, .F. ) ;
#3288=CARTESIAN_POINT ( 'NONE',  ( -53.86996498385652643, -28.06584155524119595, 283.5832628385307999 ) ) ;
#3289=PRODUCT_DEFINITION_FORMATION_WITH_SPECIFIED_SOURCE ( 'ANY', '', #1474, .NOT_KNOWN. ) ;
#3290=DIRECTION ( 'NONE',  ( 0.000000000000000000, 0.000000000000000000, 1.000000000000000000 ) ) ;
#3292=VECTOR ( 'NONE', #2804, 1000.000000000000000 ) ;
#3296=DIRECTION ( 'NONE',  ( -0.9848077530122066880, -0.1736481776669374366, 0.000000000000000000 ) ) ;
#3297=EDGE_CURVE ( 'NONE', #7092, #6348, #9320, .T. ) ;
#3298=EDGE_CURVE ( 'NONE', #18469, #1479, #8572, .T. ) ;
#3300=VERTEX_POINT ( 'NONE', #1446 ) ;
#3305=AXIS2_PLACEMENT_3D ( 'NONE', #11624, #17881, #7320 ) ;
#3306=PLANE ( 'NONE',  #5780 ) ;
#3307=ORIENTED_EDGE ( 'NONE', *, *, #18772, .T. ) ;
#3310=LINE ( 'NONE', #18968, #17848 ) ;
#3314=DIRECTION ( 'NONE',  ( -0.1736481776669340227, 0.9848077530122073542, 0.000000000000000000 ) ) ;
#3315=PLANE ( 'NONE',  #8877 ) ;
#3321=CARTESIAN_POINT ( 'NONE',  ( -78.26059000578311498, 0.8220851292432594937, 112.7772637782949516 ) ) ;
#3323=ORIENTED_EDGE ( 'NONE', *, *, #3755, .F. ) ;
#3324=ORIENTED_EDGE ( 'NONE', *, *, #3886, .T. ) ;
#3328=LINE ( 'NONE', #53, #15952 ) ;
#3329=CARTESIAN_POINT ( 'NONE',  ( 0.000000000000000000, 0.000000000000000000, 283.5832628385307999 ) ) ;
#3331=CARTESIAN_POINT ( 'NONE',  ( 76.92888220842486646, -14.39940464655733976, 112.0427633081292385 ) ) ;
#3334=FACE_OUTER_BOUND ( 'NONE', #5200, .T. ) ;
#3335=VERTEX_POINT ( 'NONE', #1342 ) ;
#3342=ADVANCED_FACE ( 'NONE', ( #1549 ), #13916, .F. ) ;
#3343=DIRECTION ( 'NONE',  ( 0.9848077530122074652, 0.1736481776669340504, 0.000000000000000000 ) ) ;
#3344=AXIS2_PLACEMENT_3D ( 'NONE', #7704, #16924, #12304 ) ;
#3345=VECTOR ( 'NONE', #16519, 1000.000000000000000 ) ;
#3347=CARTESIAN_POINT ( 'NONE',  ( 4.581103194070568208, -3.453261854573344447, 283.5832628385307999 ) ) ;
#3349=CARTESIAN_POINT ( 'NONE',  ( 0.000000000000000000, 0.000000000000000000, 132.4711112102474146 ) ) ;
#3350=ORIENTED_EDGE ( 'NONE', *, *, #18427, .T. ) ;
#3351=AXIS2_PLACEMENT_3D ( 'NONE', #11937, #14923, #910 ) ;
#3354=ORIENTED_EDGE ( 'NONE', *, *, #14924, .F. ) ;
#3355=ADVANCED_FACE ( 'NONE', ( #12381 ), #5854, .T. ) ;
#3356=DIRECTION ( 'NONE',  ( 0.000000000000000000, 0.000000000000000000, 1.000000000000000000 ) ) ;
#3357=CARTESIAN_POINT ( 'NONE',  ( 61.81362617575101837, -11.73417718768070550, 132.4711112102474146 ) ) ;
#3358=EDGE_CURVE ( 'NONE', #7769, #14586, #4617, .T. ) ;
#3359=ADVANCED_FACE ( 'NONE', ( #4204 ), #7371, .F. ) ;
#3360=FACE_OUTER_BOUND ( 'NONE', #14735, .T. ) ;
#3361=AXIS2_PLACEMENT_3D ( 'NONE', #16481, #2268, #14733 ) ;
#3362=AXIS2_PLACEMENT_3D ( 'NONE', #10149, #5644, #8610 ) ;
#3367=CARTESIAN_POINT ( 'NONE',  ( 77.21438937758502163, 12.78021302872874010, 248.9926560891072143 ) ) ;
#3368=ORIENTED_EDGE ( 'NONE', *, *, #12134, .T. ) ;
#3370=ORIENTED_EDGE ( 'NONE', *, *, #11115, .F. ) ;
#3373=ORIENTED_EDGE ( 'NONE', *, *, #157, .T. ) ;
#3374=CARTESIAN_POINT ( 'NONE',  ( 2.629250726500717672, 60.68567895461850270, 283.5832628385307999 ) ) ;
#3379=CARTESIAN_POINT ( 'NONE',  ( -47.66508197439443961, 41.06890862491521688, 293.5832628385307999 ) ) ;
#3382=EDGE_CURVE ( 'NONE', #8156, #7092, #1233, .T. ) ;
#3384=EDGE_CURVE ( 'NONE', #13329, #16043, #4409, .T. ) ;
#3386=DIRECTION ( 'NONE',  ( 1.000000000000000000, 0.000000000000000000, 0.000000000000000000 ) ) ;
#3387=ORIENTED_EDGE ( 'NONE', *, *, #18913, .T. ) ;
#3388=CARTESIAN_POINT ( 'NONE',  ( -59.58067424803613221, 20.21777810286735999, 132.4711112102474146 ) ) ;
#3389=VECTOR ( 'NONE', #2870, 1000.000000000000000 ) ;
#3393=EDGE_LOOP ( 'NONE', ( #12182, #17918, #10781 ) ) ;
#3398=ORIENTED_EDGE ( 'NONE', *, *, #20167, .T. ) ;
#3400=ORIENTED_EDGE ( 'NONE', *, *, #6622, .T. ) ;
#3404=ORIENTED_EDGE ( 'NONE', *, *, #18225, .T. ) ;
#3408=VERTEX_POINT ( 'NONE', #1749 ) ;
#3409=CARTESIAN_POINT ( 'NONE',  ( -37.09555676056967144, 45.48770046196298011, 132.4711112102474146 ) ) ;
#3416=VECTOR ( 'NONE', #3314, 1000.000000000000114 ) ;
#3417=CARTESIAN_POINT ( 'NONE',  ( -12.78021302872797449, 77.21438937758516374, 112.0427633081291816 ) ) ;
#3418=DIRECTION ( 'NONE',  ( -0.000000000000000000, -0.000000000000000000, 1.000000000000000000 ) ) ;
#3421=DIRECTION ( 'NONE',  ( 1.000000000000000000, 0.000000000000000000, 0.000000000000000000 ) ) ;
#3426=ORIENTED_EDGE ( 'NONE', *, *, #8420, .F. ) ;
#3427=LINE ( 'NONE', #1892, #10264 ) ;
#3429=CARTESIAN_POINT ( 'NONE',  ( -59.51523122377251696, 12.14914984460740754, 283.5832628385307999 ) ) ;
#3430=ORIENTED_EDGE ( 'NONE', *, *, #4220, .T. ) ;
#3431=FACE_OUTER_BOUND ( 'NONE', #19180, .T. ) ;
#3432=LINE ( 'NONE', #14578, #18368 ) ;
#3436=CARTESIAN_POINT ( 'NONE',  ( -28.94886449118903826, 53.40063514825088475, 283.5832628385307999 ) ) ;
#3437=ADVANCED_FACE ( 'NONE', ( #7882 ), #10947, .T. ) ;
#3439=CARTESIAN_POINT ( 'NONE',  ( -60.47951622432784546, -49.67518383744813804, 132.4711112102474146 ) ) ;
#3440=AXIS2_PLACEMENT_3D ( 'NONE', #10713, #1315, #12142 ) ;
#3442=ORIENTED_EDGE ( 'NONE', *, *, #6538, .F. ) ;
#3443=ORIENTED_EDGE ( 'NONE', *, *, #8164, .T. ) ;
#3446=CARTESIAN_POINT ( 'NONE',  ( -77.21438937758510690, -12.78021302872823384, 112.0427633081291816 ) ) ;
#3448=CARTESIAN_POINT ( 'NONE',  ( 28.63313560863472063, -51.23821591265105013, 248.9926560891072143 ) ) ;
#3455=DIRECTION ( 'NONE',  ( -0.8479630283625716469, 0.5300553768524345344, 0.000000000000000000 ) ) ;
#3460=EDGE_CURVE ( 'NONE', #720, #19683, #19414, .T. ) ;
#3461=FACE_OUTER_BOUND ( 'NONE', #9802, .T. ) ;
#3462=DIRECTION ( 'NONE',  ( 1.000000000000000000, 0.000000000000000000, 0.000000000000000000 ) ) ;
#3463=CARTESIAN_POINT ( 'NONE',  ( 0.000000000000000000, 0.000000000000000000, 283.5832628385307999 ) ) ;
#3467=DIRECTION ( 'NONE',  ( -0.000000000000000000, -0.000000000000000000, 1.000000000000000000 ) ) ;
#3468=ORIENTED_EDGE ( 'NONE', *, *, #8639, .F. ) ;
#3472=ORIENTED_EDGE ( 'NONE', *, *, #360, .F. ) ;
#3473=VECTOR ( 'NONE', #17804, 1000.000000000000114 ) ;
#3476=PLANE ( 'NONE',  #18757 ) ;
#3481=DIRECTION ( 'NONE',  ( 1.000000000000000000, 0.000000000000000000, 0.000000000000000000 ) ) ;
#3484=LINE ( 'NONE', #2059, #16809 ) ;
#3486=DIRECTION ( 'NONE',  ( 1.000000000000000000, 0.000000000000000000, 0.000000000000000000 ) ) ;
#3489=LINE ( 'NONE', #14534, #9228 ) ;
#3492=VECTOR ( 'NONE', #13412, 1000.000000000000000 ) ;
#3495=VERTEX_POINT ( 'NONE', #4828 ) ;
#3508=DIRECTION ( 'NONE',  ( -0.8660254037844432595, 0.4999999999999919509, 0.000000000000000000 ) ) ;
#3509=VECTOR ( 'NONE', #2855, 1000.000000000000000 ) ;
#3511=DIRECTION ( 'NONE',  ( 0.7660444431189813441, -0.6427876096865353661, 0.000000000000000000 ) ) ;
#3512=AXIS2_PLACEMENT_3D ( 'NONE', #1575, #3114, #10772 ) ;
#3514=CARTESIAN_POINT ( 'NONE',  ( -56.50138340076688337, 22.29928840491054132, 283.5832628385307999 ) ) ;
#3517=LINE ( 'NONE', #243, #19676 ) ;
#3519=EDGE_CURVE ( 'NONE', #19407, #20158, #15767, .T. ) ;
#3520=AXIS2_PLACEMENT_3D ( 'NONE', #9178, #13881, #4170 ) ;
#3521=ADVANCED_FACE ( 'NONE', ( #14532 ), #8188, .F. ) ;
#3526=VECTOR ( 'NONE', #16223, 1000.000000000000000 ) ;
#3527=EDGE_LOOP ( 'NONE', ( #8493, #14502, #18442, #6426 ) ) ;
#3528=CARTESIAN_POINT ( 'NONE',  ( 51.77076963420847733, -31.77187437101486367, 293.5832628385307999 ) ) ;
#3529=CARTESIAN_POINT ( 'NONE',  ( 58.69016442926523069, -0.8220851292429179891, 248.9926560891072143 ) ) ;
#3530=DIRECTION ( 'NONE',  ( -0.000000000000000000, -0.000000000000000000, 1.000000000000000000 ) ) ;
#3533=EDGE_CURVE ( 'NONE', #8624, #10590, #5136, .T. ) ;
#3534=EDGE_CURVE ( 'NONE', #20066, #7454, #8288, .T. ) ;
#3535=DIRECTION ( 'NONE',  ( -0.000000000000000000, -0.000000000000000000, 1.000000000000000000 ) ) ;
#3536=CARTESIAN_POINT ( 'NONE',  ( 7.948937137877743808, -60.22232964560488000, 293.5832628385307999 ) ) ;
#3539=VECTOR ( 'NONE', #3530, 1000.000000000000000 ) ;
#3542=CARTESIAN_POINT ( 'NONE',  ( -59.06449708980197499, -51.36153797460887915, 110.7293897666001214 ) ) ;
#3543=ORIENTED_EDGE ( 'NONE', *, *, #9643, .T. ) ;
#3545=VERTEX_POINT ( 'NONE', #19249 ) ;
#3546=ADVANCED_FACE ( 'NONE', ( #2453 ), #11746, .F. ) ;
#3549=VERTEX_POINT ( 'NONE', #2264 ) ;
#3551=VECTOR ( 'NONE', #19288, 1000.000000000000000 ) ;
#3553=CARTESIAN_POINT ( 'NONE',  ( 0.000000000000000000, 0.000000000000000000, 293.5832628385307999 ) ) ;
#3555=LINE ( 'NONE', #9786, #16474 ) ;
#3556=LINE ( 'NONE', #8047, #13965 ) ;
#3557=ORIENTED_EDGE ( 'NONE', *, *, #2423, .F. ) ;
#3559=DIRECTION ( 'NONE',  ( 0.3747554100459959958, 0.9271237148521535021, 0.000000000000000000 ) ) ;
#3562=DIRECTION ( 'NONE',  ( 0.000000000000000000, 0.000000000000000000, -1.000000000000000000 ) ) ;
#3563=FACE_BOUND ( 'NONE', #12463, .T. ) ;
#3571=AXIS2_PLACEMENT_3D ( 'NONE', #13147, #16445, #876 ) ;
#3572=CARTESIAN_POINT ( 'NONE',  ( 8.939227532413712041, -60.08331549348429235, 293.5832628385307999 ) ) ;
#3574=ORIENTED_EDGE ( 'NONE', *, *, #4802, .T. ) ;
#3576=ORIENTED_EDGE ( 'NONE', *, *, #5014, .F. ) ;
#3581=DIRECTION ( 'NONE',  ( -0.9781142164131917394, 0.2080686897406911207, 0.000000000000000000 ) ) ;
#3582=VECTOR ( 'NONE', #6478, 1000.000000000000227 ) ;
#3584=LINE ( 'NONE', #8075, #3957 ) ;
#3586=LINE ( 'NONE', #14626, #8524 ) ;
#3588=VERTEX_POINT ( 'NONE', #6861 ) ;
#3591=CARTESIAN_POINT ( 'NONE',  ( 0.000000000000000000, 0.000000000000000000, 293.5832628385307999 ) ) ;
#3597=ORIENTED_EDGE ( 'NONE', *, *, #4601, .F. ) ;
#3599=EDGE_LOOP ( 'NONE', ( #169, #404, #13090, #7161 ) ) ;
#3602=EDGE_CURVE ( 'NONE', #2811, #14900, #16572, .T. ) ;
#3604=VERTEX_POINT ( 'NONE', #5234 ) ;
#3605=CARTESIAN_POINT ( 'NONE',  ( 45.84586732611860782, -36.66871011346395193, 132.4711112102474146 ) ) ;
#3608=ORIENTED_EDGE ( 'NONE', *, *, #11479, .T. ) ;
#3611=AXIS2_PLACEMENT_3D ( 'NONE', #13397, #8309, #2285 ) ;
#3615=DIRECTION ( 'NONE',  ( -0.000000000000000000, -0.000000000000000000, 1.000000000000000000 ) ) ;
#3616=EDGE_CURVE ( 'NONE', #8266, #8936, #9928, .T. ) ;
#3621=EDGE_CURVE ( 'NONE', #13255, #2196, #16176, .T. ) ;
#3624=ORIENTED_EDGE ( 'NONE', *, *, #3298, .T. ) ;
#3625=AXIS2_PLACEMENT_3D ( 'NONE', #3972, #5131, #11355 ) ;
#3627=ADVANCED_FACE ( 'NONE', ( #7164 ), #14631, .T. ) ;
#3628=ORIENTED_EDGE ( 'NONE', *, *, #8222, .T. ) ;
#3629=CARTESIAN_POINT ( 'NONE',  ( -79.75827554147308263, 0.000000000000000000, 269.6944534026102360 ) ) ;
#3630=CARTESIAN_POINT ( 'NONE',  ( 53.86996498385652643, 28.06584155524120305, 283.5832628385307999 ) ) ;
#3631=CARTESIAN_POINT ( 'NONE',  ( -67.36461649554505016, 39.84224160888970800, 132.4711112102474146 ) ) ;
#3635=CARTESIAN_POINT ( 'NONE',  ( -53.86996498385652643, -28.06584155524119595, 293.5832628385307999 ) ) ;
#3636=DIRECTION ( 'NONE',  ( 1.000000000000000000, 0.000000000000000000, -0.000000000000000000 ) ) ;
#3637=EDGE_CURVE ( 'NONE', #7218, #11048, #19342, .T. ) ;
#3644=ORIENTED_EDGE ( 'NONE', *, *, #19854, .T. ) ;
#3646=EDGE_LOOP ( 'NONE', ( #4892, #9590, #6375, #13046 ) ) ;
#3647=ORIENTED_EDGE ( 'NONE', *, *, #20232, .T. ) ;
#3648=CARTESIAN_POINT ( 'NONE',  ( 53.86996498385654064, 28.06584155524121016, 293.5832628385307999 ) ) ;
#3650=ORIENTED_EDGE ( 'NONE', *, *, #9118, .F. ) ;
#3651=CARTESIAN_POINT ( 'NONE',  ( -37.93579148621510200, -68.46530598706787885, 132.4711112102474146 ) ) ;
#3652=CARTESIAN_POINT ( 'NONE',  ( -59.42266395395758849, 50.93469132750324491, 132.4711112102474146 ) ) ;
#3653=DIRECTION ( 'NONE',  ( -0.4693298356057531429, 0.8830229359480288309, 0.000000000000000000 ) ) ;
#3654=FACE_OUTER_BOUND ( 'NONE', #2393, .T. ) ;
#3657=CARTESIAN_POINT ( 'NONE',  ( 0.000000000000000000, 0.000000000000000000, 0.000000000000000000 ) ) ;
#3658=EDGE_LOOP ( 'NONE', ( #18419, #14498, #16680, #15748 ) ) ;
#3660=FACE_OUTER_BOUND ( 'NONE', #8884, .T. ) ;
#3661=ADVANCED_FACE ( 'NONE', ( #20134 ), #13476, .F. ) ;
#3662=CARTESIAN_POINT ( 'NONE',  ( 0.000000000000000000, 0.000000000000000000, 248.9926560891072143 ) ) ;
#3663=EDGE_CURVE ( 'NONE', #10563, #108, #8879, .T. ) ;
#3666=PLANE ( 'NONE',  #8894 ) ;
#3671=AXIS2_PLACEMENT_3D ( 'NONE', #15794, #3615, #6490 ) ;
#3675=ORIENTED_EDGE ( 'NONE', *, *, #15885, .T. ) ;
#3676=CARTESIAN_POINT ( 'NONE',  ( 9.401191644521611934, 61.25984398917705676, 248.9926560891072143 ) ) ;
#3678=CARTESIAN_POINT ( 'NONE',  ( 0.000000000000000000, 0.000000000000000000, 293.5832628385307999 ) ) ;
#3681=CARTESIAN_POINT ( 'NONE',  ( 25.47058595421554372, 74.01264520835162841, 132.4711112102474146 ) ) ;
#3683=AXIS2_PLACEMENT_3D ( 'NONE', #3686, #17908, #2352 ) ;
#3685=DIRECTION ( 'NONE',  ( -0.000000000000000000, -0.000000000000000000, 1.000000000000000000 ) ) ;
#3686=CARTESIAN_POINT ( 'NONE',  ( 0.000000000000000000, 0.000000000000000000, 132.4711112102474146 ) ) ;
#3687=DIRECTION ( 'NONE',  ( 0.000000000000000000, 0.000000000000000000, 1.000000000000000000 ) ) ;
#3691=ORIENTED_EDGE ( 'NONE', *, *, #12193, .F. ) ;
#3694=VERTEX_POINT ( 'NONE', #10819 ) ;
#3696=ORIENTED_EDGE ( 'NONE', *, *, #6418, .F. ) ;
#3703=AXIS2_PLACEMENT_3D ( 'NONE', #3446, #3343, #10801 ) ;
#3704=CARTESIAN_POINT ( 'NONE',  ( 5.590028426173794251, 1.289614712049196976, 293.5832628385307999 ) ) ;
#3713=CYLINDRICAL_SURFACE ( 'NONE', #13550, 62.91752772691707207 ) ;
#3715=ORIENTED_EDGE ( 'NONE', *, *, #3155, .T. ) ;
#3716=DIRECTION ( 'NONE',  ( 1.000000000000000000, 0.000000000000000000, 0.000000000000000000 ) ) ;
#3717=VECTOR ( 'NONE', #14763, 1000.000000000000000 ) ;
#3720=VERTEX_POINT ( 'NONE', #13578 ) ;
#3722=ADVANCED_FACE ( 'NONE', ( #18304 ), #4282, .F. ) ;
#3725=VECTOR ( 'NONE', #12397, 1000.000000000000000 ) ;
#3726=DIRECTION ( 'NONE',  ( 1.000000000000000000, 0.000000000000000000, 0.000000000000000000 ) ) ;
#3730=CARTESIAN_POINT ( 'NONE',  ( 77.21438937758500742, 12.78021302872875431, 132.4711112102474146 ) ) ;
#3736=ORIENTED_EDGE ( 'NONE', *, *, #3533, .F. ) ;
#3737=EDGE_LOOP ( 'NONE', ( #13111, #1035, #4240, #17971 ) ) ;
#3739=ORIENTED_EDGE ( 'NONE', *, *, #5014, .T. ) ;
#3741=VERTEX_POINT ( 'NONE', #11230 ) ;
#3743=FACE_OUTER_BOUND ( 'NONE', #2277, .T. ) ;
#3744=LINE ( 'NONE', #8451, #5686 ) ;
#3746=ORIENTED_EDGE ( 'NONE', *, *, #12878, .F. ) ;
#3748=DIRECTION ( 'NONE',  ( -0.6155349844899689060, 0.7881095627315620744, 0.000000000000000000 ) ) ;
#3750=ORIENTED_EDGE ( 'NONE', *, *, #17136, .T. ) ;
#3752=CARTESIAN_POINT ( 'NONE',  ( 30.74413178637190924, -54.89456854707551514, 248.9926560891072143 ) ) ;
#3754=LINE ( 'NONE', #16248, #5914 ) ;
#3755=EDGE_CURVE ( 'NONE', #14163, #14818, #13995, .T. ) ;
#3758=FACE_OUTER_BOUND ( 'NONE', #9626, .T. ) ;
#3761=ORIENTED_EDGE ( 'NONE', *, *, #3131, .T. ) ;
#3762=AXIS2_PLACEMENT_3D ( 'NONE', #4714, #9414, #1646 ) ;
#3763=ORIENTED_EDGE ( 'NONE', *, *, #11892, .T. ) ;
#3765=ORIENTED_EDGE ( 'NONE', *, *, #294, .T. ) ;
#3766=ADVANCED_FACE ( 'NONE', ( #7959 ), #6642, .F. ) ;
#3769=PLANE ( 'NONE',  #14825 ) ;
#3773=VERTEX_POINT ( 'NONE', #10925 ) ;
#3774=DIRECTION ( 'NONE',  ( 0.2080686897406943681, 0.9781142164131909622, 0.000000000000000000 ) ) ;
#3777=PLANE ( 'NONE',  #19615 ) ;
#3778=DIRECTION ( 'NONE',  ( 0.4693298356057531984, -0.8830229359480288309, 0.000000000000000000 ) ) ;
#3779=ORIENTED_EDGE ( 'NONE', *, *, #5127, .T. ) ;
#3783=DIRECTION ( 'NONE',  ( 0.8660254037844380415, 0.5000000000000009992, 0.000000000000000000 ) ) ;
#3786=CARTESIAN_POINT ( 'NONE',  ( 0.000000000000000000, 0.000000000000000000, 132.4711112102474146 ) ) ;
#3789=AXIS2_PLACEMENT_3D ( 'NONE', #20182, #6075, #2693 ) ;
#3790=VERTEX_POINT ( 'NONE', #1934 ) ;
#3791=EDGE_LOOP ( 'NONE', ( #17768, #10295, #4662, #652 ) ) ;
#3793=EDGE_CURVE ( 'NONE', #1302, #3741, #4578, .T. ) ;
#3794=ORIENTED_EDGE ( 'NONE', *, *, #2779, .T. ) ;
#3795=AXIS2_PLACEMENT_3D ( 'NONE', #14091, #5814, #9688 ) ;
#3796=DIRECTION ( 'NONE',  ( 1.000000000000000000, 0.000000000000000000, 0.000000000000000000 ) ) ;
#3803=VECTOR ( 'NONE', #4587, 1000.000000000000227 ) ;
#3808=DIRECTION ( 'NONE',  ( -0.9848077530122085754, 0.1736481776669273336, 0.000000000000000000 ) ) ;
#3813=DIRECTION ( 'NONE',  ( -0.1390141521205912334, 0.9902903945359629034, 0.000000000000000000 ) ) ;
#3814=CARTESIAN_POINT ( 'NONE',  ( -56.50138340076688337, 22.29928840491054487, 293.5832628385307999 ) ) ;
#3815=AXIS2_PLACEMENT_3D ( 'NONE', #14069, #17047, #19901 ) ;
#3819=DIRECTION ( 'NONE',  ( 0.7071067811865472397, 0.000000000000000000, 0.7071067811865479058 ) ) ;
#3823=CARTESIAN_POINT ( 'NONE',  ( -78.26059000578311498, -1.379293853802032732, 248.9926560891072143 ) ) ;
#3824=DIRECTION ( 'NONE',  ( 1.000000000000000000, 0.000000000000000000, -0.000000000000000000 ) ) ;
#3830=DIRECTION ( 'NONE',  ( -0.9902903945359630145, -0.1390141521205912334, 0.000000000000000000 ) ) ;
#3831=VERTEX_POINT ( 'NONE', #11338 ) ;
#3836=EDGE_LOOP ( 'NONE', ( #20021, #13092, #3889, #2591 ) ) ;
#3838=FACE_OUTER_BOUND ( 'NONE', #8072, .T. ) ;
#3840=EDGE_CURVE ( 'NONE', #3915, #6246, #17184, .T. ) ;
#3841=CARTESIAN_POINT ( 'NONE',  ( -20.69304990905115815, 6.063840362151032615, 248.9926560891072143 ) ) ;
#3842=LINE ( 'NONE', #19498, #19724 ) ;
#3843=FACE_OUTER_BOUND ( 'NONE', #10309, .T. ) ;
#3851=FACE_OUTER_BOUND ( 'NONE', #10208, .T. ) ;
#3854=DIRECTION ( 'NONE',  ( 0.000000000000000000, 0.000000000000000000, 1.000000000000000000 ) ) ;
#3856=EDGE_CURVE ( 'NONE', #11985, #15095, #12559, .T. ) ;
#3861=EDGE_CURVE ( 'NONE', #19610, #6772, #11026, .T. ) ;
#3864=ORIENTED_EDGE ( 'NONE', *, *, #5035, .T. ) ;
#3866=ORIENTED_EDGE ( 'NONE', *, *, #15885, .F. ) ;
#3867=CARTESIAN_POINT ( 'NONE',  ( -4.811834253409058348, -3.123743752084112035, 293.5832628385307999 ) ) ;
#3868=CIRCLE ( 'NONE', #15296, 60.74260934110282051 ) ;
#3871=DIRECTION ( 'NONE',  ( 0.1736481776669172583, 0.9848077530122103518, 0.000000000000000000 ) ) ;
#3873=LINE ( 'NONE', #8575, #13558 ) ;
#3876=DIRECTION ( 'NONE',  ( 0.000000000000000000, 0.000000000000000000, 1.000000000000000000 ) ) ;
#3884=DIRECTION ( 'NONE',  ( -0.3747554100459928317, -0.9271237148521548344, 0.000000000000000000 ) ) ;
#3886=EDGE_CURVE ( 'NONE', #6696, #10983, #19781, .T. ) ;
#3889=ORIENTED_EDGE ( 'NONE', *, *, #2310, .T. ) ;
#3891=DIRECTION ( 'NONE',  ( 1.000000000000000000, 0.000000000000000000, 0.000000000000000000 ) ) ;
#3893=ORIENTED_EDGE ( 'NONE', *, *, #1097, .T. ) ;
#3894=ORIENTED_EDGE ( 'NONE', *, *, #9012, .F. ) ;
#3898=DIRECTION ( 'NONE',  ( 0.000000000000000000, 0.000000000000000000, 1.000000000000000000 ) ) ;
#3903=FACE_OUTER_BOUND ( 'NONE', #11630, .T. ) ;
#3904=CARTESIAN_POINT ( 'NONE',  ( -1.379293853801755176, 62.90240729679781850, 293.5832628385307999 ) ) ;
#3907=CARTESIAN_POINT ( 'NONE',  ( 0.7000608949449850238, 5.693982670708919613, 283.5832628385307999 ) ) ;
#3910=VECTOR ( 'NONE', #15811, 1000.000000000000000 ) ;
#3913=DIRECTION ( 'NONE',  ( 1.000000000000000000, 0.000000000000000000, 0.000000000000000000 ) ) ;
#3914=ADVANCED_FACE ( 'NONE', ( #17786 ), #3666, .T. ) ;
#3915=VERTEX_POINT ( 'NONE', #9902 ) ;
#3916=ORIENTED_EDGE ( 'NONE', *, *, #7162, .T. ) ;
#3918=ORIENTED_EDGE ( 'NONE', *, *, #19767, .F. ) ;
#3921=FACE_OUTER_BOUND ( 'NONE', #7832, .T. ) ;
#3922=LINE ( 'NONE', #3631, #6822 ) ;
#3929=DIRECTION ( 'NONE',  ( -0.000000000000000000, -0.000000000000000000, 1.000000000000000000 ) ) ;
#3931=ORIENTED_EDGE ( 'NONE', *, *, #15757, .T. ) ;
#3932=VECTOR ( 'NONE', #13276, 1000.000000000000000 ) ;
#3935=VERTEX_POINT ( 'NONE', #11993 ) ;
#3936=ORIENTED_EDGE ( 'NONE', *, *, #3382, .T. ) ;
#3940=VECTOR ( 'NONE', #18791, 1000.000000000000000 ) ;
#3941=PLANE ( 'NONE',  #5375 ) ;
#3942=DIRECTION ( 'NONE',  ( 1.000000000000000000, 0.000000000000000000, 0.000000000000000000 ) ) ;
#3943=EDGE_LOOP ( 'NONE', ( #16570, #18568, #12997, #19890 ) ) ;
#3946=CARTESIAN_POINT ( 'NONE',  ( 0.000000000000000000, 0.000000000000000000, 293.5832628385307999 ) ) ;
#3947=ORIENTED_EDGE ( 'NONE', *, *, #14850, .F. ) ;
#3948=CARTESIAN_POINT ( 'NONE',  ( 9.381844291199747943, -57.94128254008187184, 248.9926560891072143 ) ) ;
#3950=LINE ( 'NONE', #8657, #17627 ) ;
#3951=DIRECTION ( 'NONE',  ( -0.8660254037844432595, 0.4999999999999919509, 0.000000000000000000 ) ) ;
#3955=ORIENTED_EDGE ( 'NONE', *, *, #1276, .F. ) ;
#3956=EDGE_CURVE ( 'NONE', #6905, #2638, #16149, .T. ) ;
#3957=VECTOR ( 'NONE', #202, 999.9999999999998863 ) ;
#3965=DIRECTION ( 'NONE',  ( 1.000000000000000000, 0.000000000000000000, 0.000000000000000000 ) ) ;
#3968=EDGE_CURVE ( 'NONE', #9705, #10158, #3988, .T. ) ;
#3969=ORIENTED_EDGE ( 'NONE', *, *, #3602, .T. ) ;
#3972=CARTESIAN_POINT ( 'NONE',  ( 0.000000000000000000, 0.000000000000000000, 83.57543755549745867 ) ) ;
#3974=ORIENTED_EDGE ( 'NONE', *, *, #10634, .F. ) ;
#3975=VECTOR ( 'NONE', #17755, 1000.000000000000000 ) ;
#3976=DIRECTION ( 'NONE',  ( 0.9781142164131917394, -0.2080686897406911207, 0.000000000000000000 ) ) ;
#3980=EDGE_CURVE ( 'NONE', #2942, #6926, #589, .T. ) ;
#3984=ORIENTED_EDGE ( 'NONE', *, *, #11842, .T. ) ;
#3985=LINE ( 'NONE', #4396, #16329 ) ;
#3986=EDGE_CURVE ( 'NONE', #7913, #1086, #8362, .T. ) ;
#3987=DIRECTION ( 'NONE',  ( 0.000000000000000000, 0.000000000000000000, 1.000000000000000000 ) ) ;
#3988=CIRCLE ( 'NONE', #5320, 62.91752772691707207 ) ;
#3989=ORIENTED_EDGE ( 'NONE', *, *, #19494, .T. ) ;
#3990=CIRCLE ( 'NONE', #6625, 62.91752772691707207 ) ;
#3994=EDGE_CURVE ( 'NONE', #15308, #11944, #13635, .T. ) ;
#3995=VECTOR ( 'NONE', #10533, 1000.000000000000000 ) ;
#3999=FACE_OUTER_BOUND ( 'NONE', #1297, .T. ) ;
#4001=CARTESIAN_POINT ( 'NONE',  ( -1.289614712049157230, 5.590028426173801357, 293.5832628385307999 ) ) ;
#4002=CARTESIAN_POINT ( 'NONE',  ( -22.28973221005119854, -58.83691981461626597, 248.9926560891072143 ) ) ;
#4003=ORIENTED_EDGE ( 'NONE', *, *, #8639, .T. ) ;
#4008=VECTOR ( 'NONE', #576, 999.9999999999998863 ) ;
#4011=VECTOR ( 'NONE', #15006, 1000.000000000000114 ) ;
#4012=ORIENTED_EDGE ( 'NONE', *, *, #1615, .F. ) ;
#4018=EDGE_CURVE ( 'NONE', #14124, #3199, #4439, .T. ) ;
#4020=AXIS2_PLACEMENT_3D ( 'NONE', #4810, #7861, #9507 ) ;
#4021=DIRECTION ( 'NONE',  ( -0.000000000000000000, -0.000000000000000000, 1.000000000000000000 ) ) ;
#4022=VECTOR ( 'NONE', #5055, 1000.000000000000000 ) ;
#4027=CARTESIAN_POINT ( 'NONE',  ( 22.28973221005080774, 58.83691981461640097, 293.5832628385307999 ) ) ;
#4034=VECTOR ( 'NONE', #8893, 1000.000000000000000 ) ;
#4035=ORIENTED_EDGE ( 'NONE', *, *, #18390, .T. ) ;
#4037=ORIENTED_EDGE ( 'NONE', *, *, #7146, .F. ) ;
#4038=VERTEX_POINT ( 'NONE', #1269 ) ;
#4042=CARTESIAN_POINT ( 'NONE',  ( -11.00103590902911499, -57.65577537092155325, 132.4711112102474146 ) ) ;
#4051=CARTESIAN_POINT ( 'NONE',  ( 0.000000000000000000, 0.000000000000000000, 283.5832628385307999 ) ) ;
#4052=LINE ( 'NONE', #15089, #7479 ) ;
#4053=DIRECTION ( 'NONE',  ( 0.000000000000000000, 0.000000000000000000, 1.000000000000000000 ) ) ;
#4054=LINE ( 'NONE', #12224, #11364 ) ;
#4055=CARTESIAN_POINT ( 'NONE',  ( 36.99387960884163817, -48.17797692984175484, 283.5832628385307999 ) ) ;
#4059=EDGE_LOOP ( 'NONE', ( #14370, #6915 ) ) ;
#4061=CARTESIAN_POINT ( 'NONE',  ( -19.23614321207234923, 57.61627707419557254, 293.5832628385307999 ) ) ;
#4063=EDGE_LOOP ( 'NONE', ( #7211, #1058, #12343 ) ) ;
#4068=EDGE_CURVE ( 'NONE', #7735, #7403, #1379, .T. ) ;
#4072=CARTESIAN_POINT ( 'NONE',  ( 0.000000000000000000, 0.000000000000000000, 283.5832628385307999 ) ) ;
#4074=ORIENTED_EDGE ( 'NONE', *, *, #5640, .F. ) ;
#4077=AXIS2_PLACEMENT_3D ( 'NONE', #5609, #16753, #13367 ) ;
#4078=FACE_OUTER_BOUND ( 'NONE', #988, .T. ) ;
#4079=ORIENTED_EDGE ( 'NONE', *, *, #547, .T. ) ;
#4080=EDGE_CURVE ( 'NONE', #4164, #13913, #14132, .T. ) ;
#4081=DIRECTION ( 'NONE',  ( 0.7430374143461900838, -0.6692498792541753394, 0.000000000000000000 ) ) ;
#4083=ORIENTED_EDGE ( 'NONE', *, *, #13614, .F. ) ;
#4086=ORIENTED_EDGE ( 'NONE', *, *, #1535, .T. ) ;
#4088=DIRECTION ( 'NONE',  ( 0.000000000000000000, 0.000000000000000000, -1.000000000000000000 ) ) ;
#4090=AXIS2_PLACEMENT_3D ( 'NONE', #17899, #17997, #19434 ) ;
#4094=EDGE_CURVE ( 'NONE', #9575, #14124, #9349, .T. ) ;
#4095=DIRECTION ( 'NONE',  ( 0.9902903945359623483, 0.1390141521205945918, 0.000000000000000000 ) ) ;
#4096=PLANE ( 'NONE',  #5596 ) ;
#4097=DIRECTION ( 'NONE',  ( -0.4999999999999919509, -0.8660254037844432595, 0.000000000000000000 ) ) ;
#4100=DIRECTION ( 'NONE',  ( -0.7430374143461878633, 0.6692498792541777819, 0.000000000000000000 ) ) ;
#4103=VERTEX_POINT ( 'NONE', #9247 ) ;
#4109=EDGE_CURVE ( 'NONE', #18597, #4682, #1475, .T. ) ;
#4111=ORIENTED_EDGE ( 'NONE', *, *, #18557, .T. ) ;
#4112=CARTESIAN_POINT ( 'NONE',  ( 22.28973221005081129, 58.83691981461641518, 132.4711112102474146 ) ) ;
#4113=ORIENTED_EDGE ( 'NONE', *, *, #5371, .F. ) ;
#4115=LINE ( 'NONE', #4316, #17284 ) ;
#4117=EDGE_CURVE ( 'NONE', #18256, #7769, #6196, .T. ) ;
#4119=DIRECTION ( 'NONE',  ( -0.9848077530122091305, 0.1736481776669241417, 0.000000000000000000 ) ) ;
#4127=CARTESIAN_POINT ( 'NONE',  ( 0.000000000000000000, 0.000000000000000000, 293.5832628385307999 ) ) ;
#4128=DIRECTION ( 'NONE',  ( -0.000000000000000000, -0.000000000000000000, 1.000000000000000000 ) ) ;
#4130=ADVANCED_FACE ( 'NONE', ( #1372 ), #6296, .F. ) ;
#4132=EDGE_CURVE ( 'NONE', #18385, #10900, #19371, .T. ) ;
#4133=ADVANCED_FACE ( 'NONE', ( #5983 ), #20086, .T. ) ;
#4135=EDGE_LOOP ( 'NONE', ( #14885, #12306, #9777 ) ) ;
#4136=AXIS2_PLACEMENT_3D ( 'NONE', #1865, #6684, #8200 ) ;
#4138=ORIENTED_EDGE ( 'NONE', *, *, #11663, .T. ) ;
#4139=VERTEX_POINT ( 'NONE', #11081 ) ;
#4141=ORIENTED_EDGE ( 'NONE', *, *, #14238, .T. ) ;
#4144=CARTESIAN_POINT ( 'NONE',  ( 0.000000000000000000, 0.000000000000000000, 283.5832628385307999 ) ) ;
#4145=ORIENTED_EDGE ( 'NONE', *, *, #7409, .F. ) ;
#4147=CARTESIAN_POINT ( 'NONE',  ( 0.000000000000000000, 0.000000000000000000, 293.5832628385307999 ) ) ;
#4150=DIRECTION ( 'NONE',  ( -0.3747554100459928317, -0.9271237148521548344, 0.000000000000000000 ) ) ;
#4152=DIRECTION ( 'NONE',  ( -0.000000000000000000, -0.000000000000000000, 1.000000000000000000 ) ) ;
#4154=EDGE_CURVE ( 'NONE', #6500, #12180, #8113, .T. ) ;
#4155=EDGE_CURVE ( 'NONE', #10080, #3915, #10520, .T. ) ;
#4158=ORIENTED_EDGE ( 'NONE', *, *, #9916, .F. ) ;
#4160=ORIENTED_EDGE ( 'NONE', *, *, #11040, .T. ) ;
#4163=CARTESIAN_POINT ( 'NONE',  ( -65.74260934110282051, 0.000000000000000000, 293.5832628385307999 ) ) ;
#4164=VERTEX_POINT ( 'NONE', #14565 ) ;
#4167=DIRECTION ( 'NONE',  ( -0.8660254037844415942, 0.4999999999999950040, 0.000000000000000000 ) ) ;
#4170=DIRECTION ( 'NONE',  ( 1.000000000000000000, 0.000000000000000000, 0.000000000000000000 ) ) ;
#4171=DIRECTION ( 'NONE',  ( -0.000000000000000000, 1.000000000000000000, 0.000000000000000000 ) ) ;
#4175=DIRECTION ( 'NONE',  ( 0.6427876096865379196, 0.7660444431189792347, 0.000000000000000000 ) ) ;
#4176=FACE_OUTER_BOUND ( 'NONE', #8033, .T. ) ;
#4178=DIRECTION ( 'NONE',  ( 0.1736481776669374366, -0.9848077530122066880, 0.000000000000000000 ) ) ;
#4181=AXIS2_PLACEMENT_3D ( 'NONE', #16932, #15288, #2922 ) ;
#4184=CIRCLE ( 'NONE', #927, 60.74260934110282051 ) ;
#4185=DIRECTION ( 'NONE',  ( 0.000000000000000000, 0.000000000000000000, 1.000000000000000000 ) ) ;
#4186=DIRECTION ( 'NONE',  ( -1.000000000000000000, 0.000000000000000000, -0.000000000000000000 ) ) ;
#4188=VERTEX_POINT ( 'NONE', #554 ) ;
#4189=CARTESIAN_POINT ( 'NONE',  ( 79.75827554147308263, 0.000000000000000000, 293.5832628385307999 ) ) ;
#4190=ORIENTED_EDGE ( 'NONE', *, *, #14549, .F. ) ;
#4194=VECTOR ( 'NONE', #3871, 1000.000000000000000 ) ;
#4195=CYLINDRICAL_SURFACE ( 'NONE', #8994, 60.74260934110282051 ) ;
#4197=CIRCLE ( 'NONE', #925, 17.50000000000001066 ) ;
#4198=AXIS2_PLACEMENT_3D ( 'NONE', #903, #10404, #5613 ) ;
#4204=FACE_OUTER_BOUND ( 'NONE', #10436, .T. ) ;
#4205=DIRECTION ( 'NONE',  ( 0.000000000000000000, 0.000000000000000000, -1.000000000000000000 ) ) ;
#4208=CARTESIAN_POINT ( 'NONE',  ( 58.03804081968166173, -8.833100819207778898, 132.4711112102474146 ) ) ;
#4210=AXIS2_PLACEMENT_3D ( 'NONE', #14405, #7030, #783 ) ;
#4211=AXIS2_PLACEMENT_3D ( 'NONE', #11120, #12448, #8050 ) ;
#4212=EDGE_CURVE ( 'NONE', #15168, #2215, #19279, .T. ) ;
#4213=ORIENTED_EDGE ( 'NONE', *, *, #2607, .F. ) ;
#4214=ORIENTED_EDGE ( 'NONE', *, *, #11535, .T. ) ;
#4215=LINE ( 'NONE', #11321, #3492 ) ;
#4216=VERTEX_POINT ( 'NONE', #17736 ) ;
#4218=CARTESIAN_POINT ( 'NONE',  ( 12.50000000000006750, 0.000000000000000000, 0.000000000000000000 ) ) ;
#4219=CARTESIAN_POINT ( 'NONE',  ( 12.23146955673593794, 77.31114765718498916, 112.0427633081292953 ) ) ;
#4220=EDGE_CURVE ( 'NONE', #6267, #8471, #5633, .T. ) ;
#4222=EDGE_CURVE ( 'NONE', #3408, #1238, #1783, .T. ) ;
#4223=DIRECTION ( 'NONE',  ( 1.000000000000000000, 3.491481338843133355E-15, 0.000000000000000000 ) ) ;
#4226=EDGE_LOOP ( 'NONE', ( #3170, #17495, #18799, #18677 ) ) ;
#4227=EDGE_CURVE ( 'NONE', #15975, #14511, #3517, .T. ) ;
#4228=DIRECTION ( 'NONE',  ( -0.1736481776669374366, 0.9848077530122067991, 0.000000000000000000 ) ) ;
#4230=CARTESIAN_POINT ( 'NONE',  ( 76.83212392882491315, 14.94814811854987191, 248.9926560891072143 ) ) ;
#4232=DIRECTION ( 'NONE',  ( 0.000000000000000000, 0.000000000000000000, 1.000000000000000000 ) ) ;
#4237=EDGE_LOOP ( 'NONE', ( #3576, #1587, #7166 ) ) ;
#4238=ORIENTED_EDGE ( 'NONE', *, *, #1732, .T. ) ;
#4239=EDGE_LOOP ( 'NONE', ( #6061, #14587, #19473, #19974 ) ) ;
#4240=ORIENTED_EDGE ( 'NONE', *, *, #11221, .T. ) ;
#4245=DIRECTION ( 'NONE',  ( -0.000000000000000000, -0.000000000000000000, 1.000000000000000000 ) ) ;
#4246=DIRECTION ( 'NONE',  ( 0.9848077530122073542, 0.1736481776669340227, 0.000000000000000000 ) ) ;
#4248=ORIENTED_EDGE ( 'NONE', *, *, #525, .T. ) ;
#4249=LINE ( 'NONE', #16244, #17291 ) ;
#4253=VECTOR ( 'NONE', #16688, 1000.000000000000000 ) ;
#4254=LINE ( 'NONE', #13658, #13095 ) ;
#4255=CARTESIAN_POINT ( 'NONE',  ( 27.53920554013639688, 73.25972925305639194, 132.4711112102474146 ) ) ;
#4256=LINE ( 'NONE', #15195, #1522 ) ;
#4258=EDGE_CURVE ( 'NONE', #11632, #5887, #16403, .T. ) ;
#4260=ORIENTED_EDGE ( 'NONE', *, *, #14996, .F. ) ;
#4261=ORIENTED_EDGE ( 'NONE', *, *, #5809, .T. ) ;
#4262=CARTESIAN_POINT ( 'NONE',  ( 3.911853314815631588, -4.196299268919051251, 283.5832628385307999 ) ) ;
#4263=AXIS2_PLACEMENT_3D ( 'NONE', #9499, #4404, #11958 ) ;
#4265=VERTEX_POINT ( 'NONE', #17941 ) ;
#4266=VECTOR ( 'NONE', #13471, 1000.000000000000000 ) ;
#4268=CARTESIAN_POINT ( 'NONE',  ( 30.74413178637192701, -54.89456854707552935, 132.4711112102474146 ) ) ;
#4269=EDGE_LOOP ( 'NONE', ( #18479, #4086, #361, #1620 ) ) ;
#4270=EDGE_CURVE ( 'NONE', #2211, #3220, #2383, .T. ) ;
#4271=CARTESIAN_POINT ( 'NONE',  ( 48.72193424476450474, 39.80940113486034448, 293.5832628385307999 ) ) ;
#4272=CARTESIAN_POINT ( 'NONE',  ( -59.39925916207560164, -20.74471755083584412, 132.4711112102474146 ) ) ;
#4273=EDGE_CURVE ( 'NONE', #4648, #5962, #8713, .T. ) ;
#4275=DIRECTION ( 'NONE',  ( -0.9396926207859092051, 0.3420201433256662704, 0.000000000000000000 ) ) ;
#4276=CARTESIAN_POINT ( 'NONE',  ( 32.16802499836741447, 54.07248341783265033, 293.5832628385307999 ) ) ;
#4278=CARTESIAN_POINT ( 'NONE',  ( 57.65577537092158877, -11.00103590902891249, 132.4711112102474146 ) ) ;
#4280=ORIENTED_EDGE ( 'NONE', *, *, #9023, .F. ) ;
#4282=PLANE ( 'NONE',  #17345 ) ;
#4285=EDGE_LOOP ( 'NONE', ( #10270, #13770, #8364, #14184 ) ) ;
#4287=DIRECTION ( 'NONE',  ( 0.000000000000000000, 0.000000000000000000, 1.000000000000000000 ) ) ;
#4288=EDGE_CURVE ( 'NONE', #18107, #5657, #15152, .T. ) ;
#4289=ORIENTED_EDGE ( 'NONE', *, *, #19302, .T. ) ;
#4290=ORIENTED_EDGE ( 'NONE', *, *, #8914, .T. ) ;
#4291=DIRECTION ( 'NONE',  ( 1.000000000000000000, 0.000000000000000000, -0.000000000000000000 ) ) ;
#4292=ORIENTED_EDGE ( 'NONE', *, *, #7908, .T. ) ;
#4293=DIRECTION ( 'NONE',  ( 0.000000000000000000, 0.000000000000000000, 1.000000000000000000 ) ) ;
#4295=EDGE_LOOP ( 'NONE', ( #9904, #2927, #14343, #12946 ) ) ;
#4297=CARTESIAN_POINT ( 'NONE',  ( 0.000000000000000000, 0.000000000000000000, 283.5832628385307999 ) ) ;
#4298=EDGE_CURVE ( 'NONE', #14566, #15008, #12160, .T. ) ;
#4299=LINE ( 'NONE', #9103, #8513 ) ;
#4302=DIRECTION ( 'NONE',  ( -0.000000000000000000, -0.000000000000000000, 1.000000000000000000 ) ) ;
#4304=CARTESIAN_POINT ( 'NONE',  ( -20.84572577951200500, -54.86954475316249358, 248.9926560891072143 ) ) ;
#4305=EDGE_LOOP ( 'NONE', ( #11207, #9441, #19175, #19401 ) ) ;
#4306=DIRECTION ( 'NONE',  ( -0.9781142164131917394, 0.2080686897406911207, 0.000000000000000000 ) ) ;
#4307=LINE ( 'NONE', #9429, #7934 ) ;
#4308=ORIENTED_EDGE ( 'NONE', *, *, #1629, .T. ) ;
#4309=ORIENTED_EDGE ( 'NONE', *, *, #6895, .F. ) ;
#4310=AXIS2_PLACEMENT_3D ( 'NONE', #11501, #10263, #19292 ) ;
#4311=ORIENTED_EDGE ( 'NONE', *, *, #2510, .F. ) ;
#4312=FACE_BOUND ( 'NONE', #10602, .T. ) ;
#4314=LINE ( 'NONE', #8449, #2397 ) ;
#4316=CARTESIAN_POINT ( 'NONE',  ( -12.78021302872797449, 77.21438937758516374, 112.0427633081291816 ) ) ;
#4318=CARTESIAN_POINT ( 'NONE',  ( 0.000000000000000000, 0.000000000000000000, 4.999999999999948486 ) ) ;
#4319=DIRECTION ( 'NONE',  ( -0.6427876096865300370, -0.7660444431189858960, -0.000000000000000000 ) ) ;
#4322=CARTESIAN_POINT ( 'NONE',  ( 28.94886449118905247, -53.40063514825087765, 283.5832628385307999 ) ) ;
#4327=FACE_OUTER_BOUND ( 'NONE', #10521, .T. ) ;
#4330=VERTEX_POINT ( 'NONE', #11865 ) ;
#4334=EDGE_CURVE ( 'NONE', #5779, #17978, #1734, .T. ) ;
#4335=VERTEX_POINT ( 'NONE', #5552 ) ;
#4338=AXIS2_PLACEMENT_3D ( 'NONE', #15728, #1709, #14394 ) ;
#4347=EDGE_CURVE ( 'NONE', #4753, #9432, #18036, .T. ) ;
#4348=VERTEX_POINT ( 'NONE', #3814 ) ;
#4349=CARTESIAN_POINT ( 'NONE',  ( 0.000000000000000000, 0.000000000000000000, 293.5832628385307999 ) ) ;
#4350=CARTESIAN_POINT ( 'NONE',  ( -4.581103194068993467, 3.453261854572371892, 283.5832628385307999 ) ) ;
#4352=LINE ( 'NONE', #10686, #3940 ) ;
#4354=VECTOR ( 'NONE', #9194, 1000.000000000000114 ) ;
#4356=LINE ( 'NONE', #12226, #16879 ) ;
#4357=EDGE_LOOP ( 'NONE', ( #5872, #7950, #2816, #10174 ) ) ;
#4358=ORIENTED_EDGE ( 'NONE', *, *, #14102, .F. ) ;
#4359=EDGE_CURVE ( 'NONE', #1787, #11573, #10059, .T. ) ;
#4360=DIRECTION ( 'NONE',  ( 0.000000000000000000, 0.000000000000000000, 1.000000000000000000 ) ) ;
#4362=VECTOR ( 'NONE', #945, 1000.000000000000227 ) ;
#4365=LINE ( 'NONE', #20014, #758 ) ;
#4366=VECTOR ( 'NONE', #17401, 1000.000000000000000 ) ;
#4369=CARTESIAN_POINT ( 'NONE',  ( -9.381844291199351815, 57.94128254008192158, 132.4711112102474146 ) ) ;
#4375=ORIENTED_EDGE ( 'NONE', *, *, #12727, .F. ) ;
#4377=CARTESIAN_POINT ( 'NONE',  ( 39.80940113486020948, -48.72193424476463974, 132.4711112102474146 ) ) ;
#4381=VECTOR ( 'NONE', #9150, 999.9999999999998863 ) ;
#4383=DIRECTION ( 'NONE',  ( -0.3420201433256630508, -0.9396926207859104263, 0.000000000000000000 ) ) ;
#4385=ORIENTED_EDGE ( 'NONE', *, *, #9464, .F. ) ;
#4386=CARTESIAN_POINT ( 'NONE',  ( -12.50000000000006750, 1.836970198721034716E-15, 0.000000000000000000 ) ) ;
#4388=ORIENTED_EDGE ( 'NONE', *, *, #4505, .T. ) ;
#4391=EDGE_LOOP ( 'NONE', ( #8845, #17238, #6617, #15831 ) ) ;
#4396=CARTESIAN_POINT ( 'NONE',  ( 62.90240729679780429, 1.379293853802413983, 293.5832628385307999 ) ) ;
#4398=ORIENTED_EDGE ( 'NONE', *, *, #15882, .T. ) ;
#4400=DIRECTION ( 'NONE',  ( 0.000000000000000000, -0.000000000000000000, 1.000000000000000000 ) ) ;
#4404=DIRECTION ( 'NONE',  ( -0.9511061040868804550, -0.3088643371590125697, 0.000000000000000000 ) ) ;
#4407=AXIS2_PLACEMENT_3D ( 'NONE', #16970, #7752, #15539 ) ;
#4408=FACE_OUTER_BOUND ( 'NONE', #4239, .T. ) ;
#4409=LINE ( 'NONE', #13710, #9450 ) ;
#4411=EDGE_LOOP ( 'NONE', ( #20148, #1362, #14929, #20163 ) ) ;
#4413=DIRECTION ( 'NONE',  ( 1.000000000000000000, 0.000000000000000000, 0.000000000000000000 ) ) ;
#4415=ORIENTED_EDGE ( 'NONE', *, *, #11994, .F. ) ;
#4417=CIRCLE ( 'NONE', #3118, 60.74260934110282051 ) ;
#4418=ORIENTED_EDGE ( 'NONE', *, *, #11276, .T. ) ;
#4420=FACE_BOUND ( 'NONE', #11253, .T. ) ;
#4422=DIRECTION ( 'NONE',  ( 1.000000000000000000, 0.000000000000000000, 0.000000000000000000 ) ) ;
#4424=LINE ( 'NONE', #8822, #1566 ) ;
#4427=CARTESIAN_POINT ( 'NONE',  ( 60.68567895461851691, -2.629250726500488078, 283.5832628385307999 ) ) ;
#4428=LINE ( 'NONE', #10658, #10390 ) ;
#4430=VERTEX_POINT ( 'NONE', #18537 ) ;
#4435=VECTOR ( 'NONE', #18023, 999.9999999999998863 ) ;
#4439=LINE ( 'NONE', #18674, #6951 ) ;
#4440=ORIENTED_EDGE ( 'NONE', *, *, #11408, .T. ) ;
#4441=AXIS2_PLACEMENT_3D ( 'NONE', #17018, #3005, #19972 ) ;
#4442=ORIENTED_EDGE ( 'NONE', *, *, #8529, .F. ) ;
#4445=LINE ( 'NONE', #9043, #13511 ) ;
#4449=DIRECTION ( 'NONE',  ( 1.000000000000000000, 0.000000000000000000, 0.000000000000000000 ) ) ;
#4453=CARTESIAN_POINT ( 'NONE',  ( -23.22641211976288744, -56.12662799072081299, 283.5832628385307999 ) ) ;
#4454=DIRECTION ( 'NONE',  ( 1.000000000000000000, 0.000000000000000000, 0.000000000000000000 ) ) ;
#4456=AXIS2_PLACEMENT_3D ( 'NONE', #4051, #12014, #11910 ) ;
#4457=VECTOR ( 'NONE', #10856, 1000.000000000000000 ) ;
#4459=DIRECTION ( 'NONE',  ( -0.000000000000000000, -0.000000000000000000, 1.000000000000000000 ) ) ;
#4462=ORIENTED_EDGE ( 'NONE', *, *, #11357, .F. ) ;
#4465=ORIENTED_EDGE ( 'NONE', *, *, #4505, .F. ) ;
#4466=ADVANCED_FACE ( 'NONE', ( #12281 ), #2788, .F. ) ;
#4468=ORIENTED_EDGE ( 'NONE', *, *, #4969, .F. ) ;
#4469=CARTESIAN_POINT ( 'NONE',  ( 54.89456854707540856, 30.74413178637212241, 248.9926560891072143 ) ) ;
#4473=VERTEX_POINT ( 'NONE', #4725 ) ;
#4475=LINE ( 'NONE', #2954, #8780 ) ;
#4477=AXIS2_PLACEMENT_3D ( 'NONE', #18843, #3290, #9525 ) ;
#4481=CARTESIAN_POINT ( 'NONE',  ( 0.000000000000000000, 0.000000000000000000, 293.5832628385307999 ) ) ;
#4483=EDGE_CURVE ( 'NONE', #1866, #1970, #4307, .T. ) ;
#4484=CARTESIAN_POINT ( 'NONE',  ( -22.29928840491073316, -56.50138340076681231, 293.5832628385307999 ) ) ;
#4485=CARTESIAN_POINT ( 'NONE',  ( 11.54977938102087620, -57.55901709132175625, 132.4711112102474146 ) ) ;
#4489=DIRECTION ( 'NONE',  ( -0.7660444431189813441, 0.6427876096865353661, 0.000000000000000000 ) ) ;
#4492=VECTOR ( 'NONE', #6022, 1000.000000000000114 ) ;
#4494=EDGE_CURVE ( 'NONE', #15118, #5313, #19856, .T. ) ;
#4499=CARTESIAN_POINT ( 'NONE',  ( -39.84224160888947353, -67.36461649554519227, 110.9660488491356887 ) ) ;
#4500=ORIENTED_EDGE ( 'NONE', *, *, #10003, .F. ) ;
#4502=CARTESIAN_POINT ( 'NONE',  ( -68.46530598706769410, 37.93579148621533648, 110.9660488491356887 ) ) ;
#4504=CIRCLE ( 'NONE', #17269, 60.74260934110282051 ) ;
#4505=EDGE_CURVE ( 'NONE', #2090, #1965, #20063, .T. ) ;
#4507=CIRCLE ( 'NONE', #20180, 62.91752772691707207 ) ;
#4508=ORIENTED_EDGE ( 'NONE', *, *, #3037, .T. ) ;
#4513=ORIENTED_EDGE ( 'NONE', *, *, #18811, .F. ) ;
#4516=VERTEX_POINT ( 'NONE', #12481 ) ;
#4517=VERTEX_POINT ( 'NONE', #7681 ) ;
#4518=ADVANCED_FACE ( 'NONE', ( #1135 ), #12385, .F. ) ;
#4529=LINE ( 'NONE', #4636, #137 ) ;
#4530=CARTESIAN_POINT ( 'NONE',  ( 0.7000608949449920182, 5.693982670708932936, 293.5832628385307999 ) ) ;
#4532=EDGE_CURVE ( 'NONE', #1086, #195, #7574, .T. ) ;
#4533=FACE_OUTER_BOUND ( 'NONE', #18798, .T. ) ;
#4534=DIRECTION ( 'NONE',  ( 1.000000000000000000, 0.000000000000000000, 0.000000000000000000 ) ) ;
#4535=EDGE_CURVE ( 'NONE', #1924, #3694, #10846, .T. ) ;
#4540=PLANE ( 'NONE',  #3512 ) ;
#4541=AXIS2_PLACEMENT_3D ( 'NONE', #16045, #17688, #16247 ) ;
#4545=VERTEX_POINT ( 'NONE', #18436 ) ;
#4546=DIRECTION ( 'NONE',  ( 1.000000000000000000, 0.000000000000000000, 0.000000000000000000 ) ) ;
#4547=ADVANCED_FACE ( 'NONE', ( #14028 ), #3090, .T. ) ;
#4548=ORIENTED_EDGE ( 'NONE', *, *, #18828, .F. ) ;
#4549=ORIENTED_EDGE ( 'NONE', *, *, #34, .F. ) ;
#4554=CIRCLE ( 'NONE', #19277, 60.74260934110282051 ) ;
#4555=CARTESIAN_POINT ( 'NONE',  ( -12.28122767885804301, 61.70726652483831032, 248.9926560891072143 ) ) ;
#4557=ORIENTED_EDGE ( 'NONE', *, *, #4222, .T. ) ;
#4558=CYLINDRICAL_SURFACE ( 'NONE', #1836, 62.91752772691707207 ) ;
#4559=CARTESIAN_POINT ( 'NONE',  ( 49.67518383744835120, -60.47951622432767493, 248.9926560891072143 ) ) ;
#4565=DIRECTION ( 'NONE',  ( -0.5300553768524375320, -0.8479630283625697595, 0.000000000000000000 ) ) ;
#4567=DIRECTION ( 'NONE',  ( 0.4693298356057564180, -0.8830229359480272766, 0.000000000000000000 ) ) ;
#4569=ORIENTED_EDGE ( 'NONE', *, *, #860, .F. ) ;
#4570=ORIENTED_EDGE ( 'NONE', *, *, #234, .F. ) ;
#4571=EDGE_LOOP ( 'NONE', ( #12099, #18319, #11264, #15458 ) ) ;
#4573=CARTESIAN_POINT ( 'NONE',  ( -28.63313560863435825, 51.23821591265124198, 110.9660488491356887 ) ) ;
#4575=ORIENTED_EDGE ( 'NONE', *, *, #6355, .T. ) ;
#4576=CARTESIAN_POINT ( 'NONE',  ( 68.18670162478805707, 38.41834839689404646, 110.9660488491356887 ) ) ;
#4578=CIRCLE ( 'NONE', #8, 62.91752772691707207 ) ;
#4583=AXIS2_PLACEMENT_3D ( 'NONE', #17201, #12472, #12682 ) ;
#4586=VERTEX_POINT ( 'NONE', #19 ) ;
#4587=DIRECTION ( 'NONE',  ( 0.2080686897406943681, 0.9781142164131909622, 0.000000000000000000 ) ) ;
#4588=DIRECTION ( 'NONE',  ( 1.000000000000000000, 0.000000000000000000, 0.000000000000000000 ) ) ;
#4589=EDGE_CURVE ( 'NONE', #14479, #1, #15446, .T. ) ;
#4591=DIRECTION ( 'NONE',  ( 0.8479630283625716469, -0.5300553768524345344, 0.000000000000000000 ) ) ;
#4594=ORIENTED_EDGE ( 'NONE', *, *, #9383, .T. ) ;
#4596=CARTESIAN_POINT ( 'NONE',  ( -57.94128254008190027, -9.381844291199545438, 132.4711112102474146 ) ) ;
#4598=VECTOR ( 'NONE', #7926, 999.9999999999998863 ) ;
#4599=VERTEX_POINT ( 'NONE', #10642 ) ;
#4600=DIRECTION ( 'NONE',  ( 0.000000000000000000, 0.000000000000000000, 1.000000000000000000 ) ) ;
#4601=EDGE_CURVE ( 'NONE', #1034, #5404, #16897, .T. ) ;
#4602=ORIENTED_EDGE ( 'NONE', *, *, #340, .F. ) ;
#4608=DIRECTION ( 'NONE',  ( -0.9848077530122091305, 0.1736481776669241417, 0.000000000000000000 ) ) ;
#4609=CIRCLE ( 'NONE', #678, 60.74260934110282051 ) ;
#4612=DIRECTION ( 'NONE',  ( 0.7430374143461900838, -0.6692498792541753394, 0.000000000000000000 ) ) ;
#4616=CARTESIAN_POINT ( 'NONE',  ( 0.000000000000000000, 0.000000000000000000, 283.5832628385307999 ) ) ;
#4617=LINE ( 'NONE', #10841, #8778 ) ;
#4621=LINE ( 'NONE', #14027, #12993 ) ;
#4627=EDGE_CURVE ( 'NONE', #13898, #1302, #17521, .T. ) ;
#4632=FACE_BOUND ( 'NONE', #11728, .T. ) ;
#4633=ORIENTED_EDGE ( 'NONE', *, *, #3298, .F. ) ;
#4635=CARTESIAN_POINT ( 'NONE',  ( 28.94983032429829350, -53.40245231972188833, 293.5832628385307999 ) ) ;
#4636=CARTESIAN_POINT ( 'NONE',  ( -5.485913980968301296, 1.678175111358176652, 293.5832628385307999 ) ) ;
#4641=DIRECTION ( 'NONE',  ( 1.000000000000000000, 0.000000000000000000, 0.000000000000000000 ) ) ;
#4642=CARTESIAN_POINT ( 'NONE',  ( 53.87178215532755132, 28.06680738835045119, 293.5832628385307999 ) ) ;
#4643=EDGE_CURVE ( 'NONE', #18107, #8936, #16111, .T. ) ;
#4645=CARTESIAN_POINT ( 'NONE',  ( 44.79940644582654841, -41.02350267428983699, 293.5832628385307999 ) ) ;
#4648=VERTEX_POINT ( 'NONE', #14637 ) ;
#4654=VERTEX_POINT ( 'NONE', #16381 ) ;
#4656=EDGE_CURVE ( 'NONE', #15357, #10563, #9579, .T. ) ;
#4662=ORIENTED_EDGE ( 'NONE', *, *, #11725, .T. ) ;
#4665=LINE ( 'NONE', #15398, #2599 ) ;
#4669=DIRECTION ( 'NONE',  ( 1.000000000000000000, 0.000000000000000000, 0.000000000000000000 ) ) ;
#4672=LINE ( 'NONE', #10894, #4266 ) ;
#4673=DIRECTION ( 'NONE',  ( -0.8479630283625698706, 0.5300553768524376430, 0.000000000000000000 ) ) ;
#4679=VECTOR ( 'NONE', #7584, 1000.000000000000000 ) ;
#4681=EDGE_CURVE ( 'NONE', #14807, #2821, #719, .T. ) ;
#4682=VERTEX_POINT ( 'NONE', #14927 ) ;
#4683=LINE ( 'NONE', #4786, #2079 ) ;
#4684=ORIENTED_EDGE ( 'NONE', *, *, #17902, .F. ) ;
#4685=CARTESIAN_POINT ( 'NONE',  ( -54.86954475316242252, 20.84572577951219330, 248.9926560891072143 ) ) ;
#4686=EDGE_CURVE ( 'NONE', #15800, #3915, #10315, .T. ) ;
#4687=DIRECTION ( 'NONE',  ( 0.000000000000000000, 0.000000000000000000, 1.000000000000000000 ) ) ;
#4688=DIRECTION ( 'NONE',  ( 0.000000000000000000, 0.000000000000000000, 1.000000000000000000 ) ) ;
#4691=ORIENTED_EDGE ( 'NONE', *, *, #18863, .T. ) ;
#4693=CYLINDRICAL_SURFACE ( 'NONE', #10752, 62.91752772691707207 ) ;
#4696=CARTESIAN_POINT ( 'NONE',  ( 53.40245231972179596, 28.94983032429848535, 283.5832628385307999 ) ) ;
#4697=DIRECTION ( 'NONE',  ( -0.000000000000000000, -0.000000000000000000, 1.000000000000000000 ) ) ;
#4698=CARTESIAN_POINT ( 'NONE',  ( -2.629322876227788264, -60.68773558783006905, 283.5832628385307999 ) ) ;
#4702=VERTEX_POINT ( 'NONE', #13280 ) ;
#4703=DIRECTION ( 'NONE',  ( -0.000000000000000000, -0.000000000000000000, 1.000000000000000000 ) ) ;
#4704=AXIS2_PLACEMENT_3D ( 'NONE', #5607, #8376, #995 ) ;
#4707=PLANE ( 'NONE',  #14663 ) ;
#4714=CARTESIAN_POINT ( 'NONE',  ( 0.000000000000000000, 0.000000000000000000, 283.5832628385307999 ) ) ;
#4715=AXIS2_PLACEMENT_3D ( 'NONE', #1281, #1062, #5788 ) ;
#4718=ADVANCED_FACE ( 'NONE', ( #13182 ), #10133, .F. ) ;
#4723=ORIENTED_EDGE ( 'NONE', *, *, #10609, .T. ) ;
#4724=PLANE ( 'NONE',  #17598 ) ;
#4725=CARTESIAN_POINT ( 'NONE',  ( 27.53920554013639688, 73.25972925305640615, 132.4711112102474146 ) ) ;
#4727=VECTOR ( 'NONE', #3685, 1000.000000000000000 ) ;
#4730=VERTEX_POINT ( 'NONE', #7168 ) ;
#4732=VECTOR ( 'NONE', #1145, 1000.000000000000000 ) ;
#4737=CARTESIAN_POINT ( 'NONE',  ( 56.12853591711344592, -23.22718332831461652, 293.5832628385307999 ) ) ;
#4738=VERTEX_POINT ( 'NONE', #19541 ) ;
#4740=DIRECTION ( 'NONE',  ( -0.7881095627315599650, -0.6155349844899714595, 0.000000000000000000 ) ) ;
#4741=LINE ( 'NONE', #18859, #3725 ) ;
#4748=CARTESIAN_POINT ( 'NONE',  ( -38.35506425062487779, -44.43084819159262366, 110.7293897666001214 ) ) ;
#4750=DIRECTION ( 'NONE',  ( 1.000000000000000000, 0.000000000000000000, 0.000000000000000000 ) ) ;
#4753=VERTEX_POINT ( 'NONE', #17817 ) ;
#4754=EDGE_CURVE ( 'NONE', #20158, #17735, #8594, .T. ) ;
#4756=DIRECTION ( 'NONE',  ( 0.3420201433256726542, -0.9396926207859069846, 0.000000000000000000 ) ) ;
#4757=AXIS2_PLACEMENT_3D ( 'NONE', #17706, #15961, #5126 ) ;
#4761=VERTEX_POINT ( 'NONE', #18013 ) ;
#4763=VECTOR ( 'NONE', #16441, 1000.000000000000000 ) ;
#4764=DIRECTION ( 'NONE',  ( 0.4999999999999888978, 0.8660254037844449249, 0.000000000000000000 ) ) ;
#4765=CARTESIAN_POINT ( 'NONE',  ( 12.78021302872850562, -77.21438937758507848, 248.9926560891072143 ) ) ;
#4769=DIRECTION ( 'NONE',  ( -0.7881095627315599650, -0.6155349844899714595, 0.000000000000000000 ) ) ;
#4772=EDGE_CURVE ( 'NONE', #13894, #15168, #6962, .T. ) ;
#4773=DIRECTION ( 'NONE',  ( -0.000000000000000000, -0.000000000000000000, 1.000000000000000000 ) ) ;
#4775=EDGE_CURVE ( 'NONE', #9982, #8985, #9914, .T. ) ;
#4779=CARTESIAN_POINT ( 'NONE',  ( 57.61823435390807902, 19.23677882349220880, 283.5832628385307999 ) ) ;
#4780=VECTOR ( 'NONE', #756, 1000.000000000000000 ) ;
#4782=ORIENTED_EDGE ( 'NONE', *, *, #8914, .F. ) ;
#4785=AXIS2_PLACEMENT_3D ( 'NONE', #1841, #13909, #2974 ) ;
#4786=CARTESIAN_POINT ( 'NONE',  ( 1.379293853801755176, -62.90240729679781850, 293.5832628385307999 ) ) ;
#4787=EDGE_CURVE ( 'NONE', #16297, #9534, #10616, .T. ) ;
#4792=DIRECTION ( 'NONE',  ( -0.9511061040868794558, -0.3088643371590157338, 0.000000000000000000 ) ) ;
#4795=DIRECTION ( 'NONE',  ( 0.000000000000000000, 0.000000000000000000, 1.000000000000000000 ) ) ;
#4797=ORIENTED_EDGE ( 'NONE', *, *, #19975, .F. ) ;
#4798=VECTOR ( 'NONE', #2487, 1000.000000000000000 ) ;
#4802=EDGE_CURVE ( 'NONE', #17872, #9691, #13795, .T. ) ;
#4803=DIRECTION ( 'NONE',  ( -0.6427876096865353661, -0.7660444431189813441, 0.000000000000000000 ) ) ;
#4804=AXIS2_PLACEMENT_3D ( 'NONE', #391, #6643, #12868 ) ;
#4806=DIRECTION ( 'NONE',  ( 0.000000000000000000, 0.000000000000000000, -1.000000000000000000 ) ) ;
#4807=DIRECTION ( 'NONE',  ( -0.000000000000000000, -0.000000000000000000, 1.000000000000000000 ) ) ;
#4808=EDGE_CURVE ( 'NONE', #3935, #5836, #7657, .T. ) ;
#4809=ORIENTED_EDGE ( 'NONE', *, *, #16004, .T. ) ;
#4810=CARTESIAN_POINT ( 'NONE',  ( 0.000000000000000000, 0.000000000000000000, 83.57543755549745867 ) ) ;
#4812=VECTOR ( 'NONE', #10305, 1000.000000000000000 ) ;
#4813=VERTEX_POINT ( 'NONE', #18510 ) ;
#4815=AXIS2_PLACEMENT_3D ( 'NONE', #11950, #3987, #3796 ) ;
#4816=EDGE_LOOP ( 'NONE', ( #13429, #1663, #8595, #12133 ) ) ;
#4818=DIRECTION ( 'NONE',  ( 0.000000000000000000, 0.000000000000000000, 1.000000000000000000 ) ) ;
#4822=CARTESIAN_POINT ( 'NONE',  ( 65.74260934110282051, 8.909359647227704685E-15, 293.5832628385307999 ) ) ;
#4824=DIRECTION ( 'NONE',  ( -0.9396926207859068736, -0.3420201433256725987, 0.000000000000000000 ) ) ;
#4826=DIRECTION ( 'NONE',  ( -0.9271237148521547233, 0.3747554100459928872, 0.000000000000000000 ) ) ;
#4828=CARTESIAN_POINT ( 'NONE',  ( 0.8220851292435327196, 62.91215678473957240, 132.4711112102474146 ) ) ;
#4830=CIRCLE ( 'NONE', #9721, 60.74260934110282051 ) ;
#4831=EDGE_LOOP ( 'NONE', ( #17378, #6527, #10797, #20027 ) ) ;
#4833=AXIS2_PLACEMENT_3D ( 'NONE', #1933, #13351, #2332 ) ;
#4834=CARTESIAN_POINT ( 'NONE',  ( 36.99514631729018532, -48.17959877923561862, 283.5832628385307999 ) ) ;
#4836=VECTOR ( 'NONE', #4979, 1000.000000000000000 ) ;
#4837=ORIENTED_EDGE ( 'NONE', *, *, #5365, .F. ) ;
#4838=VERTEX_POINT ( 'NONE', #10724 ) ;
#4841=VERTEX_POINT ( 'NONE', #9089 ) ;
#4843=FACE_OUTER_BOUND ( 'NONE', #1555, .T. ) ;
#4845=CARTESIAN_POINT ( 'NONE',  ( 5.729042578294381016, 0.2993243175132339062, 293.5832628385307999 ) ) ;
#4848=AXIS2_PLACEMENT_3D ( 'NONE', #9762, #3222, #9466 ) ;
#4849=VECTOR ( 'NONE', #13446, 1000.000000000000114 ) ;
#4851=DIRECTION ( 'NONE',  ( 0.1736481776669404620, -0.9848077530122062440, 0.000000000000000000 ) ) ;
#4858=ADVANCED_FACE ( 'NONE', ( #16976 ), #2661, .F. ) ;
#4862=VECTOR ( 'NONE', #18366, 1000.000000000000000 ) ;
#4864=VECTOR ( 'NONE', #12584, 1000.000000000000000 ) ;
#4865=ORIENTED_EDGE ( 'NONE', *, *, #14259, .T. ) ;
#4866=ORIENTED_EDGE ( 'NONE', *, *, #3956, .T. ) ;
#4867=ADVANCED_FACE ( 'NONE', ( #20040, #7757 ), #6245, .F. ) ;
#4868=ORIENTED_EDGE ( 'NONE', *, *, #14413, .T. ) ;
#4871=LINE ( 'NONE', #15708, #18774 ) ;
#4878=AXIS2_PLACEMENT_3D ( 'NONE', #16541, #19695, #19597 ) ;
#4879=CARTESIAN_POINT ( 'NONE',  ( 0.000000000000000000, 0.000000000000000000, 283.5832628385307999 ) ) ;
#4880=CARTESIAN_POINT ( 'NONE',  ( 27.53920554013639688, 73.25972925305639194, 111.4180192758974499 ) ) ;
#4881=CARTESIAN_POINT ( 'NONE',  ( 74.01264520835154315, -25.47058595421579952, 132.4711112102474146 ) ) ;
#4882=DIRECTION ( 'NONE',  ( -0.000000000000000000, -0.000000000000000000, 1.000000000000000000 ) ) ;
#4890=AXIS2_PLACEMENT_3D ( 'NONE', #488, #8255, #8355 ) ;
#4891=VECTOR ( 'NONE', #12654, 1000.000000000000227 ) ;
#4892=ORIENTED_EDGE ( 'NONE', *, *, #1393, .F. ) ;
#4893=CARTESIAN_POINT ( 'NONE',  ( -68.18670162478832708, -38.41834839689356329, 248.9926560891072143 ) ) ;
#4896=DIRECTION ( 'NONE',  ( -0.5000000000000069944, 0.8660254037844344888, -0.000000000000000000 ) ) ;
#4897=ADVANCED_FACE ( 'NONE', ( #13582 ), #19830, .T. ) ;
#4898=EDGE_CURVE ( 'NONE', #9304, #18854, #6038, .T. ) ;
#4902=ORIENTED_EDGE ( 'NONE', *, *, #12245, .F. ) ;
#4904=CARTESIAN_POINT ( 'NONE',  ( -76.92888220842476699, 14.39940464655786201, 112.0427633081292385 ) ) ;
#4905=ORIENTED_EDGE ( 'NONE', *, *, #12490, .F. ) ;
#4907=DIRECTION ( 'NONE',  ( -0.8830229359480271656, -0.4693298356057563625, 0.000000000000000000 ) ) ;
#4909=AXIS2_PLACEMENT_3D ( 'NONE', #11090, #12626, #15604 ) ;
#4910=CARTESIAN_POINT ( 'NONE',  ( -67.36461649554505016, 39.84224160888970800, 110.9660488491356887 ) ) ;
#4911=EDGE_CURVE ( 'NONE', #8175, #6529, #5939, .T. ) ;
#4914=ORIENTED_EDGE ( 'NONE', *, *, #17890, .F. ) ;
#4916=EDGE_LOOP ( 'NONE', ( #13738, #7816, #6521, #9856 ) ) ;
#4917=ORIENTED_EDGE ( 'NONE', *, *, #2729, .T. ) ;
#4918=DIRECTION ( 'NONE',  ( 0.6427876096865353661, 0.7660444431189813441, -0.000000000000000000 ) ) ;
#4919=ADVANCED_FACE ( 'NONE', ( #7555 ), #12770, .F. ) ;
#4920=ORIENTED_EDGE ( 'NONE', *, *, #8721, .F. ) ;
#4921=EDGE_CURVE ( 'NONE', #2071, #5114, #15746, .T. ) ;
#4923=ADVANCED_FACE ( 'NONE', ( #11132 ), #9401, .F. ) ;
#4924=ADVANCED_FACE ( 'NONE', ( #16056 ), #9701, .F. ) ;
#4927=EDGE_LOOP ( 'NONE', ( #19709, #10613, #2737, #12940 ) ) ;
#4930=CARTESIAN_POINT ( 'NONE',  ( -38.41834839689332171, 68.18670162478844077, 248.9926560891072143 ) ) ;
#4931=CARTESIAN_POINT ( 'NONE',  ( 44.43084819159276577, -38.35506425062471436, 132.4711112102474146 ) ) ;
#4932=VECTOR ( 'NONE', #15742, 1000.000000000000114 ) ;
#4933=CARTESIAN_POINT ( 'NONE',  ( 0.000000000000000000, 0.000000000000000000, 293.5832628385307999 ) ) ;
#4936=DIRECTION ( 'NONE',  ( 0.3088643371590157338, -0.9511061040868794558, 0.000000000000000000 ) ) ;
#4943=ORIENTED_EDGE ( 'NONE', *, *, #10223, .T. ) ;
#4945=ORIENTED_EDGE ( 'NONE', *, *, #3519, .T. ) ;
#4947=EDGE_LOOP ( 'NONE', ( #12489, #19723, #14734, #18986 ) ) ;
#4949=DIRECTION ( 'NONE',  ( 0.000000000000000000, 0.000000000000000000, 1.000000000000000000 ) ) ;
#4953=CARTESIAN_POINT ( 'NONE',  ( -17.50000000000001066, 2.143131898507869431E-15, 4.999999999999948486 ) ) ;
#4954=DIRECTION ( 'NONE',  ( 0.8660254037844328234, 0.5000000000000101030, 0.000000000000000000 ) ) ;
#4958=CARTESIAN_POINT ( 'NONE',  ( -30.05702882063063086, -50.41613078340792242, 110.9660488491356887 ) ) ;
#4966=VECTOR ( 'NONE', #13839, 1000.000000000000000 ) ;
#4969=EDGE_CURVE ( 'NONE', #8266, #9691, #12668, .T. ) ;
#4971=DIRECTION ( 'NONE',  ( 0.000000000000000000, 0.000000000000000000, 1.000000000000000000 ) ) ;
#4973=CARTESIAN_POINT ( 'NONE',  ( 4.811834253409037032, 3.123743752084113812, 293.5832628385307999 ) ) ;
#4976=DIRECTION ( 'NONE',  ( -0.000000000000000000, -0.000000000000000000, 1.000000000000000000 ) ) ;
#4979=DIRECTION ( 'NONE',  ( 0.8660254037844328234, 0.5000000000000101030, 0.000000000000000000 ) ) ;
#4984=ORIENTED_EDGE ( 'NONE', *, *, #14641, .T. ) ;
#4985=ORIENTED_EDGE ( 'NONE', *, *, #5809, .F. ) ;
#4988=DIRECTION ( 'NONE',  ( -0.8660254037844380415, -0.5000000000000009992, 0.000000000000000000 ) ) ;
#4989=VECTOR ( 'NONE', #17838, 999.9999999999998863 ) ;
#4990=CIRCLE ( 'NONE', #11816, 60.74260934110282051 ) ;
#4993=EDGE_CURVE ( 'NONE', #11573, #6558, #8920, .T. ) ;
#4995=DIRECTION ( 'NONE',  ( -0.8830229359480288309, -0.4693298356057531984, 0.000000000000000000 ) ) ;
#4997=ORIENTED_EDGE ( 'NONE', *, *, #12081, .F. ) ;
#4998=AXIS2_PLACEMENT_3D ( 'NONE', #19557, #8710, #15148 ) ;
#5002=ORIENTED_EDGE ( 'NONE', *, *, #19119, .T. ) ;
#5003=CYLINDRICAL_SURFACE ( 'NONE', #17225, 62.91752772691707207 ) ;
#5004=LINE ( 'NONE', #4696, #6510 ) ;
#5013=EDGE_LOOP ( 'NONE', ( #16850, #19899, #1456, #18040 ) ) ;
#5014=EDGE_CURVE ( 'NONE', #17034, #1059, #9596, .T. ) ;
#5016=EDGE_LOOP ( 'NONE', ( #17162, #10017, #17921, #12194 ) ) ;
#5021=EDGE_CURVE ( 'NONE', #7664, #14568, #7962, .T. ) ;
#5023=AXIS2_PLACEMENT_3D ( 'NONE', #18720, #4703, #9604 ) ;
#5029=VECTOR ( 'NONE', #15784, 999.9999999999998863 ) ;
#5031=DIRECTION ( 'NONE',  ( 1.000000000000000000, 0.000000000000000000, 0.000000000000000000 ) ) ;
#5033=CARTESIAN_POINT ( 'NONE',  ( -5.111158570922238020, 2.605298826210300511, 283.5832628385307999 ) ) ;
#5034=AXIS2_PLACEMENT_3D ( 'NONE', #509, #14521, #6655 ) ;
#5035=EDGE_CURVE ( 'NONE', #6926, #6009, #17292, .T. ) ;
#5038=ORIENTED_EDGE ( 'NONE', *, *, #10505, .F. ) ;
#5039=ADVANCED_FACE ( 'NONE', ( #3269 ), #1725, .F. ) ;
#5044=ORIENTED_EDGE ( 'NONE', *, *, #3382, .F. ) ;
#5048=ORIENTED_EDGE ( 'NONE', *, *, #6968, .T. ) ;
#5049=CARTESIAN_POINT ( 'NONE',  ( 39.84224160888901167, 67.36461649554546227, 248.9926560891072143 ) ) ;
#5052=ADVANCED_FACE ( 'NONE', ( #499 ), #6743, .T. ) ;
#5054=VERTEX_POINT ( 'NONE', #15850 ) ;
#5055=DIRECTION ( 'NONE',  ( -0.6427876096865353661, -0.7660444431189813441, 0.000000000000000000 ) ) ;
#5056=LINE ( 'NONE', #13099, #18438 ) ;
#5058=LINE ( 'NONE', #1773, #19937 ) ;
#5060=EDGE_CURVE ( 'NONE', #15899, #10298, #14314, .T. ) ;
#5068=EDGE_CURVE ( 'NONE', #17628, #1213, #2728, .T. ) ;
#5069=ORIENTED_EDGE ( 'NONE', *, *, #4754, .F. ) ;
#5071=EDGE_LOOP ( 'NONE', ( #10394, #4569, #10823, #1559 ) ) ;
#5074=DIRECTION ( 'NONE',  ( 0.000000000000000000, 0.000000000000000000, 1.000000000000000000 ) ) ;
#5077=CARTESIAN_POINT ( 'NONE',  ( 1.678175111358129801, 5.485913980968024184, 293.5832628385307999 ) ) ;
#5078=CARTESIAN_POINT ( 'NONE',  ( -59.51523122377252406, 12.14914984460740932, 283.5832628385307999 ) ) ;
#5079=DIRECTION ( 'NONE',  ( 1.000000000000000000, 0.000000000000000000, -0.000000000000000000 ) ) ;
#5080=CARTESIAN_POINT ( 'NONE',  ( 0.000000000000000000, 0.000000000000000000, 4.999999999999948486 ) ) ;
#5081=CIRCLE ( 'NONE', #16506, 60.74260934110282051 ) ;
#5082=CARTESIAN_POINT ( 'NONE',  ( 5.590028426173780929, 1.289614712049194534, 293.5832628385307999 ) ) ;
#5087=ORIENTED_EDGE ( 'NONE', *, *, #2258, .T. ) ;
#5088=ORIENTED_EDGE ( 'NONE', *, *, #19969, .F. ) ;
#5089=ORIENTED_EDGE ( 'NONE', *, *, #6746, .T. ) ;
#5090=ORIENTED_EDGE ( 'NONE', *, *, #16524, .F. ) ;
#5091=CARTESIAN_POINT ( 'NONE',  ( -1.379293853801755176, 78.26059000578311498, 132.4711112102474146 ) ) ;
#5092=PRODUCT_DEFINITION_SHAPE ( 'NONE', 'NONE',  #12261 ) ;
#5094=LINE ( 'NONE', #3448, #211 ) ;
#5095=AXIS2_PLACEMENT_3D ( 'NONE', #6586, #10045, #14245 ) ;
#5096=CARTESIAN_POINT ( 'NONE',  ( -59.06449708980196078, -51.36153797460887915, 132.4711112102474146 ) ) ;
#5098=DIRECTION ( 'NONE',  ( -0.000000000000000000, -0.000000000000000000, 1.000000000000000000 ) ) ;
#5099=ORIENTED_EDGE ( 'NONE', *, *, #3637, .T. ) ;
#5101=DIRECTION ( 'NONE',  ( -0.000000000000000000, -0.000000000000000000, 1.000000000000000000 ) ) ;
#5104=CYLINDRICAL_SURFACE ( 'NONE', #11703, 60.74260934110282051 ) ;
#5108=DIRECTION ( 'NONE',  ( -0.000000000000000000, -0.000000000000000000, 1.000000000000000000 ) ) ;
#5111=ORIENTED_EDGE ( 'NONE', *, *, #1942, .F. ) ;
#5112=EDGE_CURVE ( 'NONE', #2560, #6500, #11814, .T. ) ;
#5114=VERTEX_POINT ( 'NONE', #985 ) ;
#5115=ORIENTED_EDGE ( 'NONE', *, *, #3022, .F. ) ;
#5116=DIRECTION ( 'NONE',  ( 0.000000000000000000, 0.000000000000000000, 1.000000000000000000 ) ) ;
#5117=ORIENTED_EDGE ( 'NONE', *, *, #17857, .F. ) ;
#5119=LINE ( 'NONE', #507, #14328 ) ;
#5120=VECTOR ( 'NONE', #6069, 1000.000000000000227 ) ;
#5122=CARTESIAN_POINT ( 'NONE',  ( 60.08331549348424971, 8.939227532413909216, 293.5832628385307999 ) ) ;
#5123=ORIENTED_EDGE ( 'NONE', *, *, #6895, .T. ) ;
#5126=DIRECTION ( 'NONE',  ( 1.000000000000000000, 0.000000000000000000, 0.000000000000000000 ) ) ;
#5127=EDGE_CURVE ( 'NONE', #12537, #15505, #10293, .T. ) ;
#5130=LINE ( 'NONE', #17606, #6174 ) ;
#5131=DIRECTION ( 'NONE',  ( -0.000000000000000000, -0.000000000000000000, 1.000000000000000000 ) ) ;
#5133=VERTEX_POINT ( 'NONE', #18081 ) ;
#5135=DIRECTION ( 'NONE',  ( 0.3420201433256757073, -0.9396926207859057634, 0.000000000000000000 ) ) ;
#5136=LINE ( 'NONE', #11360, #14057 ) ;
#5138=AXIS2_PLACEMENT_3D ( 'NONE', #2428, #4150, #8656 ) ;
#5139=ORIENTED_EDGE ( 'NONE', *, *, #13851, .T. ) ;
#5140=EDGE_CURVE ( 'NONE', #11666, #14566, #2434, .T. ) ;
#5150=FACE_OUTER_BOUND ( 'NONE', #1908, .T. ) ;
#5152=VERTEX_POINT ( 'NONE', #9906 ) ;
#5158=CARTESIAN_POINT ( 'NONE',  ( 50.93469132750264095, 59.42266395395811429, 110.7293897666001214 ) ) ;
#5159=FACE_OUTER_BOUND ( 'NONE', #12209, .T. ) ;
#5161=DIRECTION ( 'NONE',  ( -0.1736481776669306920, 0.9848077530122080203, 0.000000000000000000 ) ) ;
#5162=CARTESIAN_POINT ( 'NONE',  ( 0.000000000000000000, 0.000000000000000000, 4.999999999999948486 ) ) ;
#5168=ORIENTED_EDGE ( 'NONE', *, *, #6355, .F. ) ;
#5169=VECTOR ( 'NONE', #2950, 1000.000000000000114 ) ;
#5177=CARTESIAN_POINT ( 'NONE',  ( 57.61627707419551570, 19.23614321207255884, 283.5832628385307999 ) ) ;
#5178=DIRECTION ( 'NONE',  ( 1.000000000000000000, 0.000000000000000000, 0.000000000000000000 ) ) ;
#5182=LINE ( 'NONE', #13036, #13353 ) ;
#5184=CARTESIAN_POINT ( 'NONE',  ( -78.26059000578311498, -1.379293853802032732, 132.4711112102474146 ) ) ;
#5188=EDGE_LOOP ( 'NONE', ( #7994, #10340, #14731, #298 ) ) ;
#5189=ORIENTED_EDGE ( 'NONE', *, *, #12912, .F. ) ;
#5193=DIRECTION ( 'NONE',  ( -0.7660444431189707970, -0.6427876096865481337, -0.000000000000000000 ) ) ;
#5194=AXIS2_PLACEMENT_3D ( 'NONE', #16979, #4600, #12262 ) ;
#5195=CIRCLE ( 'NONE', #20202, 60.74260934110282051 ) ;
#5199=CARTESIAN_POINT ( 'NONE',  ( -39.80940113485987553, 48.72193424476490975, 132.4711112102474146 ) ) ;
#5200=EDGE_LOOP ( 'NONE', ( #19349, #5514, #15572, #1436 ) ) ;
#5206=DIRECTION ( 'NONE',  ( -0.000000000000000000, -0.000000000000000000, 1.000000000000000000 ) ) ;
#5207=CARTESIAN_POINT ( 'NONE',  ( 60.47951622432751151, 49.67518383744852883, 110.7293897666001214 ) ) ;
#5212=EDGE_LOOP ( 'NONE', ( #921, #1087, #18578, #16287 ) ) ;
#5214=DIRECTION ( 'NONE',  ( 1.000000000000000000, 0.000000000000000000, 0.000000000000000000 ) ) ;
#5216=ORIENTED_EDGE ( 'NONE', *, *, #13359, .T. ) ;
#5217=CYLINDRICAL_SURFACE ( 'NONE', #8588, 62.91752772691707207 ) ;
#5219=CARTESIAN_POINT ( 'NONE',  ( 47.29944656917759005, 41.48948842197133757, 132.4711112102474146 ) ) ;
#5224=VECTOR ( 'NONE', #17822, 1000.000000000000000 ) ;
#5225=AXIS2_PLACEMENT_3D ( 'NONE', #3329, #16114, #5178 ) ;
#5226=EDGE_CURVE ( 'NONE', #8307, #4702, #5500, .T. ) ;
#5227=FACE_OUTER_BOUND ( 'NONE', #1962, .T. ) ;
#5230=DIRECTION ( 'NONE',  ( -0.9848077530122085754, 0.1736481776669273336, 0.000000000000000000 ) ) ;
#5231=DIRECTION ( 'NONE',  ( -0.000000000000000000, -0.000000000000000000, 1.000000000000000000 ) ) ;
#5232=FACE_OUTER_BOUND ( 'NONE', #10753, .T. ) ;
#5234=CARTESIAN_POINT ( 'NONE',  ( 59.39925916207545242, 20.74471755083624203, 132.4711112102474146 ) ) ;
#5235=CARTESIAN_POINT ( 'NONE',  ( -57.65577537092151772, 11.00103590902930328, 112.0427633081292385 ) ) ;
#5236=ORIENTED_EDGE ( 'NONE', *, *, #12545, .T. ) ;
#5241=ORIENTED_EDGE ( 'NONE', *, *, #11091, .F. ) ;
#5244=ORIENTED_EDGE ( 'NONE', *, *, #13903, .F. ) ;
#5246=ORIENTED_EDGE ( 'NONE', *, *, #3143, .T. ) ;
#5247=DIRECTION ( 'NONE',  ( -0.9848077530122062440, -0.1736481776669404620, -0.000000000000000000 ) ) ;
#5256=PLANE ( 'NONE',  #1352 ) ;
#5259=ORIENTED_EDGE ( 'NONE', *, *, #19589, .T. ) ;
#5264=ORIENTED_EDGE ( 'NONE', *, *, #18361, .F. ) ;
#5265=ORIENTED_EDGE ( 'NONE', *, *, #16057, .F. ) ;
#5268=ADVANCED_FACE ( 'NONE', ( #12230 ), #5700, .T. ) ;
#5269=CARTESIAN_POINT ( 'NONE',  ( 54.67896814532641514, 21.36933070621782349, 111.4180192758973362 ) ) ;
#5270=DIRECTION ( 'NONE',  ( -0.9781142164131917394, 0.2080686897406911207, 0.000000000000000000 ) ) ;
#5272=ORIENTED_EDGE ( 'NONE', *, *, #17501, .F. ) ;
#5273=FACE_OUTER_BOUND ( 'NONE', #6023, .T. ) ;
#5277=CARTESIAN_POINT ( 'NONE',  ( 0.000000000000000000, 0.000000000000000000, 283.5832628385307999 ) ) ;
#5279=VECTOR ( 'NONE', #7699, 1000.000000000000000 ) ;
#5280=CARTESIAN_POINT ( 'NONE',  ( -4.811834253408968642, -3.123743752084039205, 293.5832628385307999 ) ) ;
#5283=ADVANCED_FACE ( 'NONE', ( #16649 ), #18382, .T. ) ;
#5284=ORIENTED_EDGE ( 'NONE', *, *, #1273, .T. ) ;
#5292=CARTESIAN_POINT ( 'NONE',  ( -41.48948842197086861, 47.29944656917800216, 248.9926560891072143 ) ) ;
#5293=LINE ( 'NONE', #774, #14513 ) ;
#5298=EDGE_LOOP ( 'NONE', ( #1751, #11217, #9202 ) ) ;
#5301=LINE ( 'NONE', #14701, #7873 ) ;
#5311=VERTEX_POINT ( 'NONE', #12124 ) ;
#5312=DIRECTION ( 'NONE',  ( 0.000000000000000000, 0.000000000000000000, -1.000000000000000000 ) ) ;
#5313=VERTEX_POINT ( 'NONE', #13556 ) ;
#5320=AXIS2_PLACEMENT_3D ( 'NONE', #8262, #8933, #8463 ) ;
#5325=DIRECTION ( 'NONE',  ( -1.000000000000000000, -1.047444401652940164E-14, 0.000000000000000000 ) ) ;
#5328=DIRECTION ( 'NONE',  ( 0.000000000000000000, 0.000000000000000000, -1.000000000000000000 ) ) ;
#5330=ORIENTED_EDGE ( 'NONE', *, *, #2154, .F. ) ;
#5331=CARTESIAN_POINT ( 'NONE',  ( 0.000000000000000000, 0.000000000000000000, 283.5832628385307999 ) ) ;
#5340=CARTESIAN_POINT ( 'NONE',  ( 0.000000000000000000, 0.000000000000000000, 283.5832628385307999 ) ) ;
#5341=CARTESIAN_POINT ( 'NONE',  ( 38.41834839689379777, -68.18670162478818497, 132.4711112102474146 ) ) ;
#5342=ORIENTED_EDGE ( 'NONE', *, *, #19975, .T. ) ;
#5343=AXIS2_PLACEMENT_3D ( 'NONE', #503, #795, #14710 ) ;
#5344=CARTESIAN_POINT ( 'NONE',  ( 57.94128254008182921, 9.381844291199925578, 248.9926560891072143 ) ) ;
#5345=DIRECTION ( 'NONE',  ( 1.000000000000000000, 0.000000000000000000, 0.000000000000000000 ) ) ;
#5348=VECTOR ( 'NONE', #4818, 1000.000000000000000 ) ;
#5349=LINE ( 'NONE', #13011, #18313 ) ;
#5350=CARTESIAN_POINT ( 'NONE',  ( 19.23677882349201695, -57.61823435390814296, 283.5832628385307999 ) ) ;
#5351=VECTOR ( 'NONE', #8564, 1000.000000000000000 ) ;
#5352=LINE ( 'NONE', #17936, #14430 ) ;
#5355=ORIENTED_EDGE ( 'NONE', *, *, #19608, .F. ) ;
#5356=DIRECTION ( 'NONE',  ( -0.000000000000000000, -0.000000000000000000, 1.000000000000000000 ) ) ;
#5357=AXIS2_PLACEMENT_3D ( 'NONE', #12824, #19085, #10254 ) ;
#5361=VERTEX_POINT ( 'NONE', #2837 ) ;
#5364=LINE ( 'NONE', #9761, #2435 ) ;
#5365=EDGE_CURVE ( 'NONE', #4682, #11852, #7629, .T. ) ;
#5366=CARTESIAN_POINT ( 'NONE',  ( -48.72193424476477475, -39.80940113486002474, 248.9926560891072143 ) ) ;
#5368=VECTOR ( 'NONE', #10046, 1000.000000000000227 ) ;
#5369=LINE ( 'NONE', #17354, #3910 ) ;
#5371=EDGE_CURVE ( 'NONE', #7889, #11536, #17523, .T. ) ;
#5375=AXIS2_PLACEMENT_3D ( 'NONE', #10181, #577, #6826 ) ;
#5384=CARTESIAN_POINT ( 'NONE',  ( 0.000000000000000000, 0.000000000000000000, 269.6944534026102360 ) ) ;
#5386=CARTESIAN_POINT ( 'NONE',  ( 25.99419088092191643, -73.82206860051539365, 248.9926560891072143 ) ) ;
#5388=CARTESIAN_POINT ( 'NONE',  ( 0.000000000000000000, 0.000000000000000000, 283.5832628385307999 ) ) ;
#5393=LINE ( 'NONE', #19314, #15663 ) ;
#5394=EDGE_CURVE ( 'NONE', #3790, #19700, #19482, .T. ) ;
#5397=CARTESIAN_POINT ( 'NONE',  ( -9.381844291199351815, 57.94128254008192158, 248.9926560891072143 ) ) ;
#5399=VECTOR ( 'NONE', #15429, 1000.000000000000000 ) ;
#5402=DIRECTION ( 'NONE',  ( 0.000000000000000000, 0.000000000000000000, -1.000000000000000000 ) ) ;
#5404=VERTEX_POINT ( 'NONE', #2602 ) ;
#5407=ORIENTED_EDGE ( 'NONE', *, *, #12722, .F. ) ;
#5412=CARTESIAN_POINT ( 'NONE',  ( -0.7000608949449798057, -5.693982670708954252, 293.5832628385307999 ) ) ;
#5417=VECTOR ( 'NONE', #11905, 1000.000000000000114 ) ;
#5418=ORIENTED_EDGE ( 'NONE', *, *, #17033, .T. ) ;
#5423=LINE ( 'NONE', #7056, #18656 ) ;
#5424=CARTESIAN_POINT ( 'NONE',  ( 28.06281046684275182, -73.06915264522011455, 111.4180192758973362 ) ) ;
#5427=CARTESIAN_POINT ( 'NONE',  ( 61.70726652483817531, 12.28122767885865407, 132.4711112102474146 ) ) ;
#5430=ORIENTED_EDGE ( 'NONE', *, *, #3856, .T. ) ;
#5433=CARTESIAN_POINT ( 'NONE',  ( -1.379293853801755176, 78.26059000578311498, 112.7772637782949943 ) ) ;
#5434=ORIENTED_EDGE ( 'NONE', *, *, #18110, .F. ) ;
#5436=ORIENTED_EDGE ( 'NONE', *, *, #3283, .F. ) ;
#5437=EDGE_LOOP ( 'NONE', ( #4145, #3543, #16654, #16540 ) ) ;
#5438=DIRECTION ( 'NONE',  ( 0.1736481776669273336, 0.9848077530122085754, 0.000000000000000000 ) ) ;
#5442=ORIENTED_EDGE ( 'NONE', *, *, #2615, .F. ) ;
#5443=VECTOR ( 'NONE', #7750, 1000.000000000000114 ) ;
#5445=DIRECTION ( 'NONE',  ( 0.1736481776669374366, -0.9848077530122067991, 0.000000000000000000 ) ) ;
#5447=DIRECTION ( 'NONE',  ( -0.7660444431189792347, 0.6427876096865379196, 0.000000000000000000 ) ) ;
#5454=EDGE_LOOP ( 'NONE', ( #8913, #11367, #7685, #5550 ) ) ;
#5455=CIRCLE ( 'NONE', #15240, 60.74260934110282051 ) ;
#5458=DIRECTION ( 'NONE',  ( -0.3420201433256725987, 0.9396926207859068736, 0.000000000000000000 ) ) ;
#5459=AXIS2_PLACEMENT_3D ( 'NONE', #5952, #4302, #16789 ) ;
#5460=DIRECTION ( 'NONE',  ( 0.3420201433256790380, -0.9396926207859046531, 0.000000000000000000 ) ) ;
#5461=DIRECTION ( 'NONE',  ( -0.6692498792541777819, -0.7430374143461878633, 0.000000000000000000 ) ) ;
#5464=ADVANCED_FACE ( 'NONE', ( #7497 ), #12196, .F. ) ;
#5465=CARTESIAN_POINT ( 'NONE',  ( -51.24071425735603924, 32.61983739937744531, 283.5832628385307999 ) ) ;
#5469=DIRECTION ( 'NONE',  ( 0.5000000000000101030, -0.8660254037844328234, 0.000000000000000000 ) ) ;
#5477=ORIENTED_EDGE ( 'NONE', *, *, #11374, .T. ) ;
#5478=VERTEX_POINT ( 'NONE', #15375 ) ;
#5480=DIRECTION ( 'NONE',  ( 0.9848077530122103518, -0.1736481776669172583, 0.000000000000000000 ) ) ;
#5481=EDGE_LOOP ( 'NONE', ( #11039, #18396, #16367, #10534 ) ) ;
#5482=CARTESIAN_POINT ( 'NONE',  ( 0.000000000000000000, 0.000000000000000000, 293.5832628385307999 ) ) ;
#5483=FACE_OUTER_BOUND ( 'NONE', #472, .T. ) ;
#5484=CARTESIAN_POINT ( 'NONE',  ( 0.000000000000000000, 0.000000000000000000, 293.5832628385307999 ) ) ;
#5485=ORIENTED_EDGE ( 'NONE', *, *, #16912, .F. ) ;
#5486=LINE ( 'NONE', #10092, #5417 ) ;
#5487=DIRECTION ( 'NONE',  ( -0.000000000000000000, -0.000000000000000000, 1.000000000000000000 ) ) ;
#5489=ADVANCED_FACE ( 'NONE', ( #18666 ), #9341, .T. ) ;
#5490=ORIENTED_EDGE ( 'NONE', *, *, #6871, .T. ) ;
#5491=LINE ( 'NONE', #3948, #17945 ) ;
#5492=VECTOR ( 'NONE', #3813, 1000.000000000000000 ) ;
#5493=DIRECTION ( 'NONE',  ( 0.6692498792541753394, 0.7430374143461900838, 0.000000000000000000 ) ) ;
#5494=CARTESIAN_POINT ( 'NONE',  ( -62.91215678473957240, 0.8220851292433130064, 293.5832628385307999 ) ) ;
#5495=FACE_OUTER_BOUND ( 'NONE', #8432, .T. ) ;
#5500=LINE ( 'NONE', #12965, #14815 ) ;
#5502=ORIENTED_EDGE ( 'NONE', *, *, #6159, .T. ) ;
#5503=ADVANCED_FACE ( 'NONE', ( #1872 ), #14148, .F. ) ;
#5504=VECTOR ( 'NONE', #8430, 1000.000000000000000 ) ;
#5511=CARTESIAN_POINT ( 'NONE',  ( 0.000000000000000000, 0.000000000000000000, 293.5832628385307999 ) ) ;
#5513=CARTESIAN_POINT ( 'NONE',  ( -47.29944656917786006, -41.48948842197101783, 293.5832628385307999 ) ) ;
#5514=ORIENTED_EDGE ( 'NONE', *, *, #1426, .T. ) ;
#5515=EDGE_CURVE ( 'NONE', #1786, #19610, #1982, .T. ) ;
#5517=CARTESIAN_POINT ( 'NONE',  ( -31.77187437101503775, -51.77076963420834943, 293.5832628385307999 ) ) ;
#5518=VECTOR ( 'NONE', #17904, 1000.000000000000227 ) ;
#5520=CARTESIAN_POINT ( 'NONE',  ( 28.94983032429829350, -53.40245231972188833, 293.5832628385307999 ) ) ;
#5521=VECTOR ( 'NONE', #1896, 1000.000000000000000 ) ;
#5525=LINE ( 'NONE', #13179, #6632 ) ;
#5527=DIRECTION ( 'NONE',  ( 1.000000000000000000, 0.000000000000000000, 0.000000000000000000 ) ) ;
#5533=ORIENTED_EDGE ( 'NONE', *, *, #12630, .F. ) ;
#5536=VECTOR ( 'NONE', #17874, 1000.000000000000000 ) ;
#5537=CARTESIAN_POINT ( 'NONE',  ( 73.82206860051529418, 25.99419088092216867, 248.9926560891072143 ) ) ;
#5538=DIRECTION ( 'NONE',  ( 0.9396926207859082059, 0.3420201433256694901, 0.000000000000000000 ) ) ;
#5539=ORIENTED_EDGE ( 'NONE', *, *, #13761, .F. ) ;
#5543=FACE_OUTER_BOUND ( 'NONE', #8293, .T. ) ;
#5544=CARTESIAN_POINT ( 'NONE',  ( -40.32479851956769323, 67.08601213326579682, 132.4711112102474146 ) ) ;
#5547=VECTOR ( 'NONE', #11347, 1000.000000000000114 ) ;
#5550=ORIENTED_EDGE ( 'NONE', *, *, #1860, .T. ) ;
#5552=CARTESIAN_POINT ( 'NONE',  ( 53.40063514825077107, 28.94886449118924432, 293.5832628385307999 ) ) ;
#5555=VERTEX_POINT ( 'NONE', #7025 ) ;
#5556=EDGE_CURVE ( 'NONE', #17774, #17628, #19313, .T. ) ;
#5559=AXIS2_PLACEMENT_3D ( 'NONE', #6976, #543, #4095 ) ;
#5563=DIRECTION ( 'NONE',  ( -0.000000000000000000, -0.000000000000000000, 1.000000000000000000 ) ) ;
#5564=FACE_OUTER_BOUND ( 'NONE', #10194, .T. ) ;
#5565=ORIENTED_EDGE ( 'NONE', *, *, #11939, .F. ) ;
#5571=LINE ( 'NONE', #2134, #15512 ) ;
#5572=VERTEX_POINT ( 'NONE', #8552 ) ;
#5574=ORIENTED_EDGE ( 'NONE', *, *, #508, .F. ) ;
#5575=ORIENTED_EDGE ( 'NONE', *, *, #2391, .T. ) ;
#5577=EDGE_CURVE ( 'NONE', #18899, #15118, #5486, .T. ) ;
#5579=VECTOR ( 'NONE', #7724, 1000.000000000000227 ) ;
#5583=AXIS2_PLACEMENT_3D ( 'NONE', #11790, #13322, #17852 ) ;
#5587=CARTESIAN_POINT ( 'NONE',  ( 0.2993243175132189737, -5.729042578294415655, 293.5832628385307999 ) ) ;
#5595=VERTEX_POINT ( 'NONE', #8652 ) ;
#5596=AXIS2_PLACEMENT_3D ( 'NONE', #828, #2472, #8704 ) ;
#5597=DIRECTION ( 'NONE',  ( 0.000000000000000000, 0.000000000000000000, 1.000000000000000000 ) ) ;
#5601=EDGE_CURVE ( 'NONE', #16315, #15959, #17976, .T. ) ;
#5605=ORIENTED_EDGE ( 'NONE', *, *, #7734, .F. ) ;
#5606=CARTESIAN_POINT ( 'NONE',  ( 28.43859219408686911, 46.49849886828724976, 248.9926560891072143 ) ) ;
#5607=CARTESIAN_POINT ( 'NONE',  ( 36.99514631729018532, -48.17959877923561862, 293.5832628385307999 ) ) ;
#5608=CARTESIAN_POINT ( 'NONE',  ( 0.000000000000000000, 0.000000000000000000, 283.5832628385307999 ) ) ;
#5609=CARTESIAN_POINT ( 'NONE',  ( 0.000000000000000000, 0.000000000000000000, 132.4711112102474146 ) ) ;
#5610=ORIENTED_EDGE ( 'NONE', *, *, #838, .F. ) ;
#5611=EDGE_CURVE ( 'NONE', #3122, #10094, #14793, .T. ) ;
#5613=DIRECTION ( 'NONE',  ( 1.000000000000000000, 0.000000000000000000, -0.000000000000000000 ) ) ;
#5614=EDGE_CURVE ( 'NONE', #9195, #16956, #580, .T. ) ;
#5615=CARTESIAN_POINT ( 'NONE',  ( 60.72279549541555355, -1.629937663769388090, 293.5832628385307999 ) ) ;
#5616=EDGE_CURVE ( 'NONE', #8743, #19246, #10185, .T. ) ;
#5620=PLANE ( 'NONE',  #14914 ) ;
#5621=DIRECTION ( 'NONE',  ( -0.000000000000000000, -0.000000000000000000, 1.000000000000000000 ) ) ;
#5622=CARTESIAN_POINT ( 'NONE',  ( 58.69016442926520938, 1.379293853802370018, 112.7772637782949516 ) ) ;
#5624=CARTESIAN_POINT ( 'NONE',  ( -45.46712722958807973, 40.27908801170008957, 293.5832628385307999 ) ) ;
#5626=ORIENTED_EDGE ( 'NONE', *, *, #9175, .F. ) ;
#5627=EDGE_LOOP ( 'NONE', ( #1726, #3042, #13561, #18515 ) ) ;
#5628=EDGE_CURVE ( 'NONE', #13590, #15181, #683, .T. ) ;
#5629=ADVANCED_FACE ( 'NONE', ( #19408 ), #19692, .T. ) ;
#5630=ORIENTED_EDGE ( 'NONE', *, *, #14367, .T. ) ;
#5631=CARTESIAN_POINT ( 'NONE',  ( 14.94814811854963388, -76.83212392882498420, 112.0427633081291816 ) ) ;
#5632=DIRECTION ( 'NONE',  ( 0.3088643371590157338, -0.9511061040868794558, 0.000000000000000000 ) ) ;
#5633=CIRCLE ( 'NONE', #13134, 60.74260934110282051 ) ;
#5635=CIRCLE ( 'NONE', #13805, 65.74260934110282051 ) ;
#5637=FACE_OUTER_BOUND ( 'NONE', #18493, .T. ) ;
#5640=EDGE_CURVE ( 'NONE', #18497, #5054, #2620, .T. ) ;
#5643=CARTESIAN_POINT ( 'NONE',  ( -7.948651060879014629, 60.22029172860440838, 283.5832628385307999 ) ) ;
#5644=DIRECTION ( 'NONE',  ( -0.000000000000000000, -0.000000000000000000, 1.000000000000000000 ) ) ;
#5646=CARTESIAN_POINT ( 'NONE',  ( 1.379293853801755176, -62.90240729679781850, 132.4711112102474146 ) ) ;
#5651=AXIS2_PLACEMENT_3D ( 'NONE', #13273, #3884, #13081 ) ;
#5652=ORIENTED_EDGE ( 'NONE', *, *, #3994, .T. ) ;
#5657=VERTEX_POINT ( 'NONE', #13544 ) ;
#5659=AXIS2_PLACEMENT_3D ( 'NONE', #13905, #20150, #12367 ) ;
#5662=FACE_OUTER_BOUND ( 'NONE', #13250, .T. ) ;
#5663=AXIS2_PLACEMENT_3D ( 'NONE', #17493, #17393, #11341 ) ;
#5665=EDGE_CURVE ( 'NONE', #8743, #7392, #15212, .T. ) ;
#5667=CARTESIAN_POINT ( 'NONE',  ( -60.22029172860436574, -7.948651060879222463, 283.5832628385307999 ) ) ;
#5673=CARTESIAN_POINT ( 'NONE',  ( 0.000000000000000000, 0.000000000000000000, 283.5832628385307999 ) ) ;
#5674=PLANE ( 'NONE',  #6145 ) ;
#5676=ORIENTED_EDGE ( 'NONE', *, *, #10721, .T. ) ;
#5677=AXIS2_PLACEMENT_3D ( 'NONE', #5920, #15421, #9284 ) ;
#5682=ORIENTED_EDGE ( 'NONE', *, *, #11479, .F. ) ;
#5686=VECTOR ( 'NONE', #13049, 1000.000000000000000 ) ;
#5687=DIRECTION ( 'NONE',  ( 0.000000000000000000, 0.000000000000000000, 1.000000000000000000 ) ) ;
#5688=ORIENTED_EDGE ( 'NONE', *, *, #9651, .F. ) ;
#5691=ORIENTED_EDGE ( 'NONE', *, *, #16771, .F. ) ;
#5692=DIRECTION ( 'NONE',  ( 1.000000000000000000, 0.000000000000000000, 0.000000000000000000 ) ) ;
#5693=CARTESIAN_POINT ( 'NONE',  ( 44.43084819159276577, -38.35506425062471436, 248.9926560891072143 ) ) ;
#5700=PLANE ( 'NONE',  #11296 ) ;
#5702=ORIENTED_EDGE ( 'NONE', *, *, #3358, .F. ) ;
#5705=VERTEX_POINT ( 'NONE', #1383 ) ;
#5710=LINE ( 'NONE', #18188, #5368 ) ;
#5711=VECTOR ( 'NONE', #7159, 1000.000000000000227 ) ;
#5712=LINE ( 'NONE', #16659, #7055 ) ;
#5714=VERTEX_POINT ( 'NONE', #13856 ) ;
#5715=CARTESIAN_POINT ( 'NONE',  ( 0.000000000000000000, 0.000000000000000000, 293.5832628385307999 ) ) ;
#5723=CIRCLE ( 'NONE', #4077, 79.75827554147308263 ) ;
#5728=ORIENTED_EDGE ( 'NONE', *, *, #14857, .F. ) ;
#5730=VERTEX_POINT ( 'NONE', #15188 ) ;
#5732=ADVANCED_FACE ( 'NONE', ( #8944 ), #4558, .T. ) ;
#5733=EDGE_CURVE ( 'NONE', #14920, #8471, #2924, .T. ) ;
#5735=EDGE_CURVE ( 'NONE', #11666, #14612, #14583, .T. ) ;
#5736=DIRECTION ( 'NONE',  ( -0.8830229359480271656, -0.4693298356057563625, 0.000000000000000000 ) ) ;
#5737=CARTESIAN_POINT ( 'NONE',  ( 59.30716253403183913, -13.12726406102058441, 283.5832628385307999 ) ) ;
#5744=CARTESIAN_POINT ( 'NONE',  ( 0.8220851292435327196, 58.69016442926522359, 112.7772637782949943 ) ) ;
#5745=PLANE ( 'NONE',  #12819 ) ;
#5746=DIRECTION ( 'NONE',  ( -0.9781142164131910732, 0.2080686897406944236, 0.000000000000000000 ) ) ;
#5747=CARTESIAN_POINT ( 'NONE',  ( -68.18670162478832708, -38.41834839689356329, 110.9660488491356887 ) ) ;
#5748=DIRECTION ( 'NONE',  ( 1.000000000000000000, 0.000000000000000000, -0.000000000000000000 ) ) ;
#5752=DIRECTION ( 'NONE',  ( 0.000000000000000000, 0.000000000000000000, 1.000000000000000000 ) ) ;
#5757=EDGE_CURVE ( 'NONE', #16327, #16961, #10888, .T. ) ;
#5759=EDGE_CURVE ( 'NONE', #8471, #13722, #15084, .T. ) ;
#5760=CARTESIAN_POINT ( 'NONE',  ( -12.14914984460759584, -59.51523122377249564, 283.5832628385307999 ) ) ;
#5765=FACE_OUTER_BOUND ( 'NONE', #14718, .T. ) ;
#5768=EDGE_LOOP ( 'NONE', ( #8935, #12879, #6123, #16032 ) ) ;
#5771=VECTOR ( 'NONE', #11203, 1000.000000000000227 ) ;
#5778=CIRCLE ( 'NONE', #12293, 60.74260934110282051 ) ;
#5779=VERTEX_POINT ( 'NONE', #9664 ) ;
#5780=AXIS2_PLACEMENT_3D ( 'NONE', #6780, #18856, #9834 ) ;
#5781=ORIENTED_EDGE ( 'NONE', *, *, #8019, .F. ) ;
#5788=DIRECTION ( 'NONE',  ( 0.9781142164131917394, -0.2080686897406911207, 0.000000000000000000 ) ) ;
#5789=CARTESIAN_POINT ( 'NONE',  ( 0.000000000000000000, 0.000000000000000000, 283.5832628385307999 ) ) ;
#5793=VERTEX_POINT ( 'NONE', #14573 ) ;
#5794=CARTESIAN_POINT ( 'NONE',  ( 41.02350267428969488, 44.79940644582669051, 283.5832628385307999 ) ) ;
#5797=CARTESIAN_POINT ( 'NONE',  ( -59.06449708980196078, -51.36153797460887915, 248.9926560891072143 ) ) ;
#5799=CARTESIAN_POINT ( 'NONE',  ( 28.94886449118905247, -53.40063514825087765, 283.5832628385307999 ) ) ;
#5800=CARTESIAN_POINT ( 'NONE',  ( 36.99387960884163107, -48.17797692984175484, 293.5832628385307999 ) ) ;
#5803=ORIENTED_EDGE ( 'NONE', *, *, #2057, .F. ) ;
#5806=ORIENTED_EDGE ( 'NONE', *, *, #13128, .F. ) ;
#5808=AXIS2_PLACEMENT_3D ( 'NONE', #1410, #12132, #18395 ) ;
#5809=EDGE_CURVE ( 'NONE', #5313, #3073, #2303, .T. ) ;
#5812=DIRECTION ( 'NONE',  ( -0.000000000000000000, -0.000000000000000000, 1.000000000000000000 ) ) ;
#5813=EDGE_LOOP ( 'NONE', ( #9608, #3071, #20007, #13407 ) ) ;
#5814=DIRECTION ( 'NONE',  ( -0.000000000000000000, -0.000000000000000000, 1.000000000000000000 ) ) ;
#5815=CARTESIAN_POINT ( 'NONE',  ( -20.74471755083563806, 59.39925916207565137, 248.9926560891072143 ) ) ;
#5816=VERTEX_POINT ( 'NONE', #8724 ) ;
#5826=VECTOR ( 'NONE', #12894, 1000.000000000000227 ) ;
#5828=DIRECTION ( 'NONE',  ( 0.000000000000000000, 0.000000000000000000, -1.000000000000000000 ) ) ;
#5829=VERTEX_POINT ( 'NONE', #19382 ) ;
#5832=VERTEX_POINT ( 'NONE', #13217 ) ;
#5834=DIRECTION ( 'NONE',  ( -0.5300553768524346454, -0.8479630283625717579, 0.000000000000000000 ) ) ;
#5835=CARTESIAN_POINT ( 'NONE',  ( -23.22718332831480481, -56.12853591711337486, 283.5832628385307999 ) ) ;
#5836=VERTEX_POINT ( 'NONE', #10164 ) ;
#5837=VECTOR ( 'NONE', #15163, 1000.000000000000000 ) ;
#5842=CIRCLE ( 'NONE', #9768, 60.74260934110282051 ) ;
#5843=DIRECTION ( 'NONE',  ( 0.6692498792541753394, 0.7430374143461900838, 0.000000000000000000 ) ) ;
#5845=CARTESIAN_POINT ( 'NONE',  ( -30.53958573130872978, 50.13752642112859803, 110.9660488491356887 ) ) ;
#5846=EDGE_CURVE ( 'NONE', #3935, #14265, #14961, .T. ) ;
#5848=CARTESIAN_POINT ( 'NONE',  ( -29.92423416078134935, 37.80811387934245005, 248.9926560891072143 ) ) ;
#5849=DIRECTION ( 'NONE',  ( -1.000000000000000000, 0.000000000000000000, 0.000000000000000000 ) ) ;
#5851=ORIENTED_EDGE ( 'NONE', *, *, #12260, .F. ) ;
#5852=CARTESIAN_POINT ( 'NONE',  ( 28.94983032429829350, -53.40245231972188833, 293.5832628385307999 ) ) ;
#5854=CONICAL_SURFACE ( 'NONE', #17302, 79.75827554147308263, 0.5305858521701756203 ) ;
#5855=ORIENTED_EDGE ( 'NONE', *, *, #12070, .T. ) ;
#5858=VECTOR ( 'NONE', #16218, 1000.000000000000227 ) ;
#5859=ORIENTED_EDGE ( 'NONE', *, *, #4643, .F. ) ;
#5860=EDGE_LOOP ( 'NONE', ( #13086, #7023, #7441, #11510 ) ) ;
#5862=FACE_BOUND ( 'NONE', #11541, .T. ) ;
#5866=FACE_OUTER_BOUND ( 'NONE', #19611, .T. ) ;
#5867=CARTESIAN_POINT ( 'NONE',  ( 7.948937137877743808, -60.22232964560488000, 283.5832628385307999 ) ) ;
#5868=LINE ( 'NONE', #1148, #10317 ) ;
#5869=FACE_OUTER_BOUND ( 'NONE', #8321, .T. ) ;
#5871=AXIS2_PLACEMENT_3D ( 'NONE', #6707, #351, #3726 ) ;
#5872=ORIENTED_EDGE ( 'NONE', *, *, #11994, .T. ) ;
#5873=CARTESIAN_POINT ( 'NONE',  ( 0.000000000000000000, 0.000000000000000000, 248.9926560891072143 ) ) ;
#5875=EDGE_CURVE ( 'NONE', #3831, #219, #1360, .T. ) ;
#5878=FACE_OUTER_BOUND ( 'NONE', #17518, .T. ) ;
#5880=ORIENTED_EDGE ( 'NONE', *, *, #9134, .T. ) ;
#5884=ORIENTED_EDGE ( 'NONE', *, *, #16393, .F. ) ;
#5885=EDGE_LOOP ( 'NONE', ( #13901, #17723, #12361 ) ) ;
#5886=ADVANCED_FACE ( 'NONE', ( #4533 ), #8825, .F. ) ;
#5887=VERTEX_POINT ( 'NONE', #13728 ) ;
#5889=CARTESIAN_POINT ( 'NONE',  ( 38.78191089773071809, -44.07268132743684674, 132.4711112102474146 ) ) ;
#5890=LINE ( 'NONE', #7312, #4862 ) ;
#5892=CARTESIAN_POINT ( 'NONE',  ( 0.000000000000000000, 0.000000000000000000, 132.4711112102474146 ) ) ;
#5893=DIRECTION ( 'NONE',  ( 0.000000000000000000, 0.000000000000000000, -1.000000000000000000 ) ) ;
#5897=FACE_OUTER_BOUND ( 'NONE', #20126, .T. ) ;
#5899=AXIS2_PLACEMENT_3D ( 'NONE', #948, #19572, #14962 ) ;
#5900=ADVANCED_FACE ( 'NONE', ( #20076 ), #16610, .F. ) ;
#5904=EDGE_CURVE ( 'NONE', #12139, #15302, #8922, .T. ) ;
#5911=VERTEX_POINT ( 'NONE', #7692 ) ;
#5914=VECTOR ( 'NONE', #2232, 1000.000000000000000 ) ;
#5915=EDGE_CURVE ( 'NONE', #7860, #12583, #5868, .T. ) ;
#5916=ORIENTED_EDGE ( 'NONE', *, *, #11954, .F. ) ;
#5920=CARTESIAN_POINT ( 'NONE',  ( 0.000000000000000000, 0.000000000000000000, 283.5832628385307999 ) ) ;
#5922=ORIENTED_EDGE ( 'NONE', *, *, #340, .T. ) ;
#5924=CARTESIAN_POINT ( 'NONE',  ( 3.123743752084087610, -4.811834253409037920, 293.5832628385307999 ) ) ;
#5926=CARTESIAN_POINT ( 'NONE',  ( 47.56406379474552182, 37.78325588002191893, 293.5832628385307999 ) ) ;
#5927=DIRECTION ( 'NONE',  ( 0.1736481776669172583, 0.9848077530122103518, 0.000000000000000000 ) ) ;
#5928=EDGE_CURVE ( 'NONE', #48, #2962, #133, .T. ) ;
#5930=VECTOR ( 'NONE', #20073, 1000.000000000000000 ) ;
#5932=LINE ( 'NONE', #10608, #3509 ) ;
#5934=CIRCLE ( 'NONE', #8540, 60.74260934110282051 ) ;
#5937=ORIENTED_EDGE ( 'NONE', *, *, #6295, .T. ) ;
#5939=LINE ( 'NONE', #15330, #16449 ) ;
#5940=ORIENTED_EDGE ( 'NONE', *, *, #6243, .T. ) ;
#5944=LINE ( 'NONE', #5537, #17321 ) ;
#5948=FACE_OUTER_BOUND ( 'NONE', #18166, .T. ) ;
#5952=CARTESIAN_POINT ( 'NONE',  ( 0.000000000000000000, 0.000000000000000000, 248.9926560891072143 ) ) ;
#5956=FACE_OUTER_BOUND ( 'NONE', #18725, .T. ) ;
#5957=DIRECTION ( 'NONE',  ( -0.000000000000000000, -0.000000000000000000, 1.000000000000000000 ) ) ;
#5958=ORIENTED_EDGE ( 'NONE', *, *, #13101, .T. ) ;
#5959=ORIENTED_EDGE ( 'NONE', *, *, #13228, .T. ) ;
#5960=AXIS2_PLACEMENT_3D ( 'NONE', #16819, #4756, #10978 ) ;
#5962=VERTEX_POINT ( 'NONE', #3107 ) ;
#5963=FACE_BOUND ( 'NONE', #5964, .T. ) ;
#5964=EDGE_LOOP ( 'NONE', ( #7932, #18960, #19196 ) ) ;
#5965=VECTOR ( 'NONE', #2380, 999.9999999999998863 ) ;
#5966=CARTESIAN_POINT ( 'NONE',  ( 28.06680738835026290, -53.87178215532764369, 293.5832628385307999 ) ) ;
#5967=LINE ( 'NONE', #19967, #4362 ) ;
#5970=DIRECTION ( 'NONE',  ( 0.000000000000000000, 0.000000000000000000, 1.000000000000000000 ) ) ;
#5971=FACE_OUTER_BOUND ( 'NONE', #2488, .T. ) ;
#5973=DIRECTION ( 'NONE',  ( 1.000000000000000000, 0.000000000000000000, 0.000000000000000000 ) ) ;
#5976=VECTOR ( 'NONE', #18202, 1000.000000000000000 ) ;
#5978=LINE ( 'NONE', #10560, #2338 ) ;
#5983=FACE_OUTER_BOUND ( 'NONE', #14130, .T. ) ;
#5985=ORIENTED_EDGE ( 'NONE', *, *, #17890, .T. ) ;
#5989=VECTOR ( 'NONE', #19966, 1000.000000000000000 ) ;
#5990=ORIENTED_EDGE ( 'NONE', *, *, #13629, .F. ) ;
#5994=CARTESIAN_POINT ( 'NONE',  ( 79.75827554147308263, 0.000000000000000000, 132.4711112102474146 ) ) ;
#5997=DIRECTION ( 'NONE',  ( 1.000000000000000000, 0.000000000000000000, 0.000000000000000000 ) ) ;
#5998=FACE_OUTER_BOUND ( 'NONE', #6522, .T. ) ;
#5999=EDGE_LOOP ( 'NONE', ( #15306, #8570, #6730 ) ) ;
#6000=LINE ( 'NONE', #9569, #7797 ) ;
#6001=DIRECTION ( 'NONE',  ( 1.000000000000000000, 3.491481338843133355E-15, 0.000000000000000000 ) ) ;
#6003=CARTESIAN_POINT ( 'NONE',  ( 19.23677882349201695, -57.61823435390814296, 293.5832628385307999 ) ) ;
#6007=CYLINDRICAL_SURFACE ( 'NONE', #19493, 62.91752772691707207 ) ;
#6009=VERTEX_POINT ( 'NONE', #18970 ) ;
#6021=FACE_OUTER_BOUND ( 'NONE', #3658, .T. ) ;
#6022=DIRECTION ( 'NONE',  ( -0.3420201433256630508, -0.9396926207859104263, -0.000000000000000000 ) ) ;
#6023=EDGE_LOOP ( 'NONE', ( #16426, #16726, #343, #3323 ) ) ;
#6024=DIRECTION ( 'NONE',  ( -0.000000000000000000, -0.000000000000000000, 1.000000000000000000 ) ) ;
#6025=FACE_OUTER_BOUND ( 'NONE', #770, .T. ) ;
#6026=VERTEX_POINT ( 'NONE', #1569 ) ;
#6029=AXIS2_PLACEMENT_3D ( 'NONE', #16396, #2376, #5445 ) ;
#6030=CARTESIAN_POINT ( 'NONE',  ( 0.000000000000000000, 0.000000000000000000, 132.4711112102474146 ) ) ;
#6033=FACE_OUTER_BOUND ( 'NONE', #6573, .T. ) ;
#6034=DIRECTION ( 'NONE',  ( 0.9848077530122104628, -0.1736481776669172861, 0.000000000000000000 ) ) ;
#6035=CARTESIAN_POINT ( 'NONE',  ( -36.99387960884161686, 48.17797692984174773, 293.5832628385307999 ) ) ;
#6038=LINE ( 'NONE', #15225, #17765 ) ;
#6039=VERTEX_POINT ( 'NONE', #14045 ) ;
#6040=EDGE_LOOP ( 'NONE', ( #11606, #3123, #3055, #13266 ) ) ;
#6041=DIRECTION ( 'NONE',  ( -0.000000000000000000, -0.000000000000000000, 1.000000000000000000 ) ) ;
#6042=EDGE_CURVE ( 'NONE', #19700, #18461, #1772, .T. ) ;
#6043=AXIS2_PLACEMENT_3D ( 'NONE', #19530, #2351, #8584 ) ;
#6044=ORIENTED_EDGE ( 'NONE', *, *, #8529, .T. ) ;
#6046=CARTESIAN_POINT ( 'NONE',  ( -5.590028426173819120, -1.289614712049182987, 283.5832628385307999 ) ) ;
#6047=LINE ( 'NONE', #10731, #2724 ) ;
#6050=DIRECTION ( 'NONE',  ( 1.000000000000000000, 0.000000000000000000, 0.000000000000000000 ) ) ;
#6051=EDGE_CURVE ( 'NONE', #2942, #11211, #2252, .T. ) ;
#6053=VECTOR ( 'NONE', #1950, 1000.000000000000114 ) ;
#6055=DIRECTION ( 'NONE',  ( 0.8830229359480271656, 0.4693298356057563625, 0.000000000000000000 ) ) ;
#6057=AXIS2_PLACEMENT_3D ( 'NONE', #6030, #16760, #2751 ) ;
#6061=ORIENTED_EDGE ( 'NONE', *, *, #6591, .F. ) ;
#6065=ORIENTED_EDGE ( 'NONE', *, *, #8721, .T. ) ;
#6069=DIRECTION ( 'NONE',  ( 0.2080686897406943681, 0.9781142164131909622, 0.000000000000000000 ) ) ;
#6071=LINE ( 'NONE', #9543, #4679 ) ;
#6075=DIRECTION ( 'NONE',  ( -0.7881095627315619634, -0.6155349844899687950, 0.000000000000000000 ) ) ;
#6077=VECTOR ( 'NONE', #13144, 1000.000000000000227 ) ;
#6082=VECTOR ( 'NONE', #15424, 1000.000000000000114 ) ;
#6088=VECTOR ( 'NONE', #15603, 1000.000000000000114 ) ;
#6089=ORIENTED_EDGE ( 'NONE', *, *, #7902, .T. ) ;
#6092=EDGE_CURVE ( 'NONE', #13307, #6254, #8005, .T. ) ;
#6093=VECTOR ( 'NONE', #1341, 999.9999999999998863 ) ;
#6100=CARTESIAN_POINT ( 'NONE',  ( 1.379293853801755176, -58.69016442926522359, 132.4711112102474146 ) ) ;
#6102=CARTESIAN_POINT ( 'NONE',  ( 39.84224160888901167, 67.36461649554546227, 248.9926560891072143 ) ) ;
#6103=CARTESIAN_POINT ( 'NONE',  ( -38.41834839689332171, 68.18670162478844077, 248.9926560891072143 ) ) ;
#6104=DIRECTION ( 'NONE',  ( 0.6427876096865379196, 0.7660444431189792347, 0.000000000000000000 ) ) ;
#6105=VECTOR ( 'NONE', #6732, 1000.000000000000000 ) ;
#6106=CIRCLE ( 'NONE', #20147, 60.74260934110282051 ) ;
#6107=ADVANCED_FACE ( 'NONE', ( #229 ), #9919, .T. ) ;
#6110=VERTEX_POINT ( 'NONE', #7053 ) ;
#6111=ADVANCED_FACE ( 'NONE', ( #2347 ), #2447, .F. ) ;
#6112=CIRCLE ( 'NONE', #5459, 62.91752772691707207 ) ;
#6116=LINE ( 'NONE', #7938, #8282 ) ;
#6118=ORIENTED_EDGE ( 'NONE', *, *, #19057, .F. ) ;
#6119=EDGE_CURVE ( 'NONE', #2886, #10466, #5778, .T. ) ;
#6120=LINE ( 'NONE', #12335, #8446 ) ;
#6122=CARTESIAN_POINT ( 'NONE',  ( -78.26059000578311498, 0.8220851292432594937, 248.9926560891072143 ) ) ;
#6123=ORIENTED_EDGE ( 'NONE', *, *, #17109, .T. ) ;
#6126=EDGE_LOOP ( 'NONE', ( #14321, #7042, #6699, #18204 ) ) ;
#6130=CARTESIAN_POINT ( 'NONE',  ( 55.62246070845780110, -18.77710619359098132, 111.4180192758974499 ) ) ;
#6131=CARTESIAN_POINT ( 'NONE',  ( 53.86996498385654064, 28.06584155524121016, 283.5832628385307999 ) ) ;
#6133=LINE ( 'NONE', #18197, #16265 ) ;
#6134=EDGE_CURVE ( 'NONE', #17581, #19621, #19821, .T. ) ;
#6140=ORIENTED_EDGE ( 'NONE', *, *, #15206, .T. ) ;
#6142=ORIENTED_EDGE ( 'NONE', *, *, #5140, .T. ) ;
#6143=LINE ( 'NONE', #19939, #11696 ) ;
#6145=AXIS2_PLACEMENT_3D ( 'NONE', #19580, #2406, #857 ) ;
#6146=EDGE_LOOP ( 'NONE', ( #15150, #767, #17767, #12532 ) ) ;
#6147=LINE ( 'NONE', #12366, #5547 ) ;
#6148=ADVANCED_FACE ( 'NONE', ( #1000 ), #10209, .T. ) ;
#6150=ORIENTED_EDGE ( 'NONE', *, *, #8297, .T. ) ;
#6151=DIRECTION ( 'NONE',  ( -0.000000000000000000, -0.000000000000000000, 1.000000000000000000 ) ) ;
#6152=CARTESIAN_POINT ( 'NONE',  ( 0.000000000000000000, 0.000000000000000000, 283.5832628385307999 ) ) ;
#6158=CARTESIAN_POINT ( 'NONE',  ( -12.14957802882752524, -59.51724408343569905, 293.5832628385307999 ) ) ;
#6159=EDGE_CURVE ( 'NONE', #8624, #15754, #14819, .T. ) ;
#6160=DIRECTION ( 'NONE',  ( -0.6427876096865328126, -0.7660444431189835646, 0.000000000000000000 ) ) ;
#6162=DIRECTION ( 'NONE',  ( -1.000000000000000000, 0.000000000000000000, -0.000000000000000000 ) ) ;
#6165=EDGE_CURVE ( 'NONE', #15505, #16710, #19622, .T. ) ;
#6168=ORIENTED_EDGE ( 'NONE', *, *, #7875, .F. ) ;
#6169=ORIENTED_EDGE ( 'NONE', *, *, #348, .F. ) ;
#6171=VECTOR ( 'NONE', #2539, 1000.000000000000000 ) ;
#6172=VECTOR ( 'NONE', #1112, 1000.000000000000000 ) ;
#6174=VECTOR ( 'NONE', #11552, 1000.000000000000000 ) ;
#6177=FACE_BOUND ( 'NONE', #8793, .T. ) ;
#6178=ORIENTED_EDGE ( 'NONE', *, *, #1420, .T. ) ;
#6180=DIRECTION ( 'NONE',  ( 0.03505990758545895342, 0.9993852124581886764, 0.000000000000000000 ) ) ;
#6184=DIRECTION ( 'NONE',  ( 0.3420201433256694901, -0.9396926207859082059, -0.000000000000000000 ) ) ;
#6185=CARTESIAN_POINT ( 'NONE',  ( -58.63718168490499494, -22.81000261549349162, 132.4711112102474146 ) ) ;
#6189=DIRECTION ( 'NONE',  ( 0.000000000000000000, 0.000000000000000000, -1.000000000000000000 ) ) ;
#6193=CIRCLE ( 'NONE', #628, 62.91752772691707207 ) ;
#6196=LINE ( 'NONE', #15382, #7266 ) ;
#6198=EDGE_LOOP ( 'NONE', ( #3268, #14054, #11908, #2381 ) ) ;
#6201=AXIS2_PLACEMENT_3D ( 'NONE', #8229, #18995, #3636 ) ;
#6203=LINE ( 'NONE', #6403, #20067 ) ;
#6205=VERTEX_POINT ( 'NONE', #16663 ) ;
#6207=DIRECTION ( 'NONE',  ( -0.9271237148521536131, 0.3747554100459959958, 0.000000000000000000 ) ) ;
#6208=EDGE_LOOP ( 'NONE', ( #10001, #1526, #4594, #15078 ) ) ;
#6210=CARTESIAN_POINT ( 'NONE',  ( -2.629250726500700353, -60.68567895461850981, 293.5832628385307999 ) ) ;
#6213=CARTESIAN_POINT ( 'NONE',  ( 60.08127757648377099, 8.938941455415205795, 283.5832628385307999 ) ) ;
#6217=ORIENTED_EDGE ( 'NONE', *, *, #16687, .T. ) ;
#6218=EDGE_CURVE ( 'NONE', #2611, #12822, #707, .T. ) ;
#6219=ORIENTED_EDGE ( 'NONE', *, *, #14487, .T. ) ;
#6224=PLANE ( 'NONE',  #15230 ) ;
#6226=VECTOR ( 'NONE', #7550, 1000.000000000000227 ) ;
#6227=EDGE_CURVE ( 'NONE', #11122, #8663, #18498, .T. ) ;
#6228=DIRECTION ( 'NONE',  ( 0.7430374143461878633, -0.6692498792541777819, 0.000000000000000000 ) ) ;
#6233=DIRECTION ( 'NONE',  ( -0.000000000000000000, -0.000000000000000000, 1.000000000000000000 ) ) ;
#6234=ORIENTED_EDGE ( 'NONE', *, *, #17892, .F. ) ;
#6238=CARTESIAN_POINT ( 'NONE',  ( -59.30716253403183202, 13.12726406102060217, 283.5832628385307999 ) ) ;
#6239=PLANE ( 'NONE',  #7748 ) ;
#6243=EDGE_CURVE ( 'NONE', #3335, #720, #13988, .T. ) ;
#6244=EDGE_CURVE ( 'NONE', #18601, #321, #7545, .T. ) ;
#6245=PLANE ( 'NONE',  #19396 ) ;
#6246=VERTEX_POINT ( 'NONE', #4377 ) ;
#6248=ORIENTED_EDGE ( 'NONE', *, *, #7466, .F. ) ;
#6249=DIRECTION ( 'NONE',  ( 1.000000000000000000, 0.000000000000000000, 0.000000000000000000 ) ) ;
#6250=ORIENTED_EDGE ( 'NONE', *, *, #493, .T. ) ;
#6252=EDGE_CURVE ( 'NONE', #18601, #1451, #10814, .T. ) ;
#6254=VERTEX_POINT ( 'NONE', #7646 ) ;
#6257=PLANE ( 'NONE',  #15556 ) ;
#6260=PLANE ( 'NONE',  #4583 ) ;
#6261=PLANE ( 'NONE',  #9294 ) ;
#6263=CARTESIAN_POINT ( 'NONE',  ( 8.938941455415006843, -60.08127757648380651, 283.5832628385307999 ) ) ;
#6267=VERTEX_POINT ( 'NONE', #3059 ) ;
#6270=EDGE_CURVE ( 'NONE', #18758, #13055, #20233, .T. ) ;
#6271=CARTESIAN_POINT ( 'NONE',  ( 68.18670162478807129, 38.41834839689403935, 132.4711112102474146 ) ) ;
#6272=DIRECTION ( 'NONE',  ( -0.9271237148521536131, 0.3747554100459959958, 0.000000000000000000 ) ) ;
#6274=ORIENTED_EDGE ( 'NONE', *, *, #12340, .F. ) ;
#6275=EDGE_LOOP ( 'NONE', ( #12357, #11702, #1808, #18130 ) ) ;
#6279=LINE ( 'NONE', #4737, #19813 ) ;
#6282=CARTESIAN_POINT ( 'NONE',  ( 48.17959877923549072, 36.99514631729036296, 293.5832628385307999 ) ) ;
#6283=CARTESIAN_POINT ( 'NONE',  ( -1.629937663769596368, -60.72279549541552512, 293.5832628385307999 ) ) ;
#6284=DIRECTION ( 'NONE',  ( -0.000000000000000000, -0.000000000000000000, 1.000000000000000000 ) ) ;
#6291=LINE ( 'NONE', #7597, #5279 ) ;
#6292=CARTESIAN_POINT ( 'NONE',  ( -28.06584155524100765, 53.86996498385663301, 283.5832628385307999 ) ) ;
#6294=ORIENTED_EDGE ( 'NONE', *, *, #6270, .F. ) ;
#6295=EDGE_CURVE ( 'NONE', #8175, #9508, #14503, .T. ) ;
#6296=PLANE ( 'NONE',  #5960 ) ;
#6298=ORIENTED_EDGE ( 'NONE', *, *, #19958, .T. ) ;
#6303=DIRECTION ( 'NONE',  ( 0.000000000000000000, 0.000000000000000000, 1.000000000000000000 ) ) ;
#6305=DIRECTION ( 'NONE',  ( -0.9902903945359624593, -0.1390141521205945918, 0.000000000000000000 ) ) ;
#6306=VECTOR ( 'NONE', #16096, 1000.000000000000341 ) ;
#6307=CARTESIAN_POINT ( 'NONE',  ( 41.02212542604613077, 44.79787735033405482, 283.5832628385307999 ) ) ;
#6308=ADVANCED_FACE ( 'NONE', ( #16044 ), #5003, .T. ) ;
#6309=DIRECTION ( 'NONE',  ( 1.000000000000000000, 0.000000000000000000, 0.000000000000000000 ) ) ;
#6311=FACE_OUTER_BOUND ( 'NONE', #18792, .T. ) ;
#6312=VECTOR ( 'NONE', #2478, 1000.000000000000114 ) ;
#6314=FACE_OUTER_BOUND ( 'NONE', #15633, .T. ) ;
#6318=VERTEX_POINT ( 'NONE', #6540 ) ;
#6319=AXIS2_PLACEMENT_3D ( 'NONE', #15251, #3193, #15460 ) ;
#6321=ORIENTED_EDGE ( 'NONE', *, *, #7764, .F. ) ;
#6322=EDGE_LOOP ( 'NONE', ( #4035, #10341, #17262, #11083 ) ) ;
#6323=CARTESIAN_POINT ( 'NONE',  ( 67.08601213326539892, 40.32479851956841088, 132.4711112102474146 ) ) ;
#6324=VERTEX_POINT ( 'NONE', #2031 ) ;
#6325=DIRECTION ( 'NONE',  ( -0.8660254037844328234, -0.5000000000000101030, 0.000000000000000000 ) ) ;
#6326=VECTOR ( 'NONE', #14293, 1000.000000000000114 ) ;
#6332=DIRECTION ( 'NONE',  ( -0.000000000000000000, -0.000000000000000000, 1.000000000000000000 ) ) ;
#6333=ORIENTED_EDGE ( 'NONE', *, *, #6968, .F. ) ;
#6334=CARTESIAN_POINT ( 'NONE',  ( 30.05702882063027914, 50.41613078340812848, 248.9926560891072143 ) ) ;
#6339=VECTOR ( 'NONE', #19204, 1000.000000000000000 ) ;
#6343=DIRECTION ( 'NONE',  ( -0.000000000000000000, -0.000000000000000000, 1.000000000000000000 ) ) ;
#6346=VERTEX_POINT ( 'NONE', #285 ) ;
#6347=LINE ( 'NONE', #12566, #7941 ) ;
#6348=VERTEX_POINT ( 'NONE', #12761 ) ;
#6354=DIRECTION ( 'NONE',  ( 0.000000000000000000, 0.000000000000000000, 1.000000000000000000 ) ) ;
#6355=EDGE_CURVE ( 'NONE', #20199, #10313, #19216, .T. ) ;
#6356=VECTOR ( 'NONE', #19590, 1000.000000000000114 ) ;
#6358=DIRECTION ( 'NONE',  ( -0.1390141521205912334, 0.9902903945359629034, 0.000000000000000000 ) ) ;
#6360=DIRECTION ( 'NONE',  ( 0.6427876096865379196, 0.7660444431189792347, 0.000000000000000000 ) ) ;
#6361=DIRECTION ( 'NONE',  ( 0.9511061040868794558, 0.3088643371590157338, 0.000000000000000000 ) ) ;
#6363=DIRECTION ( 'NONE',  ( 0.000000000000000000, 0.000000000000000000, 1.000000000000000000 ) ) ;
#6365=EDGE_LOOP ( 'NONE', ( #18082, #10976, #18465, #16950 ) ) ;
#6366=EDGE_CURVE ( 'NONE', #10035, #19638, #19316, .T. ) ;
#6371=AXIS2_PLACEMENT_3D ( 'NONE', #12886, #8284, #9819 ) ;
#6372=ORIENTED_EDGE ( 'NONE', *, *, #19988, .T. ) ;
#6373=EDGE_CURVE ( 'NONE', #937, #9274, #15840, .T. ) ;
#6374=EDGE_LOOP ( 'NONE', ( #1516, #12435, #651, #7838 ) ) ;
#6375=ORIENTED_EDGE ( 'NONE', *, *, #16547, .T. ) ;
#6376=LINE ( 'NONE', #1560, #7174 ) ;
#6378=ORIENTED_EDGE ( 'NONE', *, *, #1111, .F. ) ;
#6379=VECTOR ( 'NONE', #7269, 1000.000000000000000 ) ;
#6380=DIRECTION ( 'NONE',  ( 0.4693298356057531984, -0.8830229359480288309, 0.000000000000000000 ) ) ;
#6382=LINE ( 'NONE', #10964, #7999 ) ;
#6383=EDGE_CURVE ( 'NONE', #11666, #20199, #15942, .T. ) ;
#6389=DIRECTION ( 'NONE',  ( 0.000000000000000000, 0.000000000000000000, 1.000000000000000000 ) ) ;
#6390=DIRECTION ( 'NONE',  ( 0.7881095627315598540, 0.6155349844899715706, 0.000000000000000000 ) ) ;
#6393=ORIENTED_EDGE ( 'NONE', *, *, #13851, .F. ) ;
#6397=AXIS2_PLACEMENT_3D ( 'NONE', #1739, #11042, #9518 ) ;
#6398=EDGE_CURVE ( 'NONE', #5054, #1479, #14601, .T. ) ;
#6400=ORIENTED_EDGE ( 'NONE', *, *, #3384, .F. ) ;
#6402=ADVANCED_FACE ( 'NONE', ( #13347 ), #8557, .F. ) ;
#6403=CARTESIAN_POINT ( 'NONE',  ( -39.84224160888947353, -67.36461649554519227, 248.9926560891072143 ) ) ;
#6405=VECTOR ( 'NONE', #12468, 1000.000000000000114 ) ;
#6409=PLANE ( 'NONE',  #10104 ) ;
#6411=DIRECTION ( 'NONE',  ( -0.000000000000000000, -0.000000000000000000, 1.000000000000000000 ) ) ;
#6413=ADVANCED_FACE ( 'NONE', ( #19798 ), #2329, .F. ) ;
#6414=CARTESIAN_POINT ( 'NONE',  ( 28.06584155524102187, -53.86996498385662591, 283.5832628385307999 ) ) ;
#6418=EDGE_CURVE ( 'NONE', #13999, #18902, #688, .T. ) ;
#6420=ORIENTED_EDGE ( 'NONE', *, *, #16379, .T. ) ;
#6422=ORIENTED_EDGE ( 'NONE', *, *, #14917, .T. ) ;
#6424=ORIENTED_EDGE ( 'NONE', *, *, #15760, .F. ) ;
#6426=ORIENTED_EDGE ( 'NONE', *, *, #14342, .F. ) ;
#6427=DIRECTION ( 'NONE',  ( 0.9396926207859068736, 0.3420201433256725987, 0.000000000000000000 ) ) ;
#6428=CARTESIAN_POINT ( 'NONE',  ( 7.948651060879040386, -60.22029172860440127, 283.5832628385307999 ) ) ;
#6436=ORIENTED_EDGE ( 'NONE', *, *, #9613, .T. ) ;
#6437=CIRCLE ( 'NONE', #8693, 60.74260934110282051 ) ;
#6440=FACE_OUTER_BOUND ( 'NONE', #16482, .T. ) ;
#6443=DIRECTION ( 'NONE',  ( 1.000000000000000000, 0.000000000000000000, 0.000000000000000000 ) ) ;
#6445=ORIENTED_EDGE ( 'NONE', *, *, #6884, .F. ) ;
#6446=DIRECTION ( 'NONE',  ( -0.7660444431189726844, -0.6427876096865456912, 0.000000000000000000 ) ) ;
#6453=DIRECTION ( 'NONE',  ( 1.000000000000000000, 0.000000000000000000, 0.000000000000000000 ) ) ;
#6454=VECTOR ( 'NONE', #8587, 1000.000000000000000 ) ;
#6455=DIRECTION ( 'NONE',  ( -0.9396926207859057634, -0.3420201433256757073, 0.000000000000000000 ) ) ;
#6456=VECTOR ( 'NONE', #10266, 1000.000000000000000 ) ;
#6457=ORIENTED_EDGE ( 'NONE', *, *, #17062, .F. ) ;
#6458=CARTESIAN_POINT ( 'NONE',  ( 36.66871011346380982, 45.84586732611875703, 132.4711112102474146 ) ) ;
#6460=DIRECTION ( 'NONE',  ( 0.3420201433256568335, 0.9396926207859126468, 0.000000000000000000 ) ) ;
#6461=PLANE ( 'NONE',  #10921 ) ;
#6464=CARTESIAN_POINT ( 'NONE',  ( 21.36933070621763164, -54.67896814532648619, 111.4180192758973362 ) ) ;
#6465=DIRECTION ( 'NONE',  ( 1.000000000000000000, 0.000000000000000000, 0.000000000000000000 ) ) ;
#6466=CARTESIAN_POINT ( 'NONE',  ( 62.91752772691707207, 0.000000000000000000, 83.57543755549745867 ) ) ;
#6467=ORIENTED_EDGE ( 'NONE', *, *, #12717, .T. ) ;
#6469=LINE ( 'NONE', #14536, #2244 ) ;
#6473=ADVANCED_FACE ( 'NONE', ( #14699 ), #10286, .T. ) ;
#6475=ORIENTED_EDGE ( 'NONE', *, *, #13910, .F. ) ;
#6477=ORIENTED_EDGE ( 'NONE', *, *, #8045, .F. ) ;
#6478=DIRECTION ( 'NONE',  ( -0.4693298356057531429, 0.8830229359480288309, 0.000000000000000000 ) ) ;
#6482=DIRECTION ( 'NONE',  ( 0.4974449862757516216, 0.000000000000000000, 0.8674955248467378643 ) ) ;
#6484=AXIS2_PLACEMENT_3D ( 'NONE', #2123, #14693, #680 ) ;
#6486=EDGE_CURVE ( 'NONE', #3220, #12611, #14890, .T. ) ;
#6488=CARTESIAN_POINT ( 'NONE',  ( 60.47951622432751151, 49.67518383744852883, 110.7293897666001214 ) ) ;
#6490=DIRECTION ( 'NONE',  ( 1.000000000000000000, 0.000000000000000000, 0.000000000000000000 ) ) ;
#6496=AXIS2_PLACEMENT_3D ( 'NONE', #2149, #10113, #1837 ) ;
#6497=VECTOR ( 'NONE', #8722, 1000.000000000000000 ) ;
#6498=EDGE_CURVE ( 'NONE', #1969, #3773, #13148, .T. ) ;
#6499=AXIS2_PLACEMENT_3D ( 'NONE', #18955, #17620, #14439 ) ;
#6500=VERTEX_POINT ( 'NONE', #17879 ) ;
#6501=ORIENTED_EDGE ( 'NONE', *, *, #9616, .F. ) ;
#6505=ADVANCED_FACE ( 'NONE', ( #3851 ), #782, .T. ) ;
#6509=CARTESIAN_POINT ( 'NONE',  ( 0.000000000000000000, 0.000000000000000000, 132.4711112102474146 ) ) ;
#6510=VECTOR ( 'NONE', #1625, 1000.000000000000227 ) ;
#6512=DIRECTION ( 'NONE',  ( 0.7660444431189792347, -0.6427876096865379196, -0.000000000000000000 ) ) ;
#6513=AXIS2_PLACEMENT_3D ( 'NONE', #8328, #14473, #255 ) ;
#6514=CARTESIAN_POINT ( 'NONE',  ( -67.08601213326564050, -40.32479851956793482, 248.9926560891072143 ) ) ;
#6516=DIRECTION ( 'NONE',  ( -0.000000000000000000, -0.000000000000000000, 1.000000000000000000 ) ) ;
#6517=DIRECTION ( 'NONE',  ( 0.03505990758545895342, 0.9993852124581886764, 0.000000000000000000 ) ) ;
#6518=ORIENTED_EDGE ( 'NONE', *, *, #4898, .F. ) ;
#6521=ORIENTED_EDGE ( 'NONE', *, *, #17186, .T. ) ;
#6522=EDGE_LOOP ( 'NONE', ( #12615, #11801, #4797, #2709 ) ) ;
#6526=CIRCLE ( 'NONE', #13336, 60.74260934110282051 ) ;
#6527=ORIENTED_EDGE ( 'NONE', *, *, #11158, .T. ) ;
#6528=CARTESIAN_POINT ( 'NONE',  ( 51.77076963420846312, -31.77187437101485656, 283.5832628385307999 ) ) ;
#6529=VERTEX_POINT ( 'NONE', #16640 ) ;
#6531=DIRECTION ( 'NONE',  ( 1.000000000000000000, 0.000000000000000000, 0.000000000000000000 ) ) ;
#6532=CARTESIAN_POINT ( 'NONE',  ( -31.77187437101503775, -51.77076963420834943, 283.5832628385307999 ) ) ;
#6537=DIRECTION ( 'NONE',  ( 0.000000000000000000, 0.000000000000000000, 1.000000000000000000 ) ) ;
#6538=EDGE_CURVE ( 'NONE', #18899, #12185, #8752, .T. ) ;
#6540=CARTESIAN_POINT ( 'NONE',  ( -13.12726406102078336, -59.30716253403180360, 293.5832628385307999 ) ) ;
#6541=CYLINDRICAL_SURFACE ( 'NONE', #6838, 62.91752772691707207 ) ;
#6545=DIRECTION ( 'NONE',  ( -0.7660444431189813441, 0.6427876096865353661, 0.000000000000000000 ) ) ;
#6546=CARTESIAN_POINT ( 'NONE',  ( 0.000000000000000000, 0.000000000000000000, 293.5832628385307999 ) ) ;
#6547=PLANE ( 'NONE',  #4804 ) ;
#6549=CARTESIAN_POINT ( 'NONE',  ( 76.92888220842486646, -14.39940464655733976, 248.9926560891072143 ) ) ;
#6558=VERTEX_POINT ( 'NONE', #12221 ) ;
#6559=EDGE_CURVE ( 'NONE', #6529, #19079, #1288, .T. ) ;
#6562=PLANE ( 'NONE',  #19959 ) ;
#6564=ADVANCED_FACE ( 'NONE', ( #5897 ), #18581, .F. ) ;
#6565=CARTESIAN_POINT ( 'NONE',  ( 30.25670013172214468, 55.16472960512381718, 132.4711112102474146 ) ) ;
#6567=ORIENTED_EDGE ( 'NONE', *, *, #6538, .T. ) ;
#6573=EDGE_LOOP ( 'NONE', ( #673, #1068, #223, #1503 ) ) ;
#6574=CARTESIAN_POINT ( 'NONE',  ( 0.000000000000000000, 0.000000000000000000, 293.5832628385307999 ) ) ;
#6576=ORIENTED_EDGE ( 'NONE', *, *, #13406, .F. ) ;
#6578=ORIENTED_EDGE ( 'NONE', *, *, #11221, .F. ) ;
#6581=LINE ( 'NONE', #10756, #16967 ) ;
#6582=AXIS2_PLACEMENT_3D ( 'NONE', #10528, #15344, #6055 ) ;
#6586=CARTESIAN_POINT ( 'NONE',  ( 36.66871011346380982, 45.84586732611875703, 110.7293897666001214 ) ) ;
#6587=CARTESIAN_POINT ( 'NONE',  ( 73.25972925305627825, -27.53920554013664912, 248.9926560891072143 ) ) ;
#6589=CARTESIAN_POINT ( 'NONE',  ( -13.12769224524071277, -59.30917539369501412, 283.5832628385307999 ) ) ;
#6591=EDGE_CURVE ( 'NONE', #15414, #16327, #9264, .T. ) ;
#6592=CARTESIAN_POINT ( 'NONE',  ( 59.39925916207545242, 20.74471755083624203, 248.9926560891072143 ) ) ;
#6600=ORIENTED_EDGE ( 'NONE', *, *, #13074, .T. ) ;
#6601=ORIENTED_EDGE ( 'NONE', *, *, #6622, .F. ) ;
#6603=CYLINDRICAL_SURFACE ( 'NONE', #9618, 17.50000000000001066 ) ;
#6604=CARTESIAN_POINT ( 'NONE',  ( 0.7000608949449915741, 5.693982670708925831, 293.5832628385307999 ) ) ;
#6605=CARTESIAN_POINT ( 'NONE',  ( -40.32479851956768613, 67.08601213326579682, 110.9660488491356887 ) ) ;
#6606=EDGE_CURVE ( 'NONE', #4738, #11620, #16941, .T. ) ;
#6607=ORIENTED_EDGE ( 'NONE', *, *, #3616, .T. ) ;
#6609=LINE ( 'NONE', #16116, #7911 ) ;
#6610=DIRECTION ( 'NONE',  ( 0.7660444431189858960, -0.6427876096865300370, 0.000000000000000000 ) ) ;
#6611=VECTOR ( 'NONE', #13223, 1000.000000000000000 ) ;
#6613=CARTESIAN_POINT ( 'NONE',  ( 4.581103194069847007, -3.453261854572897693, 293.5832628385307999 ) ) ;
#6614=ORIENTED_EDGE ( 'NONE', *, *, #16884, .T. ) ;
#6617=ORIENTED_EDGE ( 'NONE', *, *, #19589, .F. ) ;
#6620=ADVANCED_FACE ( 'NONE', ( #8948 ), #15507, .T. ) ;
#6621=EDGE_LOOP ( 'NONE', ( #163, #5630, #8810, #12591 ) ) ;
#6622=EDGE_CURVE ( 'NONE', #6500, #10158, #15608, .T. ) ;
#6623=DIRECTION ( 'NONE',  ( -0.000000000000000000, -0.000000000000000000, 1.000000000000000000 ) ) ;
#6624=AXIS2_PLACEMENT_3D ( 'NONE', #18562, #15701, #4546 ) ;
#6625=AXIS2_PLACEMENT_3D ( 'NONE', #1027, #10332, #7273 ) ;
#6626=VERTEX_POINT ( 'NONE', #4350 ) ;
#6627=FACE_OUTER_BOUND ( 'NONE', #6208, .T. ) ;
#6632=VECTOR ( 'NONE', #16377, 1000.000000000000000 ) ;
#6634=CARTESIAN_POINT ( 'NONE',  ( 77.31114765718494652, -12.23146955673620795, 112.0427633081292385 ) ) ;
#6635=EDGE_CURVE ( 'NONE', #1924, #19563, #5455, .T. ) ;
#6636=ORIENTED_EDGE ( 'NONE', *, *, #9012, .T. ) ;
#6640=VECTOR ( 'NONE', #20166, 1000.000000000000000 ) ;
#6641=LINE ( 'NONE', #290, #12307 ) ;
#6642=CYLINDRICAL_SURFACE ( 'NONE', #3285, 60.74260934110282051 ) ;
#6643=DIRECTION ( 'NONE',  ( 0.000000000000000000, 0.000000000000000000, 1.000000000000000000 ) ) ;
#6644=ORIENTED_EDGE ( 'NONE', *, *, #4772, .F. ) ;
#6645=DIRECTION ( 'NONE',  ( 0.1390141521205912056, -0.9902903945359629034, 0.000000000000000000 ) ) ;
#6646=ORIENTED_EDGE ( 'NONE', *, *, #11299, .T. ) ;
#6648=AXIS2_PLACEMENT_3D ( 'NONE', #13668, #1403, #13873 ) ;
#6650=EDGE_CURVE ( 'NONE', #16844, #18587, #9038, .T. ) ;
#6652=VERTEX_POINT ( 'NONE', #6210 ) ;
#6655=DIRECTION ( 'NONE',  ( 1.000000000000000000, 0.000000000000000000, -0.000000000000000000 ) ) ;
#6656=VECTOR ( 'NONE', #19449, 1000.000000000000227 ) ;
#6657=ORIENTED_EDGE ( 'NONE', *, *, #3104, .T. ) ;
#6658=VECTOR ( 'NONE', #11378, 999.9999999999998863 ) ;
#6661=LINE ( 'NONE', #12295, #11145 ) ;
#6663=DIRECTION ( 'NONE',  ( -0.000000000000000000, -0.000000000000000000, 1.000000000000000000 ) ) ;
#6665=CARTESIAN_POINT ( 'NONE',  ( 37.78198917157320125, -47.56244194535178593, 283.5832628385307999 ) ) ;
#6666=DIRECTION ( 'NONE',  ( -0.000000000000000000, -0.000000000000000000, 1.000000000000000000 ) ) ;
#6667=VERTEX_POINT ( 'NONE', #13961 ) ;
#6668=PLANE ( 'NONE',  #9567 ) ;
#6670=DIRECTION ( 'NONE',  ( -0.03505990758545545621, -0.9993852124581888985, 0.000000000000000000 ) ) ;
#6673=DIRECTION ( 'NONE',  ( -0.1736481776669241417, -0.9848077530122091305, 0.000000000000000000 ) ) ;
#6675=EDGE_CURVE ( 'NONE', #5793, #13282, #7419, .T. ) ;
#6677=ADVANCED_FACE ( 'NONE', ( #13656 ), #1596, .F. ) ;
#6680=PRODUCT_CONTEXT ( 'NONE', #17190, 'mechanical' ) ;
#6681=VECTOR ( 'NONE', #17116, 999.9999999999998863 ) ;
#6684=DIRECTION ( 'NONE',  ( 0.000000000000000000, 0.000000000000000000, 1.000000000000000000 ) ) ;
#6687=DIRECTION ( 'NONE',  ( -0.9993852124581887875, 0.03505990758545545621, 0.000000000000000000 ) ) ;
#6690=PLANE ( 'NONE',  #1098 ) ;
#6691=DIRECTION ( 'NONE',  ( -0.6155349844899689060, 0.7881095627315620744, 0.000000000000000000 ) ) ;
#6692=CIRCLE ( 'NONE', #20065, 62.91752772691707207 ) ;
#6693=CARTESIAN_POINT ( 'NONE',  ( 0.000000000000000000, 0.000000000000000000, 293.5832628385307999 ) ) ;
#6696=VERTEX_POINT ( 'NONE', #7825 ) ;
#6698=AXIS2_PLACEMENT_3D ( 'NONE', #2222, #17973, #6724 ) ;
#6699=ORIENTED_EDGE ( 'NONE', *, *, #492, .T. ) ;
#6701=VERTEX_POINT ( 'NONE', #18270 ) ;
#6702=VECTOR ( 'NONE', #15845, 1000.000000000000114 ) ;
#6704=LINE ( 'NONE', #8531, #7650 ) ;
#6705=CARTESIAN_POINT ( 'NONE',  ( -28.63313560863435825, 51.23821591265124198, 132.4711112102474146 ) ) ;
#6707=CARTESIAN_POINT ( 'NONE',  ( 0.000000000000000000, 0.000000000000000000, 293.5832628385307999 ) ) ;
#6708=ORIENTED_EDGE ( 'NONE', *, *, #6244, .T. ) ;
#6712=CARTESIAN_POINT ( 'NONE',  ( -41.06890862491506766, -47.66508197439458172, 132.4711112102474146 ) ) ;
#6713=LINE ( 'NONE', #6812, #4836 ) ;
#6718=ORIENTED_EDGE ( 'NONE', *, *, #2523, .T. ) ;
#6722=ORIENTED_EDGE ( 'NONE', *, *, #7504, .T. ) ;
#6723=DIRECTION ( 'NONE',  ( -0.6692498792541753394, -0.7430374143461900838, 0.000000000000000000 ) ) ;
#6724=DIRECTION ( 'NONE',  ( 1.000000000000000000, 3.491481338843133355E-15, 0.000000000000000000 ) ) ;
#6730=ORIENTED_EDGE ( 'NONE', *, *, #12968, .T. ) ;
#6732=DIRECTION ( 'NONE',  ( -0.000000000000000000, -0.000000000000000000, 1.000000000000000000 ) ) ;
#6733=FACE_OUTER_BOUND ( 'NONE', #17083, .T. ) ;
#6736=ADVANCED_FACE ( 'NONE', ( #18890 ), #15712, .F. ) ;
#6738=DIRECTION ( 'NONE',  ( -0.000000000000000000, -0.000000000000000000, 1.000000000000000000 ) ) ;
#6739=DIRECTION ( 'NONE',  ( -0.000000000000000000, -0.000000000000000000, 1.000000000000000000 ) ) ;
#6743=CYLINDRICAL_SURFACE ( 'NONE', #5023, 79.75827554147308263 ) ;
#6745=ORIENTED_EDGE ( 'NONE', *, *, #7717, .T. ) ;
#6746=EDGE_CURVE ( 'NONE', #6652, #959, #3432, .T. ) ;
#6749=VECTOR ( 'NONE', #17043, 1000.000000000000000 ) ;
#6751=AXIS2_PLACEMENT_3D ( 'NONE', #2998, #17112, #3098 ) ;
#6752=DIRECTION ( 'NONE',  ( 1.000000000000000000, 0.000000000000000000, 0.000000000000000000 ) ) ;
#6755=CARTESIAN_POINT ( 'NONE',  ( -61.70726652483826058, -12.28122767885825262, 248.9926560891072143 ) ) ;
#6756=EDGE_CURVE ( 'NONE', #13973, #6205, #6609, .T. ) ;
#6757=CARTESIAN_POINT ( 'NONE',  ( -57.61627707419551570, -19.23614321207253042, 283.5832628385307999 ) ) ;
#6759=DIRECTION ( 'NONE',  ( -0.9848077530122073542, -0.1736481776669340227, -0.000000000000000000 ) ) ;
#6762=EDGE_LOOP ( 'NONE', ( #5044, #5959, #1101, #3246 ) ) ;
#6763=CYLINDRICAL_SURFACE ( 'NONE', #7596, 60.74260934110282051 ) ;
#6764=DIRECTION ( 'NONE',  ( 1.000000000000000000, 0.000000000000000000, 0.000000000000000000 ) ) ;
#6768=ORIENTED_EDGE ( 'NONE', *, *, #10223, .F. ) ;
#6772=VERTEX_POINT ( 'NONE', #6514 ) ;
#6773=EDGE_LOOP ( 'NONE', ( #19048, #16599, #327, #16030 ) ) ;
#6774=AXIS2_PLACEMENT_3D ( 'NONE', #1652, #8080, #14227 ) ;
#6775=VERTEX_POINT ( 'NONE', #2104 ) ;
#6776=EDGE_CURVE ( 'NONE', #5779, #9877, #158, .T. ) ;
#6780=CARTESIAN_POINT ( 'NONE',  ( -73.82206860051547892, -25.99419088092166774, 111.4180192758973931 ) ) ;
#6781=VERTEX_POINT ( 'NONE', #12628 ) ;
#6783=DIRECTION ( 'NONE',  ( 0.000000000000000000, 0.000000000000000000, 1.000000000000000000 ) ) ;
#6785=ORIENTED_EDGE ( 'NONE', *, *, #17449, .T. ) ;
#6786=EDGE_CURVE ( 'NONE', #2414, #4265, #1373, .T. ) ;
#6787=EDGE_CURVE ( 'NONE', #19395, #5114, #14276, .T. ) ;
#6788=EDGE_CURVE ( 'NONE', #9930, #9275, #12733, .T. ) ;
#6790=DIRECTION ( 'NONE',  ( -0.000000000000000000, -0.000000000000000000, 1.000000000000000000 ) ) ;
#6791=CIRCLE ( 'NONE', #17240, 62.91752772691707207 ) ;
#6794=FACE_OUTER_BOUND ( 'NONE', #12998, .T. ) ;
#6796=ORIENTED_EDGE ( 'NONE', *, *, #750, .F. ) ;
#6800=ORIENTED_EDGE ( 'NONE', *, *, #61, .F. ) ;
#6801=CIRCLE ( 'NONE', #9406, 60.74260934110282051 ) ;
#6803=LINE ( 'NONE', #8625, #14821 ) ;
#6807=PLANE ( 'NONE',  #2291 ) ;
#6808=DIRECTION ( 'NONE',  ( -0.1736481776669241417, -0.9848077530122091305, -0.000000000000000000 ) ) ;
#6810=CARTESIAN_POINT ( 'NONE',  ( -60.68567895461851691, 2.629250726500500956, 283.5832628385307999 ) ) ;
#6812=CARTESIAN_POINT ( 'NONE',  ( 26.55444175051045974, 16.92388544840595799, 248.9926560891072143 ) ) ;
#6813=AXIS2_PLACEMENT_3D ( 'NONE', #19087, #5074, #18989 ) ;
#6814=EDGE_CURVE ( 'NONE', #399, #17740, #8130, .T. ) ;
#6815=ORIENTED_EDGE ( 'NONE', *, *, #18096, .F. ) ;
#6819=VERTEX_POINT ( 'NONE', #355 ) ;
#6821=ORIENTED_EDGE ( 'NONE', *, *, #20022, .F. ) ;
#6822=VECTOR ( 'NONE', #19380, 1000.000000000000227 ) ;
#6823=CIRCLE ( 'NONE', #16952, 62.91752772691707207 ) ;
#6824=CARTESIAN_POINT ( 'NONE',  ( 59.42266395395792955, -50.93469132750283279, 248.9926560891072143 ) ) ;
#6826=DIRECTION ( 'NONE',  ( -0.8660254037844328234, -0.5000000000000101030, 0.000000000000000000 ) ) ;
#6827=CARTESIAN_POINT ( 'NONE',  ( 38.35506425062457225, 44.43084819159290788, 132.4711112102474146 ) ) ;
#6830=DIRECTION ( 'NONE',  ( 0.9848077530122086864, -0.1736481776669273613, -0.000000000000000000 ) ) ;
#6831=ORIENTED_EDGE ( 'NONE', *, *, #19362, .F. ) ;
#6838=AXIS2_PLACEMENT_3D ( 'NONE', #20234, #19022, #7952 ) ;
#6839=VECTOR ( 'NONE', #6830, 999.9999999999998863 ) ;
#6840=EDGE_LOOP ( 'NONE', ( #18224, #3984, #1245, #17665 ) ) ;
#6844=CARTESIAN_POINT ( 'NONE',  ( 54.89456854707540856, 30.74413178637211885, 132.4711112102474146 ) ) ;
#6845=ORIENTED_EDGE ( 'NONE', *, *, #10383, .T. ) ;
#6846=CARTESIAN_POINT ( 'NONE',  ( 20.21777810286676313, 59.58067424803633116, 132.4711112102474146 ) ) ;
#6848=SURFACE_SIDE_STYLE ('',( #15861 ) ) ;
#6849=DIRECTION ( 'NONE',  ( 1.000000000000000000, 0.000000000000000000, 0.000000000000000000 ) ) ;
#6854=EDGE_CURVE ( 'NONE', #18461, #18497, #14474, .T. ) ;
#6858=VERTEX_POINT ( 'NONE', #3635 ) ;
#6859=DIRECTION ( 'NONE',  ( 1.047444401652940164E-14, -1.000000000000000000, 0.000000000000000000 ) ) ;
#6861=CARTESIAN_POINT ( 'NONE',  ( -62.09913334491130144, -10.11498556985140596, 248.9926560891072143 ) ) ;
#6862=DIRECTION ( 'NONE',  ( -0.1736481776669273336, -0.9848077530122085754, 0.000000000000000000 ) ) ;
#6864=PLANE ( 'NONE',  #12684 ) ;
#6866=ORIENTED_EDGE ( 'NONE', *, *, #7749, .F. ) ;
#6867=ORIENTED_EDGE ( 'NONE', *, *, #17624, .T. ) ;
#6868=ORIENTED_EDGE ( 'NONE', *, *, #13101, .F. ) ;
#6871=EDGE_CURVE ( 'NONE', #13282, #241, #2498, .T. ) ;
#6873=ORIENTED_EDGE ( 'NONE', *, *, #8272, .T. ) ;
#6874=EDGE_CURVE ( 'NONE', #4648, #9930, #19388, .T. ) ;
#6875=DIRECTION ( 'NONE',  ( 0.000000000000000000, 0.000000000000000000, 1.000000000000000000 ) ) ;
#6876=DIRECTION ( 'NONE',  ( 0.000000000000000000, 0.000000000000000000, 1.000000000000000000 ) ) ;
#6879=LINE ( 'NONE', #636, #15154 ) ;
#6881=AXIS2_PLACEMENT_3D ( 'NONE', #13378, #5621, #617 ) ;
#6883=CIRCLE ( 'NONE', #13711, 62.91752772691707207 ) ;
#6884=EDGE_CURVE ( 'NONE', #4813, #19147, #8538, .T. ) ;
#6887=DIRECTION ( 'NONE',  ( 0.4999999999999888978, 0.8660254037844449249, 0.000000000000000000 ) ) ;
#6888=CARTESIAN_POINT ( 'NONE',  ( -39.80940113485987553, 48.72193424476490975, 248.9926560891072143 ) ) ;
#6889=CARTESIAN_POINT ( 'NONE',  ( -54.89456854707562172, -30.74413178637172450, 293.5832628385307999 ) ) ;
#6892=CIRCLE ( 'NONE', #3305, 62.91752772691707207 ) ;
#6894=ADVANCED_FACE ( 'NONE', ( #13320 ), #13422, .F. ) ;
#6895=EDGE_CURVE ( 'NONE', #16743, #11013, #10356, .T. ) ;
#6896=ORIENTED_EDGE ( 'NONE', *, *, #18633, .F. ) ;
#6904=FACE_OUTER_BOUND ( 'NONE', #10463, .T. ) ;
#6905=VERTEX_POINT ( 'NONE', #2603 ) ;
#6908=AXIS2_PLACEMENT_3D ( 'NONE', #8411, #544, #16493 ) ;
#6914=FACE_OUTER_BOUND ( 'NONE', #4816, .T. ) ;
#6915=ORIENTED_EDGE ( 'NONE', *, *, #6650, .F. ) ;
#6916=ORIENTED_EDGE ( 'NONE', *, *, #15464, .T. ) ;
#6918=EDGE_CURVE ( 'NONE', #2266, #12685, #17959, .T. ) ;
#6919=EDGE_CURVE ( 'NONE', #6819, #1, #16220, .T. ) ;
#6921=ORIENTED_EDGE ( 'NONE', *, *, #9023, .T. ) ;
#6923=CARTESIAN_POINT ( 'NONE',  ( 56.12853591711344592, -23.22718332831461652, 293.5832628385307999 ) ) ;
#6925=CARTESIAN_POINT ( 'NONE',  ( 0.000000000000000000, 0.000000000000000000, 283.5832628385307999 ) ) ;
#6926=VERTEX_POINT ( 'NONE', #4230 ) ;
#6927=CARTESIAN_POINT ( 'NONE',  ( 51.24245927909996112, -32.62092819947974220, 293.5832628385307999 ) ) ;
#6928=CARTESIAN_POINT ( 'NONE',  ( -62.09913334491130854, -10.11498556985139352, 132.4711112102474146 ) ) ;
#6932=FACE_OUTER_BOUND ( 'NONE', #14977, .T. ) ;
#6933=CARTESIAN_POINT ( 'NONE',  ( 74.01264520835154315, -25.47058595421579241, 248.9926560891072143 ) ) ;
#6940=ORIENTED_EDGE ( 'NONE', *, *, #16160, .F. ) ;
#6941=ORIENTED_EDGE ( 'NONE', *, *, #12870, .F. ) ;
#6946=DIRECTION ( 'NONE',  ( 0.9848077530122103518, -0.1736481776669172583, 0.000000000000000000 ) ) ;
#6947=CYLINDRICAL_SURFACE ( 'NONE', #15187, 62.91752772691707207 ) ;
#6949=DIRECTION ( 'NONE',  ( -0.000000000000000000, -0.000000000000000000, 1.000000000000000000 ) ) ;
#6951=VECTOR ( 'NONE', #9140, 1000.000000000000000 ) ;
#6952=CARTESIAN_POINT ( 'NONE',  ( -73.82206860051547892, -25.99419088092166774, 111.4180192758973931 ) ) ;
#6953=CARTESIAN_POINT ( 'NONE',  ( 79.75827554147308263, 0.000000000000000000, 269.6944534026102360 ) ) ;
#6956=LINE ( 'NONE', #11558, #17882 ) ;
#6957=VECTOR ( 'NONE', #15246, 1000.000000000000000 ) ;
#6960=VERTEX_POINT ( 'NONE', #17541 ) ;
#6962=LINE ( 'NONE', #5433, #444 ) ;
#6963=ORIENTED_EDGE ( 'NONE', *, *, #10525, .F. ) ;
#6964=EDGE_LOOP ( 'NONE', ( #15380, #15492, #4549, #1143 ) ) ;
#6967=AXIS2_PLACEMENT_3D ( 'NONE', #10180, #11426, #677 ) ;
#6968=EDGE_CURVE ( 'NONE', #11476, #675, #9449, .T. ) ;
#6969=CARTESIAN_POINT ( 'NONE',  ( 2.240720816136066773, -5.281164089014814600, 293.5832628385307999 ) ) ;
#6975=VERTEX_POINT ( 'NONE', #8008 ) ;
#6976=CARTESIAN_POINT ( 'NONE',  ( 60.22232964560483737, 7.948937137877944537, 293.5832628385307999 ) ) ;
#6978=LINE ( 'NONE', #16587, #11867 ) ;
#6980=CARTESIAN_POINT ( 'NONE',  ( -62.91752772691707207, 7.705174894103383492E-15, 83.57543755549745867 ) ) ;
#6983=CARTESIAN_POINT ( 'NONE',  ( -10.99904278960814352, 0.5388563210140320248, 248.9926560891072143 ) ) ;
#6988=FACE_OUTER_BOUND ( 'NONE', #7208, .T. ) ;
#6994=ORIENTED_EDGE ( 'NONE', *, *, #12545, .F. ) ;
#6995=LINE ( 'NONE', #3629, #12198 ) ;
#6999=CARTESIAN_POINT ( 'NONE',  ( -27.53920554013687649, -73.25972925305620720, 248.9926560891072143 ) ) ;
#7000=CARTESIAN_POINT ( 'NONE',  ( 0.000000000000000000, 0.000000000000000000, 293.5832628385307999 ) ) ;
#7001=VERTEX_POINT ( 'NONE', #10972 ) ;
#7008=CARTESIAN_POINT ( 'NONE',  ( 0.000000000000000000, 0.000000000000000000, 283.5832628385307999 ) ) ;
#7009=DIRECTION ( 'NONE',  ( -0.3088643371590125697, 0.9511061040868803440, 0.000000000000000000 ) ) ;
#7011=EDGE_CURVE ( 'NONE', #13585, #12690, #2041, .T. ) ;
#7012=EDGE_LOOP ( 'NONE', ( #425, #819, #1448, #9370 ) ) ;
#7016=ORIENTED_EDGE ( 'NONE', *, *, #12245, .T. ) ;
#7017=DIRECTION ( 'NONE',  ( -0.1736481776669172861, -0.9848077530122104628, 0.000000000000000000 ) ) ;
#7022=FACE_OUTER_BOUND ( 'NONE', #15807, .T. ) ;
#7023=ORIENTED_EDGE ( 'NONE', *, *, #16603, .T. ) ;
#7024=VECTOR ( 'NONE', #18632, 1000.000000000000000 ) ;
#7025=CARTESIAN_POINT ( 'NONE',  ( -5.485913980968086356, 1.678175111358128024, 293.5832628385307999 ) ) ;
#7026=DIRECTION ( 'NONE',  ( -0.000000000000000000, -0.000000000000000000, 1.000000000000000000 ) ) ;
#7027=ORIENTED_EDGE ( 'NONE', *, *, #11875, .F. ) ;
#7028=CARTESIAN_POINT ( 'NONE',  ( -37.09555676056967144, 45.48770046196298011, 110.7293897666001214 ) ) ;
#7029=CARTESIAN_POINT ( 'NONE',  ( 41.02350267428969488, 44.79940644582669051, 293.5832628385307999 ) ) ;
#7030=DIRECTION ( 'NONE',  ( -0.000000000000000000, -0.000000000000000000, 1.000000000000000000 ) ) ;
#7034=CARTESIAN_POINT ( 'NONE',  ( -45.48770046196285932, -37.09555676056982065, 132.4711112102474146 ) ) ;
#7035=EDGE_CURVE ( 'NONE', #7429, #10010, #18766, .T. ) ;
#7037=DIRECTION ( 'NONE',  ( -0.3420201433256663259, -0.9396926207859093161, 0.000000000000000000 ) ) ;
#7039=EDGE_CURVE ( 'NONE', #12098, #5832, #7251, .T. ) ;
#7041=ADVANCED_FACE ( 'NONE', ( #15589 ), #3315, .F. ) ;
#7042=ORIENTED_EDGE ( 'NONE', *, *, #11663, .F. ) ;
#7045=CARTESIAN_POINT ( 'NONE',  ( -22.30005961346265408, -56.50329132715937419, 293.5832628385307999 ) ) ;
#7046=ORIENTED_EDGE ( 'NONE', *, *, #12086, .T. ) ;
#7048=CARTESIAN_POINT ( 'NONE',  ( 54.07248341783252954, -32.16802499836759210, 248.9926560891072143 ) ) ;
#7052=ORIENTED_EDGE ( 'NONE', *, *, #9797, .T. ) ;
#7053=CARTESIAN_POINT ( 'NONE',  ( -44.79787735033389851, 41.02212542604627998, 283.5832628385307999 ) ) ;
#7055=VECTOR ( 'NONE', #6946, 1000.000000000000000 ) ;
#7056=CARTESIAN_POINT ( 'NONE',  ( -9.401191644522826962, 61.25984398917663754, 248.9926560891072143 ) ) ;
#7057=CARTESIAN_POINT ( 'NONE',  ( 3.911853314815645799, -4.196299268919061021, 293.5832628385307999 ) ) ;
#7062=FACE_OUTER_BOUND ( 'NONE', #12799, .T. ) ;
#7064=ORIENTED_EDGE ( 'NONE', *, *, #12748, .T. ) ;
#7066=DIRECTION ( 'NONE',  ( -0.000000000000000000, -0.000000000000000000, 1.000000000000000000 ) ) ;
#7067=ORIENTED_EDGE ( 'NONE', *, *, #7734, .T. ) ;
#7070=ORIENTED_EDGE ( 'NONE', *, *, #7772, .F. ) ;
#7071=LINE ( 'NONE', #5049, #10422 ) ;
#7079=FACE_OUTER_BOUND ( 'NONE', #3599, .T. ) ;
#7081=DIRECTION ( 'NONE',  ( 0.9396926207859046531, 0.3420201433256790380, 0.000000000000000000 ) ) ;
#7084=DIRECTION ( 'NONE',  ( -0.6155349844899689060, 0.7881095627315620744, 0.000000000000000000 ) ) ;
#7087=AXIS2_PLACEMENT_3D ( 'NONE', #6464, #17412, #5135 ) ;
#7090=EDGE_LOOP ( 'NONE', ( #9408, #6333, #13237 ) ) ;
#7092=VERTEX_POINT ( 'NONE', #14845 ) ;
#7094=CARTESIAN_POINT ( 'NONE',  ( 22.29928840491074382, 56.50138340076680521, 293.5832628385307999 ) ) ;
#7095=ORIENTED_EDGE ( 'NONE', *, *, #8274, .T. ) ;
#7099=LINE ( 'NONE', #18045, #19878 ) ;
#7100=CARTESIAN_POINT ( 'NONE',  ( 77.21438937758502163, 12.78021302872874010, 112.0427633081291816 ) ) ;
#7101=DIRECTION ( 'NONE',  ( -0.7660444431189707970, -0.6427876096865481337, 0.000000000000000000 ) ) ;
#7103=CARTESIAN_POINT ( 'NONE',  ( 59.30917539369505675, -13.12769224524051559, 283.5832628385307999 ) ) ;
#7104=FACE_OUTER_BOUND ( 'NONE', #19344, .T. ) ;
#7105=DIRECTION ( 'NONE',  ( 1.000000000000000000, 0.000000000000000000, 0.000000000000000000 ) ) ;
#7110=AXIS2_PLACEMENT_3D ( 'NONE', #7336, #13778, #9072 ) ;
#7114=EDGE_LOOP ( 'NONE', ( #11369, #7169, #5626, #474 ) ) ;
#7116=ADVANCED_FACE ( 'NONE', ( #3999 ), #10239, .T. ) ;
#7120=CARTESIAN_POINT ( 'NONE',  ( 50.93469132750264095, 59.42266395395811429, 248.9926560891072143 ) ) ;
#7122=VERTEX_POINT ( 'NONE', #11480 ) ;
#7126=ORIENTED_EDGE ( 'NONE', *, *, #3663, .T. ) ;
#7127=CARTESIAN_POINT ( 'NONE',  ( 0.000000000000000000, 0.000000000000000000, 283.5832628385307999 ) ) ;
#7128=VECTOR ( 'NONE', #18278, 999.9999999999998863 ) ;
#7131=DIRECTION ( 'NONE',  ( -0.4999999999999919509, -0.8660254037844432595, 0.000000000000000000 ) ) ;
#7134=CARTESIAN_POINT ( 'NONE',  ( -73.06915264522021403, -28.06281046684251024, 248.9926560891072143 ) ) ;
#7139=VECTOR ( 'NONE', #10420, 1000.000000000000000 ) ;
#7140=VECTOR ( 'NONE', #2348, 1000.000000000000000 ) ;
#7143=AXIS2_PLACEMENT_3D ( 'NONE', #13279, #19540, #8790 ) ;
#7144=ORIENTED_EDGE ( 'NONE', *, *, #18919, .T. ) ;
#7146=EDGE_CURVE ( 'NONE', #20213, #1969, #16302, .T. ) ;
#7147=EDGE_CURVE ( 'NONE', #12841, #7735, #8413, .T. ) ;
#7149=CARTESIAN_POINT ( 'NONE',  ( 76.92888220842486646, -14.39940464655733976, 132.4711112102474146 ) ) ;
#7152=DIRECTION ( 'NONE',  ( 1.000000000000000000, 0.000000000000000000, 0.000000000000000000 ) ) ;
#7153=ORIENTED_EDGE ( 'NONE', *, *, #9225, .F. ) ;
#7155=DIRECTION ( 'NONE',  ( 1.000000000000000000, 0.000000000000000000, 0.000000000000000000 ) ) ;
#7156=AXIS2_PLACEMENT_3D ( 'NONE', #1417, #18607, #4588 ) ;
#7158=DIRECTION ( 'NONE',  ( -0.000000000000000000, -0.000000000000000000, 1.000000000000000000 ) ) ;
#7159=DIRECTION ( 'NONE',  ( -0.3088643371590125697, 0.9511061040868803440, 0.000000000000000000 ) ) ;
#7160=VECTOR ( 'NONE', #12012, 1000.000000000000000 ) ;
#7161=ORIENTED_EDGE ( 'NONE', *, *, #13211, .F. ) ;
#7162=EDGE_CURVE ( 'NONE', #4103, #18829, #16397, .T. ) ;
#7163=CARTESIAN_POINT ( 'NONE',  ( 5.693982670708940041, -0.7000608949449556029, 283.5832628385307999 ) ) ;
#7164=FACE_OUTER_BOUND ( 'NONE', #11817, .T. ) ;
#7166=ORIENTED_EDGE ( 'NONE', *, *, #11276, .F. ) ;
#7168=CARTESIAN_POINT ( 'NONE',  ( -77.31114765718486126, 12.23146955673674796, 132.4711112102474146 ) ) ;
#7169=ORIENTED_EDGE ( 'NONE', *, *, #5601, .T. ) ;
#7174=VECTOR ( 'NONE', #14349, 1000.000000000000227 ) ;
#7175=CIRCLE ( 'NONE', #15679, 79.75827554147308263 ) ;
#7178=ORIENTED_EDGE ( 'NONE', *, *, #15408, .F. ) ;
#7180=LINE ( 'NONE', #18213, #7333 ) ;
#7182=FACE_OUTER_BOUND ( 'NONE', #1988, .T. ) ;
#7187=AXIS2_PLACEMENT_3D ( 'NONE', #7100, #11984, #11596 ) ;
#7189=DIRECTION ( 'NONE',  ( 1.000000000000000000, 0.000000000000000000, 0.000000000000000000 ) ) ;
#7193=ORIENTED_EDGE ( 'NONE', *, *, #19983, .T. ) ;
#7195=CARTESIAN_POINT ( 'NONE',  ( -60.47951622432784546, -49.67518383744813804, 110.7293897666001214 ) ) ;
#7196=EDGE_LOOP ( 'NONE', ( #8090, #17108, #661, #6868 ) ) ;
#7198=PLANE ( 'NONE',  #18019 ) ;
#7200=DIRECTION ( 'NONE',  ( 0.3420201433256694901, -0.9396926207859082059, 0.000000000000000000 ) ) ;
#7201=ORIENTED_EDGE ( 'NONE', *, *, #6871, .F. ) ;
#7202=DIRECTION ( 'NONE',  ( -0.2080686897406911207, -0.9781142164131917394, 0.000000000000000000 ) ) ;
#7206=DIRECTION ( 'NONE',  ( -0.000000000000000000, -0.000000000000000000, 1.000000000000000000 ) ) ;
#7208=EDGE_LOOP ( 'NONE', ( #9848, #11862, #3715, #6867 ) ) ;
#7210=ORIENTED_EDGE ( 'NONE', *, *, #14652, .F. ) ;
#7211=ORIENTED_EDGE ( 'NONE', *, *, #999, .F. ) ;
#7212=ORIENTED_EDGE ( 'NONE', *, *, #5904, .T. ) ;
#7213=ORIENTED_EDGE ( 'NONE', *, *, #14984, .F. ) ;
#7214=EDGE_CURVE ( 'NONE', #9982, #13976, #17935, .T. ) ;
#7215=VECTOR ( 'NONE', #2828, 1000.000000000000000 ) ;
#7218=VERTEX_POINT ( 'NONE', #5544 ) ;
#7223=DIRECTION ( 'NONE',  ( 0.000000000000000000, 0.000000000000000000, 1.000000000000000000 ) ) ;
#7226=LINE ( 'NONE', #10480, #1004 ) ;
#7230=DIRECTION ( 'NONE',  ( 0.6427876096865379196, 0.7660444431189792347, 0.000000000000000000 ) ) ;
#7235=ORIENTED_EDGE ( 'NONE', *, *, #6383, .T. ) ;
#7237=CARTESIAN_POINT ( 'NONE',  ( 0.000000000000000000, 0.000000000000000000, 132.4711112102474146 ) ) ;
#7238=VERTEX_POINT ( 'NONE', #8707 ) ;
#7239=ORIENTED_EDGE ( 'NONE', *, *, #18828, .T. ) ;
#7240=EDGE_CURVE ( 'NONE', #10983, #14953, #19363, .T. ) ;
#7244=LINE ( 'NONE', #13568, #13877 ) ;
#7251=CIRCLE ( 'NONE', #3671, 62.91752772691707207 ) ;
#7252=PLANE ( 'NONE',  #13950 ) ;
#7255=DIRECTION ( 'NONE',  ( -0.000000000000000000, -0.000000000000000000, 1.000000000000000000 ) ) ;
#7256=EDGE_LOOP ( 'NONE', ( #17402, #8857, #3120, #13427 ) ) ;
#7257=ADVANCED_FACE ( 'NONE', ( #1128 ), #5745, .F. ) ;
#7258=DIRECTION ( 'NONE',  ( -0.7430374143461878633, 0.6692498792541777819, 0.000000000000000000 ) ) ;
#7259=DIRECTION ( 'NONE',  ( -0.000000000000000000, -0.000000000000000000, 1.000000000000000000 ) ) ;
#7261=ORIENTED_EDGE ( 'NONE', *, *, #4068, .T. ) ;
#7265=DIRECTION ( 'NONE',  ( 0.000000000000000000, 0.000000000000000000, 1.000000000000000000 ) ) ;
#7266=VECTOR ( 'NONE', #2812, 1000.000000000000000 ) ;
#7268=LINE ( 'NONE', #8896, #4435 ) ;
#7269=DIRECTION ( 'NONE',  ( 0.000000000000000000, 0.000000000000000000, -1.000000000000000000 ) ) ;
#7271=PLANE ( 'NONE',  #12094 ) ;
#7272=DIRECTION ( 'NONE',  ( -0.5000000000000009992, 0.8660254037844380415, 0.000000000000000000 ) ) ;
#7273=DIRECTION ( 'NONE',  ( 1.000000000000000000, 0.000000000000000000, 0.000000000000000000 ) ) ;
#7274=EDGE_CURVE ( 'NONE', #8089, #4188, #3990, .T. ) ;
#7277=LINE ( 'NONE', #18125, #6312 ) ;
#7279=ORIENTED_EDGE ( 'NONE', *, *, #13842, .T. ) ;
#7280=CARTESIAN_POINT ( 'NONE',  ( 7.948937137877743808, -60.22232964560488000, 293.5832628385307999 ) ) ;
#7282=AXIS2_PLACEMENT_3D ( 'NONE', #17718, #7259, #13480 ) ;
#7283=ORIENTED_EDGE ( 'NONE', *, *, #15557, .F. ) ;
#7285=EDGE_LOOP ( 'NONE', ( #594, #10961, #7413 ) ) ;
#7286=EDGE_CURVE ( 'NONE', #6626, #2011, #13499, .T. ) ;
#7291=DIRECTION ( 'NONE',  ( 0.3420201433256662704, 0.9396926207859092051, 0.000000000000000000 ) ) ;
#7292=LINE ( 'NONE', #13727, #15965 ) ;
#7293=DIRECTION ( 'NONE',  ( -0.000000000000000000, -0.000000000000000000, 1.000000000000000000 ) ) ;
#7299=CARTESIAN_POINT ( 'NONE',  ( 0.000000000000000000, 0.000000000000000000, 293.5832628385307999 ) ) ;
#7300=CARTESIAN_POINT ( 'NONE',  ( 0.000000000000000000, 0.000000000000000000, 283.5832628385307999 ) ) ;
#7307=ORIENTED_EDGE ( 'NONE', *, *, #1870, .T. ) ;
#7309=CIRCLE ( 'NONE', #17457, 60.74260934110282051 ) ;
#7311=AXIS2_PLACEMENT_3D ( 'NONE', #481, #14788, #19309 ) ;
#7312=CARTESIAN_POINT ( 'NONE',  ( 10.52001906124917774, 3.255534882826434551, 248.9926560891072143 ) ) ;
#7315=CARTESIAN_POINT ( 'NONE',  ( -57.94128254008190027, -9.381844291199545438, 112.0427633081291816 ) ) ;
#7318=CARTESIAN_POINT ( 'NONE',  ( -20.21777810286715749, -59.58067424803620327, 293.5832628385307999 ) ) ;
#7320=DIRECTION ( 'NONE',  ( 1.000000000000000000, 0.000000000000000000, 0.000000000000000000 ) ) ;
#7323=DIRECTION ( 'NONE',  ( -0.6155349844899689060, 0.7881095627315620744, 0.000000000000000000 ) ) ;
#7327=AXIS2_PLACEMENT_3D ( 'NONE', #1359, #7586, #7490 ) ;
#7329=ORIENTED_EDGE ( 'NONE', *, *, #525, .F. ) ;
#7330=DIRECTION ( 'NONE',  ( 1.000000000000000000, 0.000000000000000000, 0.000000000000000000 ) ) ;
#7333=VECTOR ( 'NONE', #8897, 1000.000000000000000 ) ;
#7336=CARTESIAN_POINT ( 'NONE',  ( 0.000000000000000000, 0.000000000000000000, 293.5832628385307999 ) ) ;
#7340=DIRECTION ( 'NONE',  ( -0.5300553768524375320, -0.8479630283625697595, 0.000000000000000000 ) ) ;
#7343=DIRECTION ( 'NONE',  ( 1.000000000000000000, 0.000000000000000000, 0.000000000000000000 ) ) ;
#7344=CARTESIAN_POINT ( 'NONE',  ( 19.23677882349201695, -57.61823435390814296, 293.5832628385307999 ) ) ;
#7346=ORIENTED_EDGE ( 'NONE', *, *, #5226, .F. ) ;
#7349=VECTOR ( 'NONE', #14012, 1000.000000000000000 ) ;
#7356=EDGE_LOOP ( 'NONE', ( #7346, #12000, #10954, #4513 ) ) ;
#7358=EDGE_LOOP ( 'NONE', ( #4462, #14287, #6636, #17081 ) ) ;
#7359=AXIS2_PLACEMENT_3D ( 'NONE', #2734, #7529, #9168 ) ;
#7361=EDGE_CURVE ( 'NONE', #4545, #1924, #7568, .T. ) ;
#7362=CARTESIAN_POINT ( 'NONE',  ( -56.50138340076688337, 22.29928840491054487, 283.5832628385307999 ) ) ;
#7370=CYLINDRICAL_SURFACE ( 'NONE', #16249, 60.74260934110282051 ) ;
#7371=PLANE ( 'NONE',  #20215 ) ;
#7373=ORIENTED_EDGE ( 'NONE', *, *, #18850, .T. ) ;
#7374=ADVANCED_FACE ( 'NONE', ( #1444 ), #20159, .F. ) ;
#7375=DIRECTION ( 'NONE',  ( -0.9993852124581887875, 0.03505990758545896036, 0.000000000000000000 ) ) ;
#7376=CARTESIAN_POINT ( 'NONE',  ( 32.03743494504719536, 36.03492788066214558, 248.9926560891072143 ) ) ;
#7377=ORIENTED_EDGE ( 'NONE', *, *, #1855, .F. ) ;
#7378=VECTOR ( 'NONE', #11119, 999.9999999999998863 ) ;
#7379=VERTEX_POINT ( 'NONE', #15870 ) ;
#7381=CARTESIAN_POINT ( 'NONE',  ( 60.68567895461851691, -2.629250726500488078, 283.5832628385307999 ) ) ;
#7382=ORIENTED_EDGE ( 'NONE', *, *, #11875, .T. ) ;
#7386=EDGE_CURVE ( 'NONE', #13644, #8891, #5635, .T. ) ;
#7387=ADVANCED_FACE ( 'NONE', ( #1848 ), #6668, .F. ) ;
#7389=LINE ( 'NONE', #2691, #695 ) ;
#7391=CARTESIAN_POINT ( 'NONE',  ( 32.61983739937762294, 51.24071425735590424, 293.5832628385307999 ) ) ;
#7392=VERTEX_POINT ( 'NONE', #8079 ) ;
#7397=LINE ( 'NONE', #9032, #12975 ) ;
#7399=EDGE_CURVE ( 'NONE', #8543, #14775, #11, .T. ) ;
#7400=ORIENTED_EDGE ( 'NONE', *, *, #11357, .T. ) ;
#7402=VECTOR ( 'NONE', #10919, 1000.000000000000114 ) ;
#7403=VERTEX_POINT ( 'NONE', #109 ) ;
#7404=VECTOR ( 'NONE', #4949, 1000.000000000000000 ) ;
#7405=VERTEX_POINT ( 'NONE', #3388 ) ;
#7407=CIRCLE ( 'NONE', #18868, 62.91752772691707207 ) ;
#7408=ORIENTED_EDGE ( 'NONE', *, *, #14389, .T. ) ;
#7409=EDGE_CURVE ( 'NONE', #8342, #17256, #15668, .T. ) ;
#7412=FACE_OUTER_BOUND ( 'NONE', #4357, .T. ) ;
#7413=ORIENTED_EDGE ( 'NONE', *, *, #5601, .F. ) ;
#7414=DIRECTION ( 'NONE',  ( 1.000000000000000000, 0.000000000000000000, 0.000000000000000000 ) ) ;
#7415=FACE_OUTER_BOUND ( 'NONE', #16101, .T. ) ;
#7419=LINE ( 'NONE', #9159, #2353 ) ;
#7421=CARTESIAN_POINT ( 'NONE',  ( 37.78198917157319414, -47.56244194535178593, 293.5832628385307999 ) ) ;
#7426=LINE ( 'NONE', #18477, #20132 ) ;
#7427=VERTEX_POINT ( 'NONE', #3288 ) ;
#7429=VERTEX_POINT ( 'NONE', #17204 ) ;
#7430=VERTEX_POINT ( 'NONE', #5033 ) ;
#7431=CARTESIAN_POINT ( 'NONE',  ( 39.37628763770420193, 49.07263256785965666, 132.4711112102474146 ) ) ;
#7435=DIRECTION ( 'NONE',  ( 0.4999999999999950040, 0.8660254037844415942, 0.000000000000000000 ) ) ;
#7436=CARTESIAN_POINT ( 'NONE',  ( 0.000000000000000000, 0.000000000000000000, 293.5832628385307999 ) ) ;
#7439=LINE ( 'NONE', #1621, #16532 ) ;
#7441=ORIENTED_EDGE ( 'NONE', *, *, #11168, .T. ) ;
#7444=DIRECTION ( 'NONE',  ( -0.9848077530122097967, 0.1736481776669206722, 0.000000000000000000 ) ) ;
#7445=DIRECTION ( 'NONE',  ( 0.000000000000000000, 0.000000000000000000, -1.000000000000000000 ) ) ;
#7447=DIRECTION ( 'NONE',  ( -0.000000000000000000, -0.000000000000000000, 1.000000000000000000 ) ) ;
#7448=VECTOR ( 'NONE', #10162, 1000.000000000000114 ) ;
#7454=VERTEX_POINT ( 'NONE', #9317 ) ;
#7455=EDGE_LOOP ( 'NONE', ( #3013, #16994, #17891, #8761 ) ) ;
#7457=ORIENTED_EDGE ( 'NONE', *, *, #19302, .F. ) ;
#7459=LINE ( 'NONE', #13802, #12854 ) ;
#7463=PLANE ( 'NONE',  #161 ) ;
#7466=EDGE_CURVE ( 'NONE', #6324, #12822, #4990, .T. ) ;
#7471=DIRECTION ( 'NONE',  ( 0.9396926207859082059, 0.3420201433256694901, 0.000000000000000000 ) ) ;
#7474=ADVANCED_FACE ( 'NONE', ( #1547 ), #17411, .F. ) ;
#7475=PLANE ( 'NONE',  #18896 ) ;
#7476=DIRECTION ( 'NONE',  ( -0.000000000000000000, -0.000000000000000000, 1.000000000000000000 ) ) ;
#7479=VECTOR ( 'NONE', #10479, 999.9999999999998863 ) ;
#7480=CIRCLE ( 'NONE', #11405, 62.91752772691707207 ) ;
#7481=ADVANCED_FACE ( 'NONE', ( #11254 ), #9524, .F. ) ;
#7484=FACE_BOUND ( 'NONE', #5885, .T. ) ;
#7486=PLANE ( 'NONE',  #10870 ) ;
#7488=DIRECTION ( 'NONE',  ( -0.000000000000000000, -0.000000000000000000, 1.000000000000000000 ) ) ;
#7490=DIRECTION ( 'NONE',  ( 1.000000000000000000, 0.000000000000000000, -0.000000000000000000 ) ) ;
#7493=VECTOR ( 'NONE', #16681, 1000.000000000000000 ) ;
#7494=CIRCLE ( 'NONE', #16646, 62.91752772691707207 ) ;
#7496=CARTESIAN_POINT ( 'NONE',  ( 1.379293853801755176, 62.91752772691707207, 248.9926560891072143 ) ) ;
#7497=FACE_OUTER_BOUND ( 'NONE', #10882, .T. ) ;
#7499=FACE_OUTER_BOUND ( 'NONE', #13075, .T. ) ;
#7500=CARTESIAN_POINT ( 'NONE',  ( -40.27908801169994035, -45.46712722958821473, 283.5832628385307999 ) ) ;
#7502=ORIENTED_EDGE ( 'NONE', *, *, #4969, .T. ) ;
#7504=EDGE_CURVE ( 'NONE', #7430, #3408, #311, .T. ) ;
#7506=ORIENTED_EDGE ( 'NONE', *, *, #6398, .T. ) ;
#7510=LINE ( 'NONE', #966, #9600 ) ;
#7513=DIRECTION ( 'NONE',  ( -0.3420201433256694901, 0.9396926207859082059, 0.000000000000000000 ) ) ;
#7522=AXIS2_PLACEMENT_3D ( 'NONE', #4072, #10307, #8782 ) ;
#7524=EDGE_CURVE ( 'NONE', #934, #93, #14824, .T. ) ;
#7529=DIRECTION ( 'NONE',  ( -0.000000000000000000, -0.000000000000000000, 1.000000000000000000 ) ) ;
#7530=ORIENTED_EDGE ( 'NONE', *, *, #18776, .T. ) ;
#7531=EDGE_CURVE ( 'NONE', #7429, #16671, #9880, .T. ) ;
#7533=CYLINDRICAL_SURFACE ( 'NONE', #6648, 60.74260934110282051 ) ;
#7534=CIRCLE ( 'NONE', #15056, 62.91752772691707207 ) ;
#7544=ORIENTED_EDGE ( 'NONE', *, *, #5640, .T. ) ;
#7545=LINE ( 'NONE', #12246, #8702 ) ;
#7546=CARTESIAN_POINT ( 'NONE',  ( 0.000000000000000000, 0.000000000000000000, 293.5832628385307999 ) ) ;
#7549=CYLINDRICAL_SURFACE ( 'NONE', #18879, 60.74260934110282051 ) ;
#7550=DIRECTION ( 'NONE',  ( -0.8479630283625716469, 0.5300553768524345344, 0.000000000000000000 ) ) ;
#7555=FACE_OUTER_BOUND ( 'NONE', #7356, .T. ) ;
#7557=ORIENTED_EDGE ( 'NONE', *, *, #14156, .F. ) ;
#7559=PLANE ( 'NONE',  #1591 ) ;
#7568=LINE ( 'NONE', #13811, #20011 ) ;
#7574=LINE ( 'NONE', #7376, #6640 ) ;
#7579=VECTOR ( 'NONE', #5402, 1000.000000000000000 ) ;
#7581=ORIENTED_EDGE ( 'NONE', *, *, #7651, .F. ) ;
#7582=FACE_BOUND ( 'NONE', #8768, .T. ) ;
#7584=DIRECTION ( 'NONE',  ( -0.000000000000000000, -0.000000000000000000, 1.000000000000000000 ) ) ;
#7586=DIRECTION ( 'NONE',  ( 0.000000000000000000, 0.000000000000000000, 1.000000000000000000 ) ) ;
#7587=ADVANCED_FACE ( 'NONE', ( #5232 ), #11557, .F. ) ;
#7596=AXIS2_PLACEMENT_3D ( 'NONE', #12985, #175, #73 ) ;
#7597=CARTESIAN_POINT ( 'NONE',  ( -62.09913334491130854, -10.11498556985139352, 293.5832628385307999 ) ) ;
#7605=ORIENTED_EDGE ( 'NONE', *, *, #685, .T. ) ;
#7609=ADVANCED_FACE ( 'NONE', ( #8285 ), #11650, .F. ) ;
#7610=DIRECTION ( 'NONE',  ( 1.000000000000000000, 0.000000000000000000, -0.000000000000000000 ) ) ;
#7611=ORIENTED_EDGE ( 'NONE', *, *, #10229, .F. ) ;
#7615=DIRECTION ( 'NONE',  ( 0.4999999999999950040, 0.8660254037844415942, 0.000000000000000000 ) ) ;
#7618=CARTESIAN_POINT ( 'NONE',  ( 73.25972925305627825, -27.53920554013664912, 248.9926560891072143 ) ) ;
#7619=CARTESIAN_POINT ( 'NONE',  ( -57.55901709132179178, -11.54977938102067547, 112.0427633081291816 ) ) ;
#7621=CARTESIAN_POINT ( 'NONE',  ( 73.82206860051529418, 25.99419088092216867, 132.4711112102474146 ) ) ;
#7622=DIRECTION ( 'NONE',  ( -0.000000000000000000, -0.000000000000000000, 1.000000000000000000 ) ) ;
#7627=ORIENTED_EDGE ( 'NONE', *, *, #11853, .F. ) ;
#7629=LINE ( 'NONE', #10486, #2802 ) ;
#7631=VECTOR ( 'NONE', #6790, 1000.000000000000000 ) ;
#7634=AXIS2_PLACEMENT_3D ( 'NONE', #15834, #4995, #17478 ) ;
#7637=CARTESIAN_POINT ( 'NONE',  ( 18.28567271940513450, -57.92709869106715814, 293.5832628385307999 ) ) ;
#7641=ADVANCED_FACE ( 'NONE', ( #518 ), #6763, .F. ) ;
#7643=CARTESIAN_POINT ( 'NONE',  ( 0.000000000000000000, 0.000000000000000000, 283.5832628385307999 ) ) ;
#7644=CARTESIAN_POINT ( 'NONE',  ( 0.000000000000000000, 0.000000000000000000, 283.5832628385307999 ) ) ;
#7645=EDGE_LOOP ( 'NONE', ( #17326, #1692, #6274, #14295 ) ) ;
#7646=CARTESIAN_POINT ( 'NONE',  ( 5.485913980968119219, -1.678175111358107374, 293.5832628385307999 ) ) ;
#7647=CARTESIAN_POINT ( 'NONE',  ( -28.06584155524100765, 53.86996498385663301, 283.5832628385307999 ) ) ;
#7650=VECTOR ( 'NONE', #11594, 1000.000000000000000 ) ;
#7651=EDGE_CURVE ( 'NONE', #10388, #2887, #10539, .T. ) ;
#7657=LINE ( 'NONE', #1210, #10881 ) ;
#7658=ADVANCED_FACE ( 'NONE', ( #18808 ), #14192, .T. ) ;
#7659=VERTEX_POINT ( 'NONE', #6428 ) ;
#7660=EDGE_LOOP ( 'NONE', ( #5533, #19398, #3368, #6475 ) ) ;
#7662=CARTESIAN_POINT ( 'NONE',  ( -62.18629025319808790, 9.564549117045718418, 293.5832628385307999 ) ) ;
#7664=VERTEX_POINT ( 'NONE', #17169 ) ;
#7665=CARTESIAN_POINT ( 'NONE',  ( -22.29928840491073316, -56.50138340076681231, 283.5832628385307999 ) ) ;
#7667=ORIENTED_EDGE ( 'NONE', *, *, #13910, .T. ) ;
#7670=LINE ( 'NONE', #3379, #2178 ) ;
#7673=ORIENTED_EDGE ( 'NONE', *, *, #457, .T. ) ;
#7674=DIRECTION ( 'NONE',  ( -0.7430374143461878633, 0.6692498792541777819, 0.000000000000000000 ) ) ;
#7680=DIRECTION ( 'NONE',  ( -0.2080686897406943958, -0.9781142164131909622, 0.000000000000000000 ) ) ;
#7681=CARTESIAN_POINT ( 'NONE',  ( -62.18629025319808790, 9.564549117045714866, 248.9926560891072143 ) ) ;
#7685=ORIENTED_EDGE ( 'NONE', *, *, #13024, .F. ) ;
#7687=FACE_BOUND ( 'NONE', #11682, .T. ) ;
#7692=CARTESIAN_POINT ( 'NONE',  ( 62.90240729679780429, 1.379293853802413983, 248.9926560891072143 ) ) ;
#7695=ADVANCED_FACE ( 'NONE', ( #14086 ), #3252, .F. ) ;
#7699=DIRECTION ( 'NONE',  ( 0.000000000000000000, 0.000000000000000000, -1.000000000000000000 ) ) ;
#7700=CIRCLE ( 'NONE', #20113, 62.91752772691707207 ) ;
#7704=CARTESIAN_POINT ( 'NONE',  ( 0.000000000000000000, 0.000000000000000000, 112.9440587442963562 ) ) ;
#7707=VECTOR ( 'NONE', #5563, 1000.000000000000000 ) ;
#7713=LINE ( 'NONE', #3126, #3216 ) ;
#7714=VERTEX_POINT ( 'NONE', #5096 ) ;
#7716=DIRECTION ( 'NONE',  ( -0.000000000000000000, -0.000000000000000000, 1.000000000000000000 ) ) ;
#7717=EDGE_CURVE ( 'NONE', #9804, #14807, #479, .T. ) ;
#7719=DIRECTION ( 'NONE',  ( 0.000000000000000000, -1.000000000000000000, 0.000000000000000000 ) ) ;
#7722=LINE ( 'NONE', #4880, #14013 ) ;
#7724=DIRECTION ( 'NONE',  ( -0.3088643371590125697, 0.9511061040868803440, 0.000000000000000000 ) ) ;
#7725=VECTOR ( 'NONE', #877, 1000.000000000000000 ) ;
#7730=VECTOR ( 'NONE', #2354, 1000.000000000000000 ) ;
#7731=ORIENTED_EDGE ( 'NONE', *, *, #11017, .T. ) ;
#7732=ADVANCED_FACE ( 'NONE', ( #2121 ), #14691, .F. ) ;
#7733=VERTEX_POINT ( 'NONE', #3652 ) ;
#7734=EDGE_CURVE ( 'NONE', #9156, #16671, #11614, .T. ) ;
#7735=VERTEX_POINT ( 'NONE', #13234 ) ;
#7738=ORIENTED_EDGE ( 'NONE', *, *, #12166, .F. ) ;
#7739=FACE_OUTER_BOUND ( 'NONE', #1397, .T. ) ;
#7740=CARTESIAN_POINT ( 'NONE',  ( 67.36461649554532016, -39.84224160888924615, 248.9926560891072143 ) ) ;
#7741=LINE ( 'NONE', #20120, #8621 ) ;
#7742=LINE ( 'NONE', #16853, #12655 ) ;
#7743=VERTEX_POINT ( 'NONE', #14882 ) ;
#7747=ORIENTED_EDGE ( 'NONE', *, *, #20219, .F. ) ;
#7748=AXIS2_PLACEMENT_3D ( 'NONE', #20240, #8166, #3166 ) ;
#7749=EDGE_CURVE ( 'NONE', #7454, #13999, #2221, .T. ) ;
#7750=DIRECTION ( 'NONE',  ( -0.4999999999999888423, -0.8660254037844449249, -0.000000000000000000 ) ) ;
#7751=LINE ( 'NONE', #17384, #19241 ) ;
#7752=DIRECTION ( 'NONE',  ( -0.000000000000000000, -0.000000000000000000, 1.000000000000000000 ) ) ;
#7754=DIRECTION ( 'NONE',  ( -0.000000000000000000, -0.000000000000000000, 1.000000000000000000 ) ) ;
#7756=ORIENTED_EDGE ( 'NONE', *, *, #1535, .F. ) ;
#7757=FACE_BOUND ( 'NONE', #12267, .T. ) ;
#7758=VERTEX_POINT ( 'NONE', #9016 ) ;
#7760=ADVANCED_FACE ( 'NONE', ( #2418 ), #7486, .F. ) ;
#7763=ORIENTED_EDGE ( 'NONE', *, *, #15652, .F. ) ;
#7764=EDGE_CURVE ( 'NONE', #19299, #14265, #9986, .T. ) ;
#7769=VERTEX_POINT ( 'NONE', #5292 ) ;
#7770=DIRECTION ( 'NONE',  ( 1.000000000000000000, 0.000000000000000000, 0.000000000000000000 ) ) ;
#7771=DIRECTION ( 'NONE',  ( 1.000000000000000000, 0.000000000000000000, 0.000000000000000000 ) ) ;
#7772=EDGE_CURVE ( 'NONE', #9468, #11620, #18063, .T. ) ;
#7773=AXIS2_PLACEMENT_3D ( 'NONE', #8550, #14789, #14593 ) ;
#7775=CARTESIAN_POINT ( 'NONE',  ( -68.46530598706767989, 37.93579148621533648, 248.9926560891072143 ) ) ;
#7776=VECTOR ( 'NONE', #16767, 1000.000000000000000 ) ;
#7777=ORIENTED_EDGE ( 'NONE', *, *, #1420, .F. ) ;
#7786=ADVANCED_FACE ( 'NONE', ( #3743 ), #12078, .T. ) ;
#7788=ORIENTED_EDGE ( 'NONE', *, *, #9797, .F. ) ;
#7789=ORIENTED_EDGE ( 'NONE', *, *, #19162, .F. ) ;
#7791=AXIS2_PLACEMENT_3D ( 'NONE', #10495, #11823, #16748 ) ;
#7796=DIRECTION ( 'NONE',  ( 1.000000000000000000, 0.000000000000000000, 0.000000000000000000 ) ) ;
#7797=VECTOR ( 'NONE', #9864, 1000.000000000000000 ) ;
#7798=FACE_BOUND ( 'NONE', #8602, .T. ) ;
#7800=DIRECTION ( 'NONE',  ( 0.4999999999999979461, 0.8660254037844398178, 0.000000000000000000 ) ) ;
#7801=CYLINDRICAL_SURFACE ( 'NONE', #14834, 60.74260934110282051 ) ;
#7808=CARTESIAN_POINT ( 'NONE',  ( 0.000000000000000000, 0.000000000000000000, 293.5832628385307999 ) ) ;
#7813=EDGE_LOOP ( 'NONE', ( #2841, #19348, #8677 ) ) ;
#7816=ORIENTED_EDGE ( 'NONE', *, *, #14480, .T. ) ;
#7817=ORIENTED_EDGE ( 'NONE', *, *, #5035, .F. ) ;
#7818=VECTOR ( 'NONE', #5736, 1000.000000000000227 ) ;
#7819=AXIS2_PLACEMENT_3D ( 'NONE', #8826, #4223, #11689 ) ;
#7820=DIRECTION ( 'NONE',  ( 0.9396926207859082059, 0.3420201433256694901, 0.000000000000000000 ) ) ;
#7822=LINE ( 'NONE', #4559, #13045 ) ;
#7825=CARTESIAN_POINT ( 'NONE',  ( 19.23614321207236699, -57.61627707419557964, 293.5832628385307999 ) ) ;
#7827=CARTESIAN_POINT ( 'NONE',  ( -67.08601213326565471, -40.32479851956794192, 132.4711112102474146 ) ) ;
#7828=DIRECTION ( 'NONE',  ( -0.7660444431189792347, 0.6427876096865379196, 0.000000000000000000 ) ) ;
#7829=VERTEX_POINT ( 'NONE', #5386 ) ;
#7831=LINE ( 'NONE', #14076, #19805 ) ;
#7832=EDGE_LOOP ( 'NONE', ( #9581, #12896, #16262 ) ) ;
#7835=VERTEX_POINT ( 'NONE', #18340 ) ;
#7836=EDGE_CURVE ( 'NONE', #16766, #7758, #4314, .T. ) ;
#7838=ORIENTED_EDGE ( 'NONE', *, *, #10639, .T. ) ;
#7839=FACE_OUTER_BOUND ( 'NONE', #10566, .T. ) ;
#7841=CARTESIAN_POINT ( 'NONE',  ( 0.000000000000000000, 0.000000000000000000, 283.5832628385307999 ) ) ;
#7845=ORIENTED_EDGE ( 'NONE', *, *, #10494, .T. ) ;
#7846=VECTOR ( 'NONE', #12059, 1000.000000000000114 ) ;
#7847=DIRECTION ( 'NONE',  ( 0.000000000000000000, 0.000000000000000000, -1.000000000000000000 ) ) ;
#7848=LINE ( 'NONE', #11619, #5536 ) ;
#7849=ORIENTED_EDGE ( 'NONE', *, *, #2349, .T. ) ;
#7850=EDGE_CURVE ( 'NONE', #9758, #5816, #16804, .T. ) ;
#7853=DIRECTION ( 'NONE',  ( 0.000000000000000000, 0.000000000000000000, 1.000000000000000000 ) ) ;
#7856=CARTESIAN_POINT ( 'NONE',  ( 0.000000000000000000, 0.000000000000000000, 293.5832628385307999 ) ) ;
#7857=DIRECTION ( 'NONE',  ( 1.000000000000000000, 0.000000000000000000, 0.000000000000000000 ) ) ;
#7860=VERTEX_POINT ( 'NONE', #16905 ) ;
#7861=DIRECTION ( 'NONE',  ( -0.000000000000000000, -0.000000000000000000, 1.000000000000000000 ) ) ;
#7865=ADVANCED_FACE ( 'NONE', ( #2896 ), #13931, .T. ) ;
#7866=DIRECTION ( 'NONE',  ( 0.000000000000000000, 0.000000000000000000, -1.000000000000000000 ) ) ;
#7870=ORIENTED_EDGE ( 'NONE', *, *, #14431, .F. ) ;
#7872=CARTESIAN_POINT ( 'NONE',  ( -39.84224160888947353, -67.36461649554519227, 248.9926560891072143 ) ) ;
#7873=VECTOR ( 'NONE', #17689, 999.9999999999998863 ) ;
#7874=ADVANCED_FACE ( 'NONE', ( #12597 ), #1563, .F. ) ;
#7875=EDGE_CURVE ( 'NONE', #19407, #7835, #20176, .T. ) ;
#7877=CARTESIAN_POINT ( 'NONE',  ( 44.07268132743672595, 38.78191089773085309, 110.7293897666001214 ) ) ;
#7879=EDGE_LOOP ( 'NONE', ( #8665, #19810, #5330, #3624 ) ) ;
#7881=CARTESIAN_POINT ( 'NONE',  ( -51.36153797460868731, 59.06449708980215973, 132.4711112102474146 ) ) ;
#7882=FACE_OUTER_BOUND ( 'NONE', #11342, .T. ) ;
#7889=VERTEX_POINT ( 'NONE', #1460 ) ;
#7892=ORIENTED_EDGE ( 'NONE', *, *, #12134, .F. ) ;
#7894=FACE_BOUND ( 'NONE', #7285, .T. ) ;
#7898=DIRECTION ( 'NONE',  ( 1.000000000000000000, 0.000000000000000000, 0.000000000000000000 ) ) ;
#7900=EDGE_CURVE ( 'NONE', #1487, #15959, #17331, .T. ) ;
#7901=CARTESIAN_POINT ( 'NONE',  ( 77.21438937758502163, 12.78021302872874010, 132.4711112102474146 ) ) ;
#7902=EDGE_CURVE ( 'NONE', #1787, #14365, #14470, .T. ) ;
#7905=FACE_OUTER_BOUND ( 'NONE', #4305, .T. ) ;
#7906=DIRECTION ( 'NONE',  ( -0.000000000000000000, -0.000000000000000000, 1.000000000000000000 ) ) ;
#7908=EDGE_CURVE ( 'NONE', #4730, #4430, #6071, .T. ) ;
#7911=VECTOR ( 'NONE', #3535, 1000.000000000000000 ) ;
#7913=VERTEX_POINT ( 'NONE', #20071 ) ;
#7914=ORIENTED_EDGE ( 'NONE', *, *, #3980, .T. ) ;
#7915=ORIENTED_EDGE ( 'NONE', *, *, #1389, .T. ) ;
#7916=CARTESIAN_POINT ( 'NONE',  ( -55.16472960512350454, 30.25670013172272377, 293.5832628385307999 ) ) ;
#7917=FACE_OUTER_BOUND ( 'NONE', #3836, .T. ) ;
#7918=AXIS2_PLACEMENT_3D ( 'NONE', #8186, #14334, #14434 ) ;
#7924=LINE ( 'NONE', #4453, #20216 ) ;
#7925=CIRCLE ( 'NONE', #13459, 62.91752772691707207 ) ;
#7926=DIRECTION ( 'NONE',  ( 0.1736481776669273613, 0.9848077530122086864, 0.000000000000000000 ) ) ;
#7927=DIRECTION ( 'NONE',  ( 1.000000000000000000, 0.000000000000000000, 0.000000000000000000 ) ) ;
#7929=ORIENTED_EDGE ( 'NONE', *, *, #14238, .F. ) ;
#7932=ORIENTED_EDGE ( 'NONE', *, *, #9841, .F. ) ;
#7933=ORIENTED_EDGE ( 'NONE', *, *, #2845, .F. ) ;
#7934=VECTOR ( 'NONE', #1347, 1000.000000000000000 ) ;
#7938=CARTESIAN_POINT ( 'NONE',  ( 57.61823435390807902, 19.23677882349220880, 283.5832628385307999 ) ) ;
#7940=CARTESIAN_POINT ( 'NONE',  ( 0.000000000000000000, 0.000000000000000000, 283.5832628385307999 ) ) ;
#7941=VECTOR ( 'NONE', #194, 1000.000000000000000 ) ;
#7945=AXIS2_PLACEMENT_3D ( 'NONE', #12676, #9411, #14111 ) ;
#7946=FACE_OUTER_BOUND ( 'NONE', #6374, .T. ) ;
#7950=ORIENTED_EDGE ( 'NONE', *, *, #7147, .T. ) ;
#7951=DIRECTION ( 'NONE',  ( -0.000000000000000000, -0.000000000000000000, 1.000000000000000000 ) ) ;
#7952=DIRECTION ( 'NONE',  ( 1.000000000000000000, 0.000000000000000000, 0.000000000000000000 ) ) ;
#7954=CARTESIAN_POINT ( 'NONE',  ( 19.30071112029679625, -55.43188410062176530, 132.4711112102474146 ) ) ;
#7956=DIRECTION ( 'NONE',  ( 0.8660254037844398178, -0.4999999999999979461, 0.000000000000000000 ) ) ;
#7958=AXIS2_PLACEMENT_3D ( 'NONE', #5384, #6623, #17866 ) ;
#7959=FACE_OUTER_BOUND ( 'NONE', #10064, .T. ) ;
#7962=LINE ( 'NONE', #17594, #14800 ) ;
#7964=ORIENTED_EDGE ( 'NONE', *, *, #145, .T. ) ;
#7966=DIRECTION ( 'NONE',  ( -0.5000000000000069944, 0.8660254037844345998, 0.000000000000000000 ) ) ;
#7967=ADVANCED_FACE ( 'NONE', ( #129 ), #3000, .F. ) ;
#7973=( LENGTH_UNIT ( ) NAMED_UNIT ( * ) SI_UNIT ( .MILLI., .METRE. ) );
#7974=CARTESIAN_POINT ( 'NONE',  ( -14.39940464655760799, -76.92888220842480962, 132.4711112102474146 ) ) ;
#7975=CARTESIAN_POINT ( 'NONE',  ( -32.64570716507502368, 53.78543575132162857, 248.9926560891072143 ) ) ;
#7976=VECTOR ( 'NONE', #10089, 999.9999999999998863 ) ;
#7979=CARTESIAN_POINT ( 'NONE',  ( 73.82206860051529418, 25.99419088092216867, 111.4180192758973362 ) ) ;
#7981=DIRECTION ( 'NONE',  ( -0.8660254037844397068, 0.4999999999999978906, 0.000000000000000000 ) ) ;
#7983=DIRECTION ( 'NONE',  ( 0.000000000000000000, 0.000000000000000000, 1.000000000000000000 ) ) ;
#7986=DIRECTION ( 'NONE',  ( 0.000000000000000000, 0.000000000000000000, -1.000000000000000000 ) ) ;
#7988=ORIENTED_EDGE ( 'NONE', *, *, #2012, .F. ) ;
#7989=VECTOR ( 'NONE', #16666, 1000.000000000000000 ) ;
#7990=EDGE_LOOP ( 'NONE', ( #71, #10573, #18297, #13670 ) ) ;
#7991=ORIENTED_EDGE ( 'NONE', *, *, #17156, .F. ) ;
#7993=EDGE_CURVE ( 'NONE', #2635, #9958, #1766, .T. ) ;
#7994=ORIENTED_EDGE ( 'NONE', *, *, #3840, .F. ) ;
#7995=EDGE_CURVE ( 'NONE', #13722, #11567, #10962, .T. ) ;
#7999=VECTOR ( 'NONE', #1565, 1000.000000000000114 ) ;
#8001=DIRECTION ( 'NONE',  ( 0.000000000000000000, 0.000000000000000000, 1.000000000000000000 ) ) ;
#8004=VECTOR ( 'NONE', #18500, 1000.000000000000000 ) ;
#8005=LINE ( 'NONE', #14250, #3473 ) ;
#8008=CARTESIAN_POINT ( 'NONE',  ( -61.81362617575094021, 11.73417718768112294, 248.9926560891072143 ) ) ;
#8014=VECTOR ( 'NONE', #4608, 1000.000000000000114 ) ;
#8017=EDGE_CURVE ( 'NONE', #7913, #4516, #2278, .T. ) ;
#8019=EDGE_CURVE ( 'NONE', #2515, #19514, #635, .T. ) ;
#8022=AXIS2_PLACEMENT_3D ( 'NONE', #13940, #18450, #16917 ) ;
#8025=CARTESIAN_POINT ( 'NONE',  ( 60.22232964560483737, 7.948937137877944537, 283.5832628385307999 ) ) ;
#8030=DIRECTION ( 'NONE',  ( 0.000000000000000000, 0.000000000000000000, 1.000000000000000000 ) ) ;
#8032=CARTESIAN_POINT ( 'NONE',  ( -2.629322876227788264, -60.68773558783006905, 283.5832628385307999 ) ) ;
#8033=EDGE_LOOP ( 'NONE', ( #11884, #4691, #18337, #17189 ) ) ;
#8034=FACE_OUTER_BOUND ( 'NONE', #11066, .T. ) ;
#8040=EDGE_CURVE ( 'NONE', #6009, #13255, #8204, .T. ) ;
#8044=CARTESIAN_POINT ( 'NONE',  ( -67.36461649554505016, 39.84224160888970800, 110.9660488491356887 ) ) ;
#8045=EDGE_CURVE ( 'NONE', #9731, #20066, #17727, .T. ) ;
#8047=CARTESIAN_POINT ( 'NONE',  ( 60.08331549348424971, 8.939227532413909216, 283.5832628385307999 ) ) ;
#8048=ORIENTED_EDGE ( 'NONE', *, *, #18134, .F. ) ;
#8050=DIRECTION ( 'NONE',  ( 1.000000000000000000, 0.000000000000000000, 0.000000000000000000 ) ) ;
#8052=VERTEX_POINT ( 'NONE', #11574 ) ;
#8055=LINE ( 'NONE', #12762, #1936 ) ;
#8062=ORIENTED_EDGE ( 'NONE', *, *, #14116, .T. ) ;
#8065=ORIENTED_EDGE ( 'NONE', *, *, #11374, .F. ) ;
#8066=LINE ( 'NONE', #14106, #611 ) ;
#8067=VERTEX_POINT ( 'NONE', #3704 ) ;
#8068=FACE_OUTER_BOUND ( 'NONE', #19061, .T. ) ;
#8070=FACE_OUTER_BOUND ( 'NONE', #15331, .T. ) ;
#8071=AXIS2_PLACEMENT_3D ( 'NONE', #14682, #7206, #13425 ) ;
#8072=EDGE_LOOP ( 'NONE', ( #14392, #2095, #7193, #20203 ) ) ;
#8074=DIRECTION ( 'NONE',  ( 0.000000000000000000, 0.000000000000000000, -1.000000000000000000 ) ) ;
#8075=CARTESIAN_POINT ( 'NONE',  ( 37.09555676056997697, -45.48770046196272432, 132.4711112102474146 ) ) ;
#8078=ORIENTED_EDGE ( 'NONE', *, *, #16389, .F. ) ;
#8079=CARTESIAN_POINT ( 'NONE',  ( 48.17797692984161984, 36.99387960884179449, 283.5832628385307999 ) ) ;
#8080=DIRECTION ( 'NONE',  ( -0.000000000000000000, -0.000000000000000000, 1.000000000000000000 ) ) ;
#8082=CARTESIAN_POINT ( 'NONE',  ( -27.53920554013687649, -73.25972925305620720, 111.4180192758973931 ) ) ;
#8084=ORIENTED_EDGE ( 'NONE', *, *, #10979, .F. ) ;
#8089=VERTEX_POINT ( 'NONE', #14646 ) ;
#8090=ORIENTED_EDGE ( 'NONE', *, *, #15177, .F. ) ;
#8101=VECTOR ( 'NONE', #10796, 1000.000000000000000 ) ;
#8106=DIRECTION ( 'NONE',  ( 0.6427876096865353661, 0.7660444431189813441, 0.000000000000000000 ) ) ;
#8107=ADVANCED_FACE ( 'NONE', ( #14352 ), #13098, .F. ) ;
#8108=CARTESIAN_POINT ( 'NONE',  ( 28.15057869795588985, 51.51682027493075111, 110.9660488491356887 ) ) ;
#8111=ORIENTED_EDGE ( 'NONE', *, *, #772, .F. ) ;
#8113=LINE ( 'NONE', #3321, #14461 ) ;
#8116=VECTOR ( 'NONE', #4175, 1000.000000000000000 ) ;
#8117=CIRCLE ( 'NONE', #19552, 62.91752772691707207 ) ;
#8123=CARTESIAN_POINT ( 'NONE',  ( -25.99419088092141550, 73.82206860051556419, 111.4180192758973931 ) ) ;
#8124=DIRECTION ( 'NONE',  ( 0.7660444431189792347, -0.6427876096865379196, 0.000000000000000000 ) ) ;
#8127=VECTOR ( 'NONE', #2546, 1000.000000000000000 ) ;
#8128=CARTESIAN_POINT ( 'NONE',  ( 12.11787020633414080, 60.78082026081718681, 248.9926560891072143 ) ) ;
#8130=LINE ( 'NONE', #14379, #726 ) ;
#8132=EDGE_CURVE ( 'NONE', #14586, #2211, #7268, .T. ) ;
#8135=EDGE_CURVE ( 'NONE', #4473, #241, #18117, .T. ) ;
#8136=ORIENTED_EDGE ( 'NONE', *, *, #1276, .T. ) ;
#8141=VECTOR ( 'NONE', #19465, 1000.000000000000000 ) ;
#8143=VECTOR ( 'NONE', #19352, 1000.000000000000000 ) ;
#8145=EDGE_LOOP ( 'NONE', ( #14155, #8488, #7929, #16356 ) ) ;
#8146=FACE_OUTER_BOUND ( 'NONE', #5454, .T. ) ;
#8147=ADVANCED_FACE ( 'NONE', ( #15139 ), #4195, .F. ) ;
#8148=ORIENTED_EDGE ( 'NONE', *, *, #7274, .F. ) ;
#8149=PLANE ( 'NONE',  #2830 ) ;
#8151=CARTESIAN_POINT ( 'NONE',  ( -39.37628763770454299, -49.07263256785938665, 248.9926560891072143 ) ) ;
#8155=CARTESIAN_POINT ( 'NONE',  ( 51.77251465595239921, -31.77296517111717478, 283.5832628385307999 ) ) ;
#8156=VERTEX_POINT ( 'NONE', #2469 ) ;
#8157=CARTESIAN_POINT ( 'NONE',  ( 44.07268132743672595, 38.78191089773085309, 132.4711112102474146 ) ) ;
#8160=FACE_OUTER_BOUND ( 'NONE', #4059, .T. ) ;
#8164=EDGE_CURVE ( 'NONE', #18256, #9985, #2468, .T. ) ;
#8165=DIRECTION ( 'NONE',  ( 0.8660254037844363761, 0.5000000000000039968, 0.000000000000000000 ) ) ;
#8166=DIRECTION ( 'NONE',  ( 0.3088643371590157338, -0.9511061040868794558, 0.000000000000000000 ) ) ;
#8168=EDGE_CURVE ( 'NONE', #4702, #14818, #2772, .T. ) ;
#8171=ORIENTED_EDGE ( 'NONE', *, *, #763, .F. ) ;
#8172=ORIENTED_EDGE ( 'NONE', *, *, #1201, .F. ) ;
#8174=( GEOMETRIC_REPRESENTATION_CONTEXT ( 3 ) GLOBAL_UNCERTAINTY_ASSIGNED_CONTEXT ( ( #81 ) ) GLOBAL_UNIT_ASSIGNED_CONTEXT ( ( #12072, #11974, #1139 ) ) REPRESENTATION_CONTEXT ( 'NONE', 'WORKASPACE' ) );
#8175=VERTEX_POINT ( 'NONE', #8995 ) ;
#8178=CARTESIAN_POINT ( 'NONE',  ( 0.000000000000000000, 0.000000000000000000, 283.5832628385307999 ) ) ;
#8181=LINE ( 'NONE', #14427, #10168 ) ;
#8185=ORIENTED_EDGE ( 'NONE', *, *, #3358, .T. ) ;
#8186=CARTESIAN_POINT ( 'NONE',  ( 38.78191089773071809, -44.07268132743684674, 110.7293897666001214 ) ) ;
#8187=CARTESIAN_POINT ( 'NONE',  ( 0.000000000000000000, 0.000000000000000000, 293.5832628385307999 ) ) ;
#8188=PLANE ( 'NONE',  #16672 ) ;
#8189=VECTOR ( 'NONE', #6460, 999.9999999999998863 ) ;
#8190=CARTESIAN_POINT ( 'NONE',  ( -73.06915264522022824, -28.06281046684250313, 132.4711112102474146 ) ) ;
#8192=LINE ( 'NONE', #16079, #4864 ) ;
#8200=DIRECTION ( 'NONE',  ( 1.000000000000000000, 0.000000000000000000, 0.000000000000000000 ) ) ;
#8201=MANIFOLD_SOLID_BREP ( 'CirPattern4', #11315 ) ;
#8204=LINE ( 'NONE', #5344, #445 ) ;
#8205=DIRECTION ( 'NONE',  ( 0.000000000000000000, 0.000000000000000000, 1.000000000000000000 ) ) ;
#8208=VECTOR ( 'NONE', #13014, 1000.000000000000000 ) ;
#8209=CARTESIAN_POINT ( 'NONE',  ( -51.36153797460868731, 59.06449708980214552, 248.9926560891072143 ) ) ;
#8211=DIRECTION ( 'NONE',  ( 0.8660254037844450359, -0.4999999999999889533, 0.000000000000000000 ) ) ;
#8215=ORIENTED_EDGE ( 'NONE', *, *, #4775, .T. ) ;
#8222=EDGE_CURVE ( 'NONE', #7430, #934, #1949, .T. ) ;
#8224=CARTESIAN_POINT ( 'NONE',  ( 5.590028426173794251, 1.289614712049196976, 283.5832628385307999 ) ) ;
#8226=LINE ( 'NONE', #11093, #10393 ) ;
#8229=CARTESIAN_POINT ( 'NONE',  ( 0.000000000000000000, 0.000000000000000000, 283.5832628385307999 ) ) ;
#8232=CARTESIAN_POINT ( 'NONE',  ( 0.000000000000000000, 0.000000000000000000, 293.5832628385307999 ) ) ;
#8235=DIRECTION ( 'NONE',  ( 0.000000000000000000, 0.000000000000000000, -1.000000000000000000 ) ) ;
#8236=ORIENTED_EDGE ( 'NONE', *, *, #8607, .F. ) ;
#8240=LINE ( 'NONE', #12944, #6339 ) ;
#8244=ORIENTED_EDGE ( 'NONE', *, *, #7214, .T. ) ;
#8245=CARTESIAN_POINT ( 'NONE',  ( -23.22641211976288389, -56.12662799072081299, 283.5832628385307999 ) ) ;
#8249=ORIENTED_EDGE ( 'NONE', *, *, #1870, .F. ) ;
#8252=DIRECTION ( 'NONE',  ( 0.000000000000000000, 0.000000000000000000, -1.000000000000000000 ) ) ;
#8254=CARTESIAN_POINT ( 'NONE',  ( 59.06449708980163393, 51.36153797460926995, 110.7293897666001214 ) ) ;
#8255=DIRECTION ( 'NONE',  ( -0.1736481776669374644, 0.9848077530122069101, 0.000000000000000000 ) ) ;
#8256=LINE ( 'NONE', #14505, #13408 ) ;
#8259=AXIS2_PLACEMENT_3D ( 'NONE', #10951, #7476, #12176 ) ;
#8262=CARTESIAN_POINT ( 'NONE',  ( 0.000000000000000000, 0.000000000000000000, 132.4711112102474146 ) ) ;
#8264=ORIENTED_EDGE ( 'NONE', *, *, #2272, .T. ) ;
#8266=VERTEX_POINT ( 'NONE', #18091 ) ;
#8267=AXIS2_PLACEMENT_3D ( 'NONE', #4573, #4988, #12541 ) ;
#8269=DIRECTION ( 'NONE',  ( -0.000000000000000000, -0.000000000000000000, 1.000000000000000000 ) ) ;
#8270=CIRCLE ( 'NONE', #7945, 60.74260934110282051 ) ;
#8271=ORIENTED_EDGE ( 'NONE', *, *, #17109, .F. ) ;
#8272=EDGE_CURVE ( 'NONE', #3178, #20227, #13366, .T. ) ;
#8274=EDGE_CURVE ( 'NONE', #4648, #20212, #3873, .T. ) ;
#8282=VECTOR ( 'NONE', #271, 1000.000000000000114 ) ;
#8283=DIRECTION ( 'NONE',  ( -0.000000000000000000, -0.000000000000000000, 1.000000000000000000 ) ) ;
#8284=DIRECTION ( 'NONE',  ( -0.3747554100459928317, -0.9271237148521548344, 0.000000000000000000 ) ) ;
#8285=FACE_OUTER_BOUND ( 'NONE', #14544, .T. ) ;
#8286=ADVANCED_FACE ( 'NONE', ( #14816 ), #703, .F. ) ;
#8287=CARTESIAN_POINT ( 'NONE',  ( 0.000000000000000000, 0.000000000000000000, 248.9926560891072143 ) ) ;
#8288=LINE ( 'NONE', #12477, #1320 ) ;
#8293=EDGE_LOOP ( 'NONE', ( #9630, #13559, #887, #18637 ) ) ;
#8297=EDGE_CURVE ( 'NONE', #14124, #6346, #10301, .T. ) ;
#8298=CIRCLE ( 'NONE', #9276, 60.74260934110282051 ) ;
#8300=PLANE ( 'NONE',  #14687 ) ;
#8302=AXIS2_PLACEMENT_3D ( 'NONE', #2321, #16134, #17680 ) ;
#8303=ORIENTED_EDGE ( 'NONE', *, *, #15198, .T. ) ;
#8307=VERTEX_POINT ( 'NONE', #19817 ) ;
#8309=DIRECTION ( 'NONE',  ( -3.491481338843133355E-15, 1.000000000000000000, 0.000000000000000000 ) ) ;
#8313=CARTESIAN_POINT ( 'NONE',  ( 37.93579148621461883, 68.46530598706807780, 110.9660488491356887 ) ) ;
#8314=DIRECTION ( 'NONE',  ( -0.000000000000000000, -0.000000000000000000, 1.000000000000000000 ) ) ;
#8315=ORIENTED_EDGE ( 'NONE', *, *, #7836, .F. ) ;
#8318=ORIENTED_EDGE ( 'NONE', *, *, #16234, .T. ) ;
#8319=VECTOR ( 'NONE', #16585, 1000.000000000000000 ) ;
#8320=ORIENTED_EDGE ( 'NONE', *, *, #18557, .F. ) ;
#8321=EDGE_LOOP ( 'NONE', ( #16060, #454, #8813, #8568 ) ) ;
#8322=AXIS2_PLACEMENT_3D ( 'NONE', #19220, #8165, #15740 ) ;
#8323=LINE ( 'NONE', #14569, #3064 ) ;
#8325=DIRECTION ( 'NONE',  ( 0.000000000000000000, 1.000000000000000000, 0.000000000000000000 ) ) ;
#8327=CARTESIAN_POINT ( 'NONE',  ( -50.93469132750304595, -59.42266395395772349, 132.4711112102474146 ) ) ;
#8328=CARTESIAN_POINT ( 'NONE',  ( 0.000000000000000000, 0.000000000000000000, 293.5832628385307999 ) ) ;
#8330=CARTESIAN_POINT ( 'NONE',  ( 50.93469132750264095, 59.42266395395811429, 248.9926560891072143 ) ) ;
#8335=EDGE_CURVE ( 'NONE', #18849, #12537, #12590, .T. ) ;
#8336=CIRCLE ( 'NONE', #3121, 62.91752772691707207 ) ;
#8342=VERTEX_POINT ( 'NONE', #15015 ) ;
#8346=CARTESIAN_POINT ( 'NONE',  ( -20.74471755083563806, 59.39925916207565137, 293.5832628385307999 ) ) ;
#8347=EDGE_CURVE ( 'NONE', #7001, #17581, #5712, .T. ) ;
#8349=DIRECTION ( 'NONE',  ( 0.000000000000000000, 0.000000000000000000, 1.000000000000000000 ) ) ;
#8355=DIRECTION ( 'NONE',  ( -0.9848077530122067991, -0.1736481776669374366, 0.000000000000000000 ) ) ;
#8358=DIRECTION ( 'NONE',  ( 1.000000000000000000, 0.000000000000000000, 0.000000000000000000 ) ) ;
#8359=EDGE_CURVE ( 'NONE', #5887, #19198, #9663, .T. ) ;
#8362=LINE ( 'NONE', #14803, #16740 ) ;
#8364=ORIENTED_EDGE ( 'NONE', *, *, #6918, .F. ) ;
#8368=ORIENTED_EDGE ( 'NONE', *, *, #3616, .F. ) ;
#8375=AXIS2_PLACEMENT_3D ( 'NONE', #11212, #9585, #9282 ) ;
#8376=DIRECTION ( 'NONE',  ( -0.7881095627315619634, -0.6155349844899687950, 0.000000000000000000 ) ) ;
#8379=AXIS2_PLACEMENT_3D ( 'NONE', #12534, #470, #17669 ) ;
#8382=CARTESIAN_POINT ( 'NONE',  ( -58.03804081968160489, 8.833100819208169696, 112.0427633081292385 ) ) ;
#8384=ORIENTED_EDGE ( 'NONE', *, *, #8863, .F. ) ;
#8387=EDGE_CURVE ( 'NONE', #3256, #9877, #1412, .T. ) ;
#8388=CARTESIAN_POINT ( 'NONE',  ( 62.09913334491123749, 10.11498556985180031, 293.5832628385307999 ) ) ;
#8390=VECTOR ( 'NONE', #1821, 1000.000000000000000 ) ;
#8391=EDGE_CURVE ( 'NONE', #4335, #8743, #7439, .T. ) ;
#8392=ORIENTED_EDGE ( 'NONE', *, *, #4656, .T. ) ;
#8393=EDGE_CURVE ( 'NONE', #2297, #19280, #1513, .T. ) ;
#8396=CARTESIAN_POINT ( 'NONE',  ( 40.28046525994349736, 45.46865632508086463, 293.5832628385307999 ) ) ;
#8398=ORIENTED_EDGE ( 'NONE', *, *, #18811, .T. ) ;
#8403=CARTESIAN_POINT ( 'NONE',  ( 60.08331549348424971, 8.939227532413909216, 293.5832628385307999 ) ) ;
#8404=EDGE_CURVE ( 'NONE', #5478, #18696, #18295, .T. ) ;
#8405=DIRECTION ( 'NONE',  ( 0.000000000000000000, 0.000000000000000000, -1.000000000000000000 ) ) ;
#8409=ORIENTED_EDGE ( 'NONE', *, *, #16057, .T. ) ;
#8411=CARTESIAN_POINT ( 'NONE',  ( 45.46865632508072963, -40.28046525994365368, 293.5832628385307999 ) ) ;
#8413=LINE ( 'NONE', #6980, #6306 ) ;
#8414=EDGE_CURVE ( 'NONE', #4682, #10750, #7700, .T. ) ;
#8416=CARTESIAN_POINT ( 'NONE',  ( 0.000000000000000000, 0.000000000000000000, 0.000000000000000000 ) ) ;
#8418=DIRECTION ( 'NONE',  ( 1.000000000000000000, 0.000000000000000000, 0.000000000000000000 ) ) ;
#8419=ORIENTED_EDGE ( 'NONE', *, *, #9225, .T. ) ;
#8420=EDGE_CURVE ( 'NONE', #12185, #11142, #2483, .T. ) ;
#8422=ADVANCED_FACE ( 'NONE', ( #1310 ), #13677, .F. ) ;
#8423=ORIENTED_EDGE ( 'NONE', *, *, #14219, .F. ) ;
#8425=ORIENTED_EDGE ( 'NONE', *, *, #17504, .F. ) ;
#8429=LINE ( 'NONE', #2394, #1455 ) ;
#8430=DIRECTION ( 'NONE',  ( -0.6692498792541753394, -0.7430374143461900838, 0.000000000000000000 ) ) ;
#8431=LINE ( 'NONE', #6605, #18958 ) ;
#8432=EDGE_LOOP ( 'NONE', ( #730, #1344, #5418, #113 ) ) ;
#8433=CARTESIAN_POINT ( 'NONE',  ( 0.000000000000000000, 0.000000000000000000, 283.5832628385307999 ) ) ;
#8436=LINE ( 'NONE', #14579, #17956 ) ;
#8438=CARTESIAN_POINT ( 'NONE',  ( 59.51724408343574879, -12.14957802882732452, 293.5832628385307999 ) ) ;
#8440=ORIENTED_EDGE ( 'NONE', *, *, #15757, .F. ) ;
#8441=VECTOR ( 'NONE', #19148, 1000.000000000000114 ) ;
#8442=ORIENTED_EDGE ( 'NONE', *, *, #19307, .T. ) ;
#8445=ORIENTED_EDGE ( 'NONE', *, *, #7011, .F. ) ;
#8446=VECTOR ( 'NONE', #19666, 1000.000000000000000 ) ;
#8447=ORIENTED_EDGE ( 'NONE', *, *, #19281, .T. ) ;
#8448=AXIS2_PLACEMENT_3D ( 'NONE', #19129, #5116, #6249 ) ;
#8449=CARTESIAN_POINT ( 'NONE',  ( -14.39940464655760799, -76.92888220842480962, 248.9926560891072143 ) ) ;
#8450=VECTOR ( 'NONE', #7719, 1000.000000000000000 ) ;
#8451=CARTESIAN_POINT ( 'NONE',  ( 67.36461649554532016, -39.84224160888924615, 132.4711112102474146 ) ) ;
#8452=PLANE ( 'NONE',  #7773 ) ;
#8454=DIRECTION ( 'NONE',  ( -0.8479630283625716469, 0.5300553768524345344, 0.000000000000000000 ) ) ;
#8455=DIRECTION ( 'NONE',  ( -0.000000000000000000, -0.000000000000000000, 1.000000000000000000 ) ) ;
#8456=ORIENTED_EDGE ( 'NONE', *, *, #11638, .T. ) ;
#8457=CARTESIAN_POINT ( 'NONE',  ( 0.000000000000000000, 0.000000000000000000, 293.5832628385307999 ) ) ;
#8460=CARTESIAN_POINT ( 'NONE',  ( 0.000000000000000000, 62.91752772691707207, 248.9926560891072143 ) ) ;
#8463=DIRECTION ( 'NONE',  ( 1.000000000000000000, 0.000000000000000000, 0.000000000000000000 ) ) ;
#8466=VECTOR ( 'NONE', #3455, 1000.000000000000227 ) ;
#8467=ORIENTED_EDGE ( 'NONE', *, *, #19270, .T. ) ;
#8470=ORIENTED_EDGE ( 'NONE', *, *, #18913, .F. ) ;
#8471=VERTEX_POINT ( 'NONE', #2746 ) ;
#8472=DIRECTION ( 'NONE',  ( 0.000000000000000000, 0.000000000000000000, 1.000000000000000000 ) ) ;
#8473=ORIENTED_EDGE ( 'NONE', *, *, #16277, .F. ) ;
#8485=CARTESIAN_POINT ( 'NONE',  ( 53.40245231972179596, 28.94983032429848535, 293.5832628385307999 ) ) ;
#8487=CARTESIAN_POINT ( 'NONE',  ( 60.72073886220397299, -1.629865514042299512, 283.5832628385307999 ) ) ;
#8488=ORIENTED_EDGE ( 'NONE', *, *, #13456, .T. ) ;
#8490=DIRECTION ( 'NONE',  ( -0.000000000000000000, -0.000000000000000000, 1.000000000000000000 ) ) ;
#8493=ORIENTED_EDGE ( 'NONE', *, *, #12992, .T. ) ;
#8495=CARTESIAN_POINT ( 'NONE',  ( 32.64570716507540737, -53.78543575132140830, 293.5832628385307999 ) ) ;
#8496=CARTESIAN_POINT ( 'NONE',  ( 4.196299268919061021, 3.911853314815666671, 293.5832628385307999 ) ) ;
#8497=EDGE_LOOP ( 'NONE', ( #13132, #20230, #7178, #7892 ) ) ;
#8504=ORIENTED_EDGE ( 'NONE', *, *, #15223, .T. ) ;
#8505=ADVANCED_FACE ( 'NONE', ( #3156 ), #15634, .T. ) ;
#8513=VECTOR ( 'NONE', #18216, 1000.000000000000114 ) ;
#8516=CARTESIAN_POINT ( 'NONE',  ( -12.78021302872797449, 77.21438937758516374, 248.9926560891072143 ) ) ;
#8517=LINE ( 'NONE', #10055, #11717 ) ;
#8519=ORIENTED_EDGE ( 'NONE', *, *, #8391, .T. ) ;
#8523=AXIS2_PLACEMENT_3D ( 'NONE', #14799, #3854, #10099 ) ;
#8524=VECTOR ( 'NONE', #2350, 1000.000000000000000 ) ;
#8526=ORIENTED_EDGE ( 'NONE', *, *, #15392, .T. ) ;
#8529=EDGE_CURVE ( 'NONE', #20114, #3604, #19111, .T. ) ;
#8531=CARTESIAN_POINT ( 'NONE',  ( 36.99387960884163107, -48.17797692984174063, 283.5832628385307999 ) ) ;
#8532=LINE ( 'NONE', #6705, #3551 ) ;
#8533=LINE ( 'NONE', #2304, #19586 ) ;
#8535=CARTESIAN_POINT ( 'NONE',  ( 48.17959877923549072, 36.99514631729036296, 283.5832628385307999 ) ) ;
#8537=VECTOR ( 'NONE', #10763, 1000.000000000000000 ) ;
#8538=LINE ( 'NONE', #14868, #6611 ) ;
#8540=AXIS2_PLACEMENT_3D ( 'NONE', #7299, #8635, #19776 ) ;
#8541=FACE_OUTER_BOUND ( 'NONE', #14074, .T. ) ;
#8542=EDGE_LOOP ( 'NONE', ( #16915, #11105, #7777, #9835 ) ) ;
#8543=VERTEX_POINT ( 'NONE', #1713 ) ;
#8544=ORIENTED_EDGE ( 'NONE', *, *, #547, .F. ) ;
#8546=FACE_OUTER_BOUND ( 'NONE', #4295, .T. ) ;
#8548=DIRECTION ( 'NONE',  ( 0.000000000000000000, 0.000000000000000000, -1.000000000000000000 ) ) ;
#8549=CARTESIAN_POINT ( 'NONE',  ( 28.06680738835026290, -53.87178215532764369, 283.5832628385307999 ) ) ;
#8550=CARTESIAN_POINT ( 'NONE',  ( 50.13752642112827829, 30.53958573130925558, 110.9660488491356887 ) ) ;
#8551=ORIENTED_EDGE ( 'NONE', *, *, #13629, .T. ) ;
#8552=CARTESIAN_POINT ( 'NONE',  ( -73.25972925305609351, 27.53920554013712874, 248.9926560891072143 ) ) ;
#8553=DIRECTION ( 'NONE',  ( 0.3420201433256662704, 0.9396926207859092051, 0.000000000000000000 ) ) ;
#8557=CYLINDRICAL_SURFACE ( 'NONE', #4456, 60.74260934110282051 ) ;
#8558=CYLINDRICAL_SURFACE ( 'NONE', #4210, 60.74260934110282051 ) ;
#8560=LINE ( 'NONE', #14802, #2865 ) ;
#8562=PLANE ( 'NONE',  #1861 ) ;
#8564=DIRECTION ( 'NONE',  ( -3.491481338843133355E-15, 1.000000000000000000, 0.000000000000000000 ) ) ;
#8568=ORIENTED_EDGE ( 'NONE', *, *, #11419, .T. ) ;
#8570=ORIENTED_EDGE ( 'NONE', *, *, #11030, .F. ) ;
#8572=CIRCLE ( 'NONE', #20003, 62.91752772691707207 ) ;
#8575=CARTESIAN_POINT ( 'NONE',  ( -5.693982670708905403, 0.7000608949449642626, 293.5832628385307999 ) ) ;
#8578=ORIENTED_EDGE ( 'NONE', *, *, #3968, .F. ) ;
#8579=CARTESIAN_POINT ( 'NONE',  ( 14.39940464655707331, 76.92888220842492331, 112.0427633081292953 ) ) ;
#8581=AXIS2_PLACEMENT_3D ( 'NONE', #18106, #915, #16576 ) ;
#8584=DIRECTION ( 'NONE',  ( 1.000000000000000000, 0.000000000000000000, 0.000000000000000000 ) ) ;
#8587=DIRECTION ( 'NONE',  ( 0.5000000000000009992, -0.8660254037844380415, -0.000000000000000000 ) ) ;
#8588=AXIS2_PLACEMENT_3D ( 'NONE', #11444, #8269, #16260 ) ;
#8594=LINE ( 'NONE', #11751, #6656 ) ;
#8595=ORIENTED_EDGE ( 'NONE', *, *, #14270, .T. ) ;
#8596=EDGE_LOOP ( 'NONE', ( #8986, #15082, #7016 ) ) ;
#8597=VECTOR ( 'NONE', #10822, 1000.000000000000000 ) ;
#8598=AXIS2_PLACEMENT_3D ( 'NONE', #1920, #1815, #17271 ) ;
#8600=PLANE ( 'NONE',  #14030 ) ;
#8601=LINE ( 'NONE', #14932, #18186 ) ;
#8602=EDGE_LOOP ( 'NONE', ( #14585, #15596, #11150 ) ) ;
#8606=ORIENTED_EDGE ( 'NONE', *, *, #601, .T. ) ;
#8607=EDGE_CURVE ( 'NONE', #19610, #16066, #12653, .T. ) ;
#8610=DIRECTION ( 'NONE',  ( 1.000000000000000000, 0.000000000000000000, 0.000000000000000000 ) ) ;
#8612=CARTESIAN_POINT ( 'NONE',  ( -1.629865514042508456, -60.72073886220396588, 293.5832628385307999 ) ) ;
#8613=FACE_OUTER_BOUND ( 'NONE', #3393, .T. ) ;
#8614=EDGE_LOOP ( 'NONE', ( #6821, #3137, #4261, #3866 ) ) ;
#8621=VECTOR ( 'NONE', #8964, 1000.000000000000114 ) ;
#8624=VERTEX_POINT ( 'NONE', #12599 ) ;
#8625=CARTESIAN_POINT ( 'NONE',  ( 17.50000000000001066, 0.000000000000000000, 4.999999999999948486 ) ) ;
#8627=DIRECTION ( 'NONE',  ( -0.000000000000000000, -0.000000000000000000, 1.000000000000000000 ) ) ;
#8633=DIRECTION ( 'NONE',  ( 0.000000000000000000, 0.000000000000000000, -1.000000000000000000 ) ) ;
#8634=VECTOR ( 'NONE', #3023, 1000.000000000000000 ) ;
#8635=DIRECTION ( 'NONE',  ( 0.000000000000000000, 0.000000000000000000, 1.000000000000000000 ) ) ;
#8637=ORIENTED_EDGE ( 'NONE', *, *, #10730, .T. ) ;
#8638=EDGE_CURVE ( 'NONE', #2266, #13730, #3310, .T. ) ;
#8639=EDGE_CURVE ( 'NONE', #12535, #3408, #18160, .T. ) ;
#8641=ORIENTED_EDGE ( 'NONE', *, *, #9875, .F. ) ;
#8642=ORIENTED_EDGE ( 'NONE', *, *, #14102, .T. ) ;
#8650=ORIENTED_EDGE ( 'NONE', *, *, #8272, .F. ) ;
#8652=CARTESIAN_POINT ( 'NONE',  ( -40.32479851956768613, 67.08601213326579682, 248.9926560891072143 ) ) ;
#8654=ORIENTED_EDGE ( 'NONE', *, *, #18633, .T. ) ;
#8655=CARTESIAN_POINT ( 'NONE',  ( 41.48948842197119546, -47.29944656917770374, 293.5832628385307999 ) ) ;
#8656=DIRECTION ( 'NONE',  ( 0.9271237148521548344, -0.3747554100459928317, 0.000000000000000000 ) ) ;
#8657=CARTESIAN_POINT ( 'NONE',  ( -58.69016442926521648, -1.379293853801960124, 132.4711112102474146 ) ) ;
#8658=AXIS2_PLACEMENT_3D ( 'NONE', #710, #19440, #13375 ) ;
#8659=DIRECTION ( 'NONE',  ( 0.9848077530122097967, -0.1736481776669206722, 0.000000000000000000 ) ) ;
#8660=EDGE_CURVE ( 'NONE', #18107, #6039, #14043, .T. ) ;
#8662=DIRECTION ( 'NONE',  ( -0.000000000000000000, -0.000000000000000000, 1.000000000000000000 ) ) ;
#8663=VERTEX_POINT ( 'NONE', #18659 ) ;
#8665=ORIENTED_EDGE ( 'NONE', *, *, #6398, .F. ) ;
#8668=VERTEX_POINT ( 'NONE', #9335 ) ;
#8670=EDGE_LOOP ( 'NONE', ( #6831, #14018, #28, #8215 ) ) ;
#8672=LINE ( 'NONE', #7149, #9434 ) ;
#8673=DIRECTION ( 'NONE',  ( 1.000000000000000000, 0.000000000000000000, 0.000000000000000000 ) ) ;
#8675=FACE_OUTER_BOUND ( 'NONE', #17293, .T. ) ;
#8677=ORIENTED_EDGE ( 'NONE', *, *, #14413, .F. ) ;
#8680=VECTOR ( 'NONE', #10600, 1000.000000000000000 ) ;
#8682=FACE_OUTER_BOUND ( 'NONE', #12219, .T. ) ;
#8683=VERTEX_POINT ( 'NONE', #14354 ) ;
#8684=CARTESIAN_POINT ( 'NONE',  ( 7.948937137877743808, -60.22232964560488000, 293.5832628385307999 ) ) ;
#8686=PLANE ( 'NONE',  #3351 ) ;
#8687=ORIENTED_EDGE ( 'NONE', *, *, #4686, .F. ) ;
#8688=DIRECTION ( 'NONE',  ( -0.000000000000000000, -0.000000000000000000, 1.000000000000000000 ) ) ;
#8693=AXIS2_PLACEMENT_3D ( 'NONE', #7940, #14191, #17372 ) ;
#8696=CARTESIAN_POINT ( 'NONE',  ( -60.83768308848345185, 49.24833719034248958, 132.4711112102474146 ) ) ;
#8697=AXIS2_PLACEMENT_3D ( 'NONE', #13061, #7037, #982 ) ;
#8699=ORIENTED_EDGE ( 'NONE', *, *, #13672, .T. ) ;
#8702=VECTOR ( 'NONE', #17280, 1000.000000000000114 ) ;
#8704=DIRECTION ( 'NONE',  ( 1.000000000000000000, 0.000000000000000000, -0.000000000000000000 ) ) ;
#8705=DIRECTION ( 'NONE',  ( -0.1736481776669172583, -0.9848077530122103518, 0.000000000000000000 ) ) ;
#8707=CARTESIAN_POINT ( 'NONE',  ( 59.58067424803626722, -20.21777810286697985, 248.9926560891072143 ) ) ;
#8708=CARTESIAN_POINT ( 'NONE',  ( -3.123743752083685266, 4.811834253408552087, 293.5832628385307999 ) ) ;
#8710=DIRECTION ( 'NONE',  ( -0.000000000000000000, -0.000000000000000000, 1.000000000000000000 ) ) ;
#8713=LINE ( 'NONE', #11681, #16421 ) ;
#8715=ORIENTED_EDGE ( 'NONE', *, *, #7993, .T. ) ;
#8717=CARTESIAN_POINT ( 'NONE',  ( 0.8220851292435327196, 58.69016442926522359, 248.9926560891072143 ) ) ;
#8719=LINE ( 'NONE', #13311, #20035 ) ;
#8721=EDGE_CURVE ( 'NONE', #3127, #11536, #6382, .T. ) ;
#8722=DIRECTION ( 'NONE',  ( -0.1390141521205912334, 0.9902903945359629034, 0.000000000000000000 ) ) ;
#8724=CARTESIAN_POINT ( 'NONE',  ( 5.111158570922254896, -2.605298826210304064, 293.5832628385307999 ) ) ;
#8725=PLANE ( 'NONE',  #5899 ) ;
#8727=DIRECTION ( 'NONE',  ( -0.000000000000000000, -0.000000000000000000, 1.000000000000000000 ) ) ;
#8732=DIRECTION ( 'NONE',  ( -0.7881095627315599650, -0.6155349844899714595, 0.000000000000000000 ) ) ;
#8733=ORIENTED_EDGE ( 'NONE', *, *, #1685, .T. ) ;
#8734=VECTOR ( 'NONE', #15260, 1000.000000000000114 ) ;
#8739=ORIENTED_EDGE ( 'NONE', *, *, #9357, .T. ) ;
#8741=DIRECTION ( 'NONE',  ( -0.9902903945359624593, -0.1390141521205945918, 0.000000000000000000 ) ) ;
#8743=VERTEX_POINT ( 'NONE', #12164 ) ;
#8744=ADVANCED_FACE ( 'NONE', ( #18321 ), #13703, .F. ) ;
#8746=CARTESIAN_POINT ( 'NONE',  ( 78.26059000578312919, -0.8220851292427129309, 248.9926560891072143 ) ) ;
#8751=VECTOR ( 'NONE', #1753, 1000.000000000000000 ) ;
#8752=LINE ( 'NONE', #7318, #10011 ) ;
#8754=CARTESIAN_POINT ( 'NONE',  ( -60.83768308848343764, 49.24833719034248958, 110.7293897666001214 ) ) ;
#8756=DIRECTION ( 'NONE',  ( -0.6155349844899689060, 0.7881095627315620744, 0.000000000000000000 ) ) ;
#8758=EDGE_CURVE ( 'NONE', #7379, #18614, #15043, .T. ) ;
#8761=ORIENTED_EDGE ( 'NONE', *, *, #11040, .F. ) ;
#8762=AXIS2_PLACEMENT_3D ( 'NONE', #1639, #1729, #14005 ) ;
#8763=VECTOR ( 'NONE', #13572, 1000.000000000000227 ) ;
#8764=ORIENTED_EDGE ( 'NONE', *, *, #9766, .F. ) ;
#8765=FACE_OUTER_BOUND ( 'NONE', #16186, .T. ) ;
#8768=EDGE_LOOP ( 'NONE', ( #11204, #16683, #17809 ) ) ;
#8769=DIRECTION ( 'NONE',  ( -0.000000000000000000, -0.000000000000000000, 1.000000000000000000 ) ) ;
#8772=DIRECTION ( 'NONE',  ( 1.000000000000000000, 0.000000000000000000, 0.000000000000000000 ) ) ;
#8773=FACE_OUTER_BOUND ( 'NONE', #5212, .T. ) ;
#8774=EDGE_CURVE ( 'NONE', #5714, #3545, #7180, .T. ) ;
#8775=EDGE_LOOP ( 'NONE', ( #8924, #1557, #9935, #1162 ) ) ;
#8777=LINE ( 'NONE', #4276, #8127 ) ;
#8778=VECTOR ( 'NONE', #11963, 999.9999999999998863 ) ;
#8780=VECTOR ( 'NONE', #10916, 1000.000000000000114 ) ;
#8781=EDGE_CURVE ( 'NONE', #4188, #19638, #13807, .T. ) ;
#8782=DIRECTION ( 'NONE',  ( 1.000000000000000000, 0.000000000000000000, -0.000000000000000000 ) ) ;
#8785=EDGE_LOOP ( 'NONE', ( #9009, #6044, #18108, #6614 ) ) ;
#8788=CARTESIAN_POINT ( 'NONE',  ( -50.41613078340781584, 30.05702882063080494, 110.9660488491356887 ) ) ;
#8790=DIRECTION ( 'NONE',  ( 0.9993852124581887875, -0.03505990758545544927, 0.000000000000000000 ) ) ;
#8792=ORIENTED_EDGE ( 'NONE', *, *, #6227, .F. ) ;
#8793=EDGE_LOOP ( 'NONE', ( #12051, #4289, #9782, #4782 ) ) ;
#8794=LINE ( 'NONE', #4189, #13997 ) ;
#8796=CIRCLE ( 'NONE', #950, 60.74260934110282051 ) ;
#8797=DIRECTION ( 'NONE',  ( -0.000000000000000000, -0.000000000000000000, 1.000000000000000000 ) ) ;
#8803=CARTESIAN_POINT ( 'NONE',  ( 40.28046525994349736, 45.46865632508086463, 293.5832628385307999 ) ) ;
#8804=CARTESIAN_POINT ( 'NONE',  ( 77.31114765718494652, -12.23146955673620084, 248.9926560891072143 ) ) ;
#8808=CARTESIAN_POINT ( 'NONE',  ( 0.000000000000000000, 0.000000000000000000, 248.9926560891072143 ) ) ;
#8810=ORIENTED_EDGE ( 'NONE', *, *, #13356, .T. ) ;
#8811=DIRECTION ( 'NONE',  ( -0.9902903945359630145, -0.1390141521205912334, 0.000000000000000000 ) ) ;
#8813=ORIENTED_EDGE ( 'NONE', *, *, #13431, .T. ) ;
#8815=VERTEX_POINT ( 'NONE', #19647 ) ;
#8816=VECTOR ( 'NONE', #18717, 1000.000000000000000 ) ;
#8817=DIRECTION ( 'NONE',  ( -0.000000000000000000, -0.000000000000000000, 1.000000000000000000 ) ) ;
#8822=CARTESIAN_POINT ( 'NONE',  ( 79.75827554147308263, 0.000000000000000000, 293.5832628385307999 ) ) ;
#8823=DIRECTION ( 'NONE',  ( -0.000000000000000000, -0.000000000000000000, 1.000000000000000000 ) ) ;
#8825=PLANE ( 'NONE',  #3789 ) ;
#8826=CARTESIAN_POINT ( 'NONE',  ( -78.26059000578311498, 0.8220851292432594937, 112.7772637782949516 ) ) ;
#8827=ADVANCED_FACE ( 'NONE', ( #5637 ), #2470, .F. ) ;
#8828=ORIENTED_EDGE ( 'NONE', *, *, #17763, .F. ) ;
#8833=DIRECTION ( 'NONE',  ( -0.7430374143461878633, 0.6692498792541777819, 0.000000000000000000 ) ) ;
#8842=CIRCLE ( 'NONE', #11131, 62.91752772691707207 ) ;
#8844=LINE ( 'NONE', #12106, #10701 ) ;
#8845=ORIENTED_EDGE ( 'NONE', *, *, #4258, .F. ) ;
#8846=AXIS2_PLACEMENT_3D ( 'NONE', #4127, #18147, #10358 ) ;
#8847=DIRECTION ( 'NONE',  ( -0.9781142164131917394, 0.2080686897406911207, 0.000000000000000000 ) ) ;
#8849=ADVANCED_FACE ( 'NONE', ( #5948, #18425 ), #7463, .F. ) ;
#8851=DIRECTION ( 'NONE',  ( -0.1736481776669374644, 0.9848077530122066880, -0.000000000000000000 ) ) ;
#8857=ORIENTED_EDGE ( 'NONE', *, *, #19418, .T. ) ;
#8858=EDGE_CURVE ( 'NONE', #11398, #15547, #10627, .T. ) ;
#8860=ORIENTED_EDGE ( 'NONE', *, *, #9863, .F. ) ;
#8861=EDGE_CURVE ( 'NONE', #7743, #14775, #18522, .T. ) ;
#8862=ORIENTED_EDGE ( 'NONE', *, *, #11250, .T. ) ;
#8863=EDGE_CURVE ( 'NONE', #13278, #9985, #7670, .T. ) ;
#8866=ORIENTED_EDGE ( 'NONE', *, *, #18134, .T. ) ;
#8867=CARTESIAN_POINT ( 'NONE',  ( 0.000000000000000000, 0.000000000000000000, 283.5832628385307999 ) ) ;
#8869=DIRECTION ( 'NONE',  ( -0.000000000000000000, -0.000000000000000000, 1.000000000000000000 ) ) ;
#8870=CARTESIAN_POINT ( 'NONE',  ( -32.62092819947992695, -51.24245927909985454, 293.5832628385307999 ) ) ;
#8871=ORIENTED_EDGE ( 'NONE', *, *, #14113, .T. ) ;
#8872=EDGE_CURVE ( 'NONE', #10010, #13503, #18837, .T. ) ;
#8874=DIRECTION ( 'NONE',  ( -0.000000000000000000, -0.000000000000000000, 1.000000000000000000 ) ) ;
#8875=DIRECTION ( 'NONE',  ( -0.9511061040868794558, -0.3088643371590157338, 0.000000000000000000 ) ) ;
#8876=ORIENTED_EDGE ( 'NONE', *, *, #4494, .F. ) ;
#8877=AXIS2_PLACEMENT_3D ( 'NONE', #4748, #3511, #8106 ) ;
#8878=DIRECTION ( 'NONE',  ( -0.8660254037844344888, -0.5000000000000069944, 0.000000000000000000 ) ) ;
#8879=LINE ( 'NONE', #1205, #6226 ) ;
#8881=ORIENTED_EDGE ( 'NONE', *, *, #10331, .T. ) ;
#8883=DIRECTION ( 'NONE',  ( -0.000000000000000000, -0.000000000000000000, 1.000000000000000000 ) ) ;
#8884=EDGE_LOOP ( 'NONE', ( #3597, #3608, #19886, #10057 ) ) ;
#8885=EDGE_CURVE ( 'NONE', #7238, #2129, #15662, .T. ) ;
#8886=EDGE_CURVE ( 'NONE', #15222, #6324, #12678, .T. ) ;
#8887=ORIENTED_EDGE ( 'NONE', *, *, #2310, .F. ) ;
#8889=ADVANCED_FACE ( 'NONE', ( #1439 ), #6257, .T. ) ;
#8891=VERTEX_POINT ( 'NONE', #4822 ) ;
#8893=DIRECTION ( 'NONE',  ( -0.000000000000000000, -0.000000000000000000, 1.000000000000000000 ) ) ;
#8894=AXIS2_PLACEMENT_3D ( 'NONE', #19421, #2705, #18253 ) ;
#8896=CARTESIAN_POINT ( 'NONE',  ( -49.67518383744793908, 60.47951622432801599, 248.9926560891072143 ) ) ;
#8897=DIRECTION ( 'NONE',  ( -0.000000000000000000, -0.000000000000000000, 1.000000000000000000 ) ) ;
#8899=PLANE ( 'NONE',  #6029 ) ;
#8901=PLANE ( 'NONE',  #17546 ) ;
#8902=DIRECTION ( 'NONE',  ( -0.000000000000000000, -0.000000000000000000, 1.000000000000000000 ) ) ;
#8908=AXIS2_PLACEMENT_3D ( 'NONE', #5966, #9229, #12186 ) ;
#8909=ADVANCED_FACE ( 'NONE', ( #15862 ), #17199, .F. ) ;
#8910=VERTEX_POINT ( 'NONE', #7872 ) ;
#8911=ORIENTED_EDGE ( 'NONE', *, *, #13431, .F. ) ;
#8913=ORIENTED_EDGE ( 'NONE', *, *, #16912, .T. ) ;
#8914=EDGE_CURVE ( 'NONE', #11201, #14920, #16217, .T. ) ;
#8917=ORIENTED_EDGE ( 'NONE', *, *, #8017, .F. ) ;
#8919=CARTESIAN_POINT ( 'NONE',  ( -32.64570716507503079, 53.78543575132162857, 132.4711112102474146 ) ) ;
#8920=CIRCLE ( 'NONE', #4020, 17.50000000000001066 ) ;
#8922=LINE ( 'NONE', #19770, #1163 ) ;
#8923=CARTESIAN_POINT ( 'NONE',  ( 0.000000000000000000, 0.000000000000000000, 283.5832628385307999 ) ) ;
#8924=ORIENTED_EDGE ( 'NONE', *, *, #13759, .F. ) ;
#8931=LINE ( 'NONE', #957, #12909 ) ;
#8933=DIRECTION ( 'NONE',  ( -0.000000000000000000, -0.000000000000000000, 1.000000000000000000 ) ) ;
#8934=AXIS2_PLACEMENT_3D ( 'NONE', #5511, #11733, #3965 ) ;
#8935=ORIENTED_EDGE ( 'NONE', *, *, #498, .F. ) ;
#8936=VERTEX_POINT ( 'NONE', #20153 ) ;
#8937=EDGE_LOOP ( 'NONE', ( #7377, #4508, #14235, #13959 ) ) ;
#8941=AXIS2_PLACEMENT_3D ( 'NONE', #5269, #5460, #14467 ) ;
#8942=CARTESIAN_POINT ( 'NONE',  ( 0.2993243175132189737, -5.729042578294415655, 283.5832628385307999 ) ) ;
#8943=ORIENTED_EDGE ( 'NONE', *, *, #631, .T. ) ;
#8944=FACE_OUTER_BOUND ( 'NONE', #16537, .T. ) ;
#8947=CARTESIAN_POINT ( 'NONE',  ( 73.25972925305629246, -27.53920554013664912, 132.4711112102474146 ) ) ;
#8948=FACE_OUTER_BOUND ( 'NONE', #13774, .T. ) ;
#8952=CIRCLE ( 'NONE', #1452, 62.91752772691707207 ) ;
#8954=ORIENTED_EDGE ( 'NONE', *, *, #10331, .F. ) ;
#8957=ORIENTED_EDGE ( 'NONE', *, *, #14652, .T. ) ;
#8963=DIRECTION ( 'NONE',  ( 0.000000000000000000, 0.000000000000000000, -1.000000000000000000 ) ) ;
#8964=DIRECTION ( 'NONE',  ( -0.3420201433256757073, 0.9396926207859057634, -0.000000000000000000 ) ) ;
#8967=AXIS2_PLACEMENT_3D ( 'NONE', #11126, #12764, #1718 ) ;
#8971=EDGE_CURVE ( 'NONE', #2011, #18719, #4417, .T. ) ;
#8973=LINE ( 'NONE', #18499, #19561 ) ;
#8974=EDGE_CURVE ( 'NONE', #4841, #10024, #1541, .T. ) ;
#8975=ADVANCED_FACE ( 'NONE', ( #3079 ), #3181, .F. ) ;
#8976=CARTESIAN_POINT ( 'NONE',  ( -53.40063514825077107, -28.94886449118923011, 283.5832628385307999 ) ) ;
#8978=CARTESIAN_POINT ( 'NONE',  ( -40.27908801169994035, -45.46712722958821473, 293.5832628385307999 ) ) ;
#8981=CARTESIAN_POINT ( 'NONE',  ( 0.000000000000000000, 0.000000000000000000, 132.4711112102474146 ) ) ;
#8982=ORIENTED_EDGE ( 'NONE', *, *, #2283, .F. ) ;
#8985=VERTEX_POINT ( 'NONE', #12469 ) ;
#8986=ORIENTED_EDGE ( 'NONE', *, *, #16984, .T. ) ;
#8987=ADVANCED_FACE ( 'NONE', ( #14115 ), #12783, .F. ) ;
#8994=AXIS2_PLACEMENT_3D ( 'NONE', #13491, #10326, #1022 ) ;
#8995=CARTESIAN_POINT ( 'NONE',  ( -4.196299268919065462, -3.911853314815649796, 283.5832628385307999 ) ) ;
#8998=EDGE_CURVE ( 'NONE', #9304, #10138, #14855, .T. ) ;
#9000=DIRECTION ( 'NONE',  ( 1.000000000000000000, 0.000000000000000000, 0.000000000000000000 ) ) ;
#9001=EDGE_CURVE ( 'NONE', #13542, #2315, #18943, .T. ) ;
#9003=FACE_OUTER_BOUND ( 'NONE', #7660, .T. ) ;
#9005=CARTESIAN_POINT ( 'NONE',  ( 37.78325588002174840, -47.56406379474564972, 283.5832628385307999 ) ) ;
#9009=ORIENTED_EDGE ( 'NONE', *, *, #17156, .T. ) ;
#9012=EDGE_CURVE ( 'NONE', #2414, #12970, #16068, .T. ) ;
#9013=ORIENTED_EDGE ( 'NONE', *, *, #18489, .T. ) ;
#9016=CARTESIAN_POINT ( 'NONE',  ( -14.39940464655760799, -76.92888220842480962, 248.9926560891072143 ) ) ;
#9017=CARTESIAN_POINT ( 'NONE',  ( -3.453261854572979406, -4.581103194069958917, 283.5832628385307999 ) ) ;
#9020=VECTOR ( 'NONE', #5193, 999.9999999999998863 ) ;
#9021=PLANE ( 'NONE',  #1117 ) ;
#9022=LINE ( 'NONE', #10656, #10718 ) ;
#9023=EDGE_CURVE ( 'NONE', #13898, #10316, #10611, .T. ) ;
#9026=EDGE_LOOP ( 'NONE', ( #5940, #13745, #14090 ) ) ;
#9031=CARTESIAN_POINT ( 'NONE',  ( 51.51682027493064453, -28.15057869795607459, 132.4711112102474146 ) ) ;
#9032=CARTESIAN_POINT ( 'NONE',  ( -12.14957802882752524, -59.51724408343569905, 293.5832628385307999 ) ) ;
#9035=ORIENTED_EDGE ( 'NONE', *, *, #7995, .F. ) ;
#9037=ADVANCED_FACE ( 'NONE', ( #19135 ), #6947, .T. ) ;
#9038=CIRCLE ( 'NONE', #15759, 79.75827554147308263 ) ;
#9039=EDGE_LOOP ( 'NONE', ( #4003, #15197, #12936 ) ) ;
#9043=CARTESIAN_POINT ( 'NONE',  ( 74.01264520835151473, -25.47058595421579597, 111.4180192758974499 ) ) ;
#9045=ORIENTED_EDGE ( 'NONE', *, *, #17980, .F. ) ;
#9047=CARTESIAN_POINT ( 'NONE',  ( -30.05702882063063086, -50.41613078340792242, 132.4711112102474146 ) ) ;
#9048=ORIENTED_EDGE ( 'NONE', *, *, #12722, .T. ) ;
#9050=DIRECTION ( 'NONE',  ( -0.1736481776669340504, 0.9848077530122074652, 0.000000000000000000 ) ) ;
#9056=CIRCLE ( 'NONE', #249, 62.91752772691707207 ) ;
#9066=ORIENTED_EDGE ( 'NONE', *, *, #11425, .F. ) ;
#9067=AXIS2_PLACEMENT_3D ( 'NONE', #4144, #5687, #10370 ) ;
#9068=DIRECTION ( 'NONE',  ( 0.000000000000000000, 0.000000000000000000, 1.000000000000000000 ) ) ;
#9070=VECTOR ( 'NONE', #10641, 1000.000000000000227 ) ;
#9072=DIRECTION ( 'NONE',  ( 1.000000000000000000, 0.000000000000000000, 0.000000000000000000 ) ) ;
#9073=ORIENTED_EDGE ( 'NONE', *, *, #3534, .F. ) ;
#9081=VECTOR ( 'NONE', #13904, 1000.000000000000000 ) ;
#9089=CARTESIAN_POINT ( 'NONE',  ( -12.23146955673647618, -77.31114765718484705, 132.4711112102474146 ) ) ;
#9100=CIRCLE ( 'NONE', #11077, 79.75827554147308263 ) ;
#9103=CARTESIAN_POINT ( 'NONE',  ( -54.86954475316242252, 20.84572577951219330, 132.4711112102474146 ) ) ;
#9104=DIRECTION ( 'NONE',  ( -0.3420201433256601642, -0.9396926207859114255, 0.000000000000000000 ) ) ;
#9111=CARTESIAN_POINT ( 'NONE',  ( 59.30917539369505675, -13.12769224524051559, 293.5832628385307999 ) ) ;
#9112=CARTESIAN_POINT ( 'NONE',  ( 12.78021302872850562, -77.21438937758507848, 132.4711112102474146 ) ) ;
#9113=EDGE_LOOP ( 'NONE', ( #11417, #5922, #14744, #10485 ) ) ;
#9118=EDGE_CURVE ( 'NONE', #11697, #11236, #11601, .T. ) ;
#9120=ADVANCED_FACE ( 'NONE', ( #19333 ), #11351, .T. ) ;
#9121=FACE_BOUND ( 'NONE', #4135, .T. ) ;
#9125=LINE ( 'NONE', #2690, #8734 ) ;
#9126=CARTESIAN_POINT ( 'NONE',  ( -53.78543575132151489, -32.64570716507521553, 132.4711112102474146 ) ) ;
#9131=ORIENTED_EDGE ( 'NONE', *, *, #61, .T. ) ;
#9132=CARTESIAN_POINT ( 'NONE',  ( 9.381844291199747943, -57.94128254008187184, 112.0427633081291816 ) ) ;
#9134=EDGE_CURVE ( 'NONE', #5555, #9722, #704, .T. ) ;
#9137=CARTESIAN_POINT ( 'NONE',  ( 0.000000000000000000, 0.000000000000000000, 283.5832628385307999 ) ) ;
#9140=DIRECTION ( 'NONE',  ( -0.000000000000000000, -0.000000000000000000, 1.000000000000000000 ) ) ;
#9142=ORIENTED_EDGE ( 'NONE', *, *, #9643, .F. ) ;
#9147=ORIENTED_EDGE ( 'NONE', *, *, #4775, .F. ) ;
#9148=EDGE_LOOP ( 'NONE', ( #11780, #15203, #8368, #7502 ) ) ;
#9150=DIRECTION ( 'NONE',  ( 0.6427876096865458022, -0.7660444431189726844, 0.000000000000000000 ) ) ;
#9153=ADVANCED_FACE ( 'NONE', ( #8675 ), #898, .T. ) ;
#9156=VERTEX_POINT ( 'NONE', #5815 ) ;
#9158=EDGE_CURVE ( 'NONE', #2090, #5714, #7244, .T. ) ;
#9159=CARTESIAN_POINT ( 'NONE',  ( 20.84572577951164618, 54.86954475316263569, 248.9926560891072143 ) ) ;
#9161=CARTESIAN_POINT ( 'NONE',  ( 32.61983739937763005, 51.24071425735591845, 283.5832628385307999 ) ) ;
#9163=DIRECTION ( 'NONE',  ( 0.3420201433256630508, 0.9396926207859104263, 0.000000000000000000 ) ) ;
#9165=FACE_OUTER_BOUND ( 'NONE', #5071, .T. ) ;
#9166=ORIENTED_EDGE ( 'NONE', *, *, #14113, .F. ) ;
#9168=DIRECTION ( 'NONE',  ( 1.000000000000000000, 0.000000000000000000, 0.000000000000000000 ) ) ;
#9169=ORIENTED_EDGE ( 'NONE', *, *, #11535, .F. ) ;
#9170=ORIENTED_EDGE ( 'NONE', *, *, #4754, .T. ) ;
#9171=DIRECTION ( 'NONE',  ( -0.000000000000000000, -0.000000000000000000, 1.000000000000000000 ) ) ;
#9172=VERTEX_POINT ( 'NONE', #4272 ) ;
#9175=EDGE_CURVE ( 'NONE', #9484, #15959, #18190, .T. ) ;
#9178=CARTESIAN_POINT ( 'NONE',  ( 0.000000000000000000, 0.000000000000000000, 132.4711112102474146 ) ) ;
#9185=CARTESIAN_POINT ( 'NONE',  ( 5.693982670708947147, -0.7000608949449556029, 293.5832628385307999 ) ) ;
#9190=VECTOR ( 'NONE', #3808, 1000.000000000000114 ) ;
#9192=ORIENTED_EDGE ( 'NONE', *, *, #16479, .T. ) ;
#9194=DIRECTION ( 'NONE',  ( 0.9848077530122073542, 0.1736481776669340227, 0.000000000000000000 ) ) ;
#9195=VERTEX_POINT ( 'NONE', #10401 ) ;
#9198=EDGE_LOOP ( 'NONE', ( #10649, #3894, #18779 ) ) ;
#9201=FACE_OUTER_BOUND ( 'NONE', #9560, .T. ) ;
#9202=ORIENTED_EDGE ( 'NONE', *, *, #6252, .T. ) ;
#9204=CARTESIAN_POINT ( 'NONE',  ( -53.40063514825077107, -28.94886449118923011, 283.5832628385307999 ) ) ;
#9209=EDGE_CURVE ( 'NONE', #4654, #6858, #5081, .T. ) ;
#9214=EDGE_LOOP ( 'NONE', ( #17946, #12312, #2180, #17045 ) ) ;
#9220=VECTOR ( 'NONE', #15489, 1000.000000000000000 ) ;
#9221=AXIS2_PLACEMENT_3D ( 'NONE', #6158, #1958, #3186 ) ;
#9225=EDGE_CURVE ( 'NONE', #2759, #1374, #5723, .T. ) ;
#9227=VERTEX_POINT ( 'NONE', #12033 ) ;
#9228=VECTOR ( 'NONE', #16077, 1000.000000000000000 ) ;
#9229=DIRECTION ( 'NONE',  ( -0.8830229359480288309, -0.4693298356057531984, 0.000000000000000000 ) ) ;
#9232=LINE ( 'NONE', #4930, #8537 ) ;
#9236=DIRECTION ( 'NONE',  ( 0.000000000000000000, 0.000000000000000000, 1.000000000000000000 ) ) ;
#9238=EDGE_CURVE ( 'NONE', #4139, #13695, #19620, .T. ) ;
#9241=AXIS2_PLACEMENT_3D ( 'NONE', #16235, #17972, #867 ) ;
#9245=ORIENTED_EDGE ( 'NONE', *, *, #2365, .F. ) ;
#9247=CARTESIAN_POINT ( 'NONE',  ( 58.63718168490485283, 22.81000261549389307, 132.4711112102474146 ) ) ;
#9248=AXIS2_PLACEMENT_3D ( 'NONE', #15102, #1082, #7330 ) ;
#9249=CIRCLE ( 'NONE', #12511, 60.74260934110282051 ) ;
#9251=ORIENTED_EDGE ( 'NONE', *, *, #9724, .T. ) ;
#9257=FACE_OUTER_BOUND ( 'NONE', #19991, .T. ) ;
#9258=LINE ( 'NONE', #18464, #2875 ) ;
#9261=CARTESIAN_POINT ( 'NONE',  ( 41.02212542604613077, 44.79787735033405482, 293.5832628385307999 ) ) ;
#9262=ORIENTED_EDGE ( 'NONE', *, *, #764, .T. ) ;
#9263=DIRECTION ( 'NONE',  ( 1.000000000000000000, 0.000000000000000000, 0.000000000000000000 ) ) ;
#9264=LINE ( 'NONE', #18689, #17875 ) ;
#9265=CARTESIAN_POINT ( 'NONE',  ( 48.17959877923549072, 36.99514631729036296, 293.5832628385307999 ) ) ;
#9267=EDGE_CURVE ( 'NONE', #17702, #8089, #15211, .T. ) ;
#9268=DIRECTION ( 'NONE',  ( -0.9993852124581887875, 0.03505990758545545621, 0.000000000000000000 ) ) ;
#9269=CARTESIAN_POINT ( 'NONE',  ( -31.77296517111735596, -51.77251465595229263, 293.5832628385307999 ) ) ;
#9272=LINE ( 'NONE', #20108, #216 ) ;
#9274=VERTEX_POINT ( 'NONE', #19922 ) ;
#9275=VERTEX_POINT ( 'NONE', #18398 ) ;
#9276=AXIS2_PLACEMENT_3D ( 'NONE', #11068, #11171, #17436 ) ;
#9278=LINE ( 'NONE', #4893, #16456 ) ;
#9280=AXIS2_PLACEMENT_3D ( 'NONE', #16462, #2442, #8673 ) ;
#9281=ORIENTED_EDGE ( 'NONE', *, *, #2241, .F. ) ;
#9282=DIRECTION ( 'NONE',  ( -0.1736481776669306920, 0.9848077530122080203, 0.000000000000000000 ) ) ;
#9284=DIRECTION ( 'NONE',  ( 1.000000000000000000, 0.000000000000000000, 0.000000000000000000 ) ) ;
#9288=CARTESIAN_POINT ( 'NONE',  ( 78.26059000578310076, 1.379293853802574077, 132.4711112102474146 ) ) ;
#9291=DIRECTION ( 'NONE',  ( 0.7660444431189749048, 0.6427876096865430267, -0.000000000000000000 ) ) ;
#9292=DIRECTION ( 'NONE',  ( -0.000000000000000000, -0.000000000000000000, 1.000000000000000000 ) ) ;
#9293=ADVANCED_FACE ( 'NONE', ( #8773 ), #15016, .F. ) ;
#9294=AXIS2_PLACEMENT_3D ( 'NONE', #14119, #12473, #18429 ) ;
#9295=PLANE ( 'NONE',  #3440 ) ;
#9298=CARTESIAN_POINT ( 'NONE',  ( 59.30917539369505675, -13.12769224524051559, 283.5832628385307999 ) ) ;
#9300=EDGE_CURVE ( 'NONE', #11632, #3495, #15323, .T. ) ;
#9304=VERTEX_POINT ( 'NONE', #15532 ) ;
#9305=CARTESIAN_POINT ( 'NONE',  ( 28.63313560863472063, -51.23821591265105013, 110.9660488491356887 ) ) ;
#9307=ORIENTED_EDGE ( 'NONE', *, *, #20115, .F. ) ;
#9310=EDGE_LOOP ( 'NONE', ( #2318, #1723, #1662, #5574 ) ) ;
#9312=DIRECTION ( 'NONE',  ( -0.000000000000000000, -0.000000000000000000, 1.000000000000000000 ) ) ;
#9314=DIRECTION ( 'NONE',  ( 0.7660444431189707970, 0.6427876096865481337, 0.000000000000000000 ) ) ;
#9316=ORIENTED_EDGE ( 'NONE', *, *, #17991, .T. ) ;
#9317=CARTESIAN_POINT ( 'NONE',  ( 60.83768308848376449, -49.24833719034207036, 248.9926560891072143 ) ) ;
#9320=LINE ( 'NONE', #15563, #11822 ) ;
#9323=DIRECTION ( 'NONE',  ( 1.000000000000000000, 0.000000000000000000, 0.000000000000000000 ) ) ;
#9325=VERTEX_POINT ( 'NONE', #15425 ) ;
#9331=FACE_BOUND ( 'NONE', #10472, .T. ) ;
#9333=CARTESIAN_POINT ( 'NONE',  ( 37.78325588002174840, -47.56406379474564972, 283.5832628385307999 ) ) ;
#9334=LINE ( 'NONE', #3204, #19088 ) ;
#9335=CARTESIAN_POINT ( 'NONE',  ( 28.06584155524102187, -53.86996498385662591, 283.5832628385307999 ) ) ;
#9338=DIRECTION ( 'NONE',  ( -0.000000000000000000, -0.000000000000000000, 1.000000000000000000 ) ) ;
#9339=VECTOR ( 'NONE', #19793, 1000.000000000000114 ) ;
#9340=LINE ( 'NONE', #4322, #3292 ) ;
#9341=PLANE ( 'NONE',  #12587 ) ;
#9344=CARTESIAN_POINT ( 'NONE',  ( -23.22641211976288389, -56.12662799072081299, 293.5832628385307999 ) ) ;
#9348=AXIS2_PLACEMENT_3D ( 'NONE', #7643, #6024, #20123 ) ;
#9349=LINE ( 'NONE', #10875, #9220 ) ;
#9350=EDGE_LOOP ( 'NONE', ( #10799, #8419 ) ) ;
#9351=VERTEX_POINT ( 'NONE', #20124 ) ;
#9353=EDGE_CURVE ( 'NONE', #17450, #13065, #16963, .T. ) ;
#9357=EDGE_CURVE ( 'NONE', #9351, #8683, #20025, .T. ) ;
#9358=CIRCLE ( 'NONE', #553, 62.91752772691707207 ) ;
#9360=PLANE ( 'NONE',  #12334 ) ;
#9366=DIRECTION ( 'NONE',  ( 0.3747554100459959958, 0.9271237148521535021, 0.000000000000000000 ) ) ;
#9369=EDGE_CURVE ( 'NONE', #1970, #5595, #1714, .T. ) ;
#9370=ORIENTED_EDGE ( 'NONE', *, *, #12775, .F. ) ;
#9371=VECTOR ( 'NONE', #7265, 1000.000000000000000 ) ;
#9372=PLANE ( 'NONE',  #264 ) ;
#9374=EDGE_LOOP ( 'NONE', ( #19782, #19965, #5937, #17993 ) ) ;
#9378=VERTEX_POINT ( 'NONE', #12342 ) ;
#9382=CARTESIAN_POINT ( 'NONE',  ( 20.84572577951164618, 54.86954475316263569, 111.4180192758974499 ) ) ;
#9383=EDGE_CURVE ( 'NONE', #1375, #20213, #4475, .T. ) ;
#9384=ADVANCED_FACE ( 'NONE', ( #6025 ), #4693, .T. ) ;
#9388=DIRECTION ( 'NONE',  ( 1.000000000000000000, 0.000000000000000000, 0.000000000000000000 ) ) ;
#9389=VERTEX_POINT ( 'NONE', #13986 ) ;
#9392=ORIENTED_EDGE ( 'NONE', *, *, #12737, .F. ) ;
#9394=PLANE ( 'NONE',  #18260 ) ;
#9395=DIRECTION ( 'NONE',  ( 1.000000000000000000, 0.000000000000000000, 0.000000000000000000 ) ) ;
#9397=DIRECTION ( 'NONE',  ( 0.000000000000000000, 0.000000000000000000, 1.000000000000000000 ) ) ;
#9399=LINE ( 'NONE', #10612, #12494 ) ;
#9401=PLANE ( 'NONE',  #15806 ) ;
#9402=ORIENTED_EDGE ( 'NONE', *, *, #15277, .T. ) ;
#9406=AXIS2_PLACEMENT_3D ( 'NONE', #10536, #20165, #9323 ) ;
#9407=ADVANCED_FACE ( 'NONE', ( #1413 ), #17278, .T. ) ;
#9408=ORIENTED_EDGE ( 'NONE', *, *, #17186, .F. ) ;
#9410=CARTESIAN_POINT ( 'NONE',  ( 17.50000000000001066, 0.000000000000000000, 83.57543755549745867 ) ) ;
#9411=DIRECTION ( 'NONE',  ( 0.000000000000000000, 0.000000000000000000, 1.000000000000000000 ) ) ;
#9412=ORIENTED_EDGE ( 'NONE', *, *, #16389, .T. ) ;
#9414=DIRECTION ( 'NONE',  ( -0.000000000000000000, -0.000000000000000000, 1.000000000000000000 ) ) ;
#9422=VERTEX_POINT ( 'NONE', #9288 ) ;
#9424=CARTESIAN_POINT ( 'NONE',  ( -1.678175111358135130, -5.485913980968154746, 293.5832628385307999 ) ) ;
#9427=ORIENTED_EDGE ( 'NONE', *, *, #19467, .T. ) ;
#9429=CARTESIAN_POINT ( 'NONE',  ( -32.64570716507503079, 53.78543575132162857, 293.5832628385307999 ) ) ;
#9430=EDGE_LOOP ( 'NONE', ( #7738, #697, #15597 ) ) ;
#9432=VERTEX_POINT ( 'NONE', #181 ) ;
#9434=VECTOR ( 'NONE', #13364, 1000.000000000000114 ) ;
#9437=VECTOR ( 'NONE', #13989, 1000.000000000000000 ) ;
#9439=CIRCLE ( 'NONE', #1939, 60.74260934110282051 ) ;
#9440=CARTESIAN_POINT ( 'NONE',  ( -13.12726406102078158, -59.30716253403180360, 283.5832628385307999 ) ) ;
#9441=ORIENTED_EDGE ( 'NONE', *, *, #11091, .T. ) ;
#9444=EDGE_CURVE ( 'NONE', #19147, #6858, #79, .T. ) ;
#9449=LINE ( 'NONE', #1776, #17059 ) ;
#9450=VECTOR ( 'NONE', #10635, 1000.000000000000000 ) ;
#9451=DIRECTION ( 'NONE',  ( -0.6427876096865300370, -0.7660444431189858960, 0.000000000000000000 ) ) ;
#9452=LINE ( 'NONE', #8313, #2013 ) ;
#9453=CIRCLE ( 'NONE', #938, 62.91752772691707207 ) ;
#9455=AXIS2_PLACEMENT_3D ( 'NONE', #971, #15189, #13439 ) ;
#9457=AXIS2_PLACEMENT_3D ( 'NONE', #13419, #11691, #7101 ) ;
#9458=DIRECTION ( 'NONE',  ( 1.000000000000000000, 0.000000000000000000, -0.000000000000000000 ) ) ;
#9461=ORIENTED_EDGE ( 'NONE', *, *, #8885, .F. ) ;
#9464=EDGE_CURVE ( 'NONE', #7122, #13906, #7848, .T. ) ;
#9465=DIRECTION ( 'NONE',  ( -0.8660254037844415942, 0.4999999999999949485, 0.000000000000000000 ) ) ;
#9466=DIRECTION ( 'NONE',  ( 1.000000000000000000, 0.000000000000000000, 0.000000000000000000 ) ) ;
#9467=CARTESIAN_POINT ( 'NONE',  ( 1.629865514042525776, 60.72073886220395877, 293.5832628385307999 ) ) ;
#9468=VERTEX_POINT ( 'NONE', #15938 ) ;
#9470=CARTESIAN_POINT ( 'NONE',  ( 1.629865514042525554, 60.72073886220396588, 283.5832628385307999 ) ) ;
#9472=LINE ( 'NONE', #3232, #4598 ) ;
#9478=ORIENTED_EDGE ( 'NONE', *, *, #19156, .T. ) ;
#9481=ORIENTED_EDGE ( 'NONE', *, *, #2790, .F. ) ;
#9482=DIRECTION ( 'NONE',  ( -0.000000000000000000, -0.000000000000000000, 1.000000000000000000 ) ) ;
#9484=VERTEX_POINT ( 'NONE', #11219 ) ;
#9485=LINE ( 'NONE', #8044, #2187 ) ;
#9486=ADVANCED_FACE ( 'NONE', ( #2326 ), #9790, .F. ) ;
#9489=AXIS2_PLACEMENT_3D ( 'NONE', #10716, #6034, #1006 ) ;
#9490=CARTESIAN_POINT ( 'NONE',  ( 57.92514141135451666, 18.28503710798567994, 283.5832628385307999 ) ) ;
#9499=CARTESIAN_POINT ( 'NONE',  ( 18.28567271940513450, -57.92709869106715814, 293.5832628385307999 ) ) ;
#9501=EDGE_CURVE ( 'NONE', #18959, #4038, #13145, .T. ) ;
#9502=CARTESIAN_POINT ( 'NONE',  ( 0.000000000000000000, 0.000000000000000000, 248.9926560891072143 ) ) ;
#9507=DIRECTION ( 'NONE',  ( 1.000000000000000000, 0.000000000000000000, 0.000000000000000000 ) ) ;
#9508=VERTEX_POINT ( 'NONE', #19018 ) ;
#9511=DIRECTION ( 'NONE',  ( -0.9271237148521536131, 0.3747554100459959958, 0.000000000000000000 ) ) ;
#9512=ORIENTED_EDGE ( 'NONE', *, *, #9267, .T. ) ;
#9515=LINE ( 'NONE', #12974, #5348 ) ;
#9516=EDGE_LOOP ( 'NONE', ( #18737, #15826, #2236 ) ) ;
#9518=DIRECTION ( 'NONE',  ( 1.000000000000000000, 0.000000000000000000, 0.000000000000000000 ) ) ;
#9519=VECTOR ( 'NONE', #512, 1000.000000000000000 ) ;
#9521=DIRECTION ( 'NONE',  ( -0.5300553768524346454, -0.8479630283625717579, 0.000000000000000000 ) ) ;
#9523=EDGE_LOOP ( 'NONE', ( #14711, #6250, #10318, #8442 ) ) ;
#9524=CYLINDRICAL_SURFACE ( 'NONE', #19677, 60.74260934110282051 ) ;
#9525=DIRECTION ( 'NONE',  ( 1.000000000000000000, 0.000000000000000000, -0.000000000000000000 ) ) ;
#9526=EDGE_CURVE ( 'NONE', #12122, #18228, #18592, .T. ) ;
#9530=EDGE_CURVE ( 'NONE', #10395, #8936, #5393, .T. ) ;
#9534=VERTEX_POINT ( 'NONE', #6928 ) ;
#9535=EDGE_LOOP ( 'NONE', ( #3277, #6142, #4079, #5168 ) ) ;
#9538=VERTEX_POINT ( 'NONE', #19409 ) ;
#9542=ORIENTED_EDGE ( 'NONE', *, *, #18534, .T. ) ;
#9543=CARTESIAN_POINT ( 'NONE',  ( -77.31114765718484705, 12.23146955673673197, 112.0427633081292385 ) ) ;
#9552=DIRECTION ( 'NONE',  ( 0.9848077530122080203, 0.1736481776669306920, 0.000000000000000000 ) ) ;
#9553=FACE_OUTER_BOUND ( 'NONE', #9703, .T. ) ;
#9555=ORIENTED_EDGE ( 'NONE', *, *, #14758, .T. ) ;
#9559=EDGE_CURVE ( 'NONE', #6626, #18719, #581, .T. ) ;
#9560=EDGE_LOOP ( 'NONE', ( #12202, #12543, #17670 ) ) ;
#9561=CIRCLE ( 'NONE', #12153, 62.91752772691707207 ) ;
#9563=ORIENTED_EDGE ( 'NONE', *, *, #360, .T. ) ;
#9565=CARTESIAN_POINT ( 'NONE',  ( 0.8220851292435327196, 78.26059000578311498, 112.7772637782949943 ) ) ;
#9567=AXIS2_PLACEMENT_3D ( 'NONE', #15971, #11151, #6360 ) ;
#9569=CARTESIAN_POINT ( 'NONE',  ( 54.89456854707540856, 30.74413178637211885, 293.5832628385307999 ) ) ;
#9574=CYLINDRICAL_SURFACE ( 'NONE', #10054, 60.74260934110282051 ) ;
#9575=VERTEX_POINT ( 'NONE', #14401 ) ;
#9578=VERTEX_POINT ( 'NONE', #382 ) ;
#9579=CIRCLE ( 'NONE', #3361, 60.74260934110282051 ) ;
#9581=ORIENTED_EDGE ( 'NONE', *, *, #7286, .T. ) ;
#9583=LINE ( 'NONE', #3248, #11540 ) ;
#9584=ORIENTED_EDGE ( 'NONE', *, *, #19859, .T. ) ;
#9585=DIRECTION ( 'NONE',  ( 0.9848077530122080203, 0.1736481776669306920, 0.000000000000000000 ) ) ;
#9586=VECTOR ( 'NONE', #13256, 1000.000000000000114 ) ;
#9590=ORIENTED_EDGE ( 'NONE', *, *, #18361, .T. ) ;
#9594=DIRECTION ( 'NONE',  ( 0.6427876096865353661, 0.7660444431189813441, 0.000000000000000000 ) ) ;
#9595=CARTESIAN_POINT ( 'NONE',  ( 30.53958573130908505, -50.13752642112839197, 110.9660488491356887 ) ) ;
#9596=CIRCLE ( 'NONE', #5663, 60.74260934110282051 ) ;
#9597=DIRECTION ( 'NONE',  ( -0.000000000000000000, -0.000000000000000000, 1.000000000000000000 ) ) ;
#9600=VECTOR ( 'NONE', #13746, 1000.000000000000000 ) ;
#9602=VERTEX_POINT ( 'NONE', #684 ) ;
#9603=EDGE_CURVE ( 'NONE', #8683, #6975, #16339, .T. ) ;
#9604=DIRECTION ( 'NONE',  ( 1.000000000000000000, 0.000000000000000000, 0.000000000000000000 ) ) ;
#9605=ORIENTED_EDGE ( 'NONE', *, *, #14143, .F. ) ;
#9606=ORIENTED_EDGE ( 'NONE', *, *, #3460, .F. ) ;
#9607=CARTESIAN_POINT ( 'NONE',  ( 25.99419088092191643, -73.82206860051540787, 132.4711112102474146 ) ) ;
#9608=ORIENTED_EDGE ( 'NONE', *, *, #174, .T. ) ;
#9611=LINE ( 'NONE', #18940, #4366 ) ;
#9613=EDGE_CURVE ( 'NONE', #5657, #2071, #14500, .T. ) ;
#9615=DIRECTION ( 'NONE',  ( 0.9396926207859114255, -0.3420201433256601642, 0.000000000000000000 ) ) ;
#9616=EDGE_CURVE ( 'NONE', #6558, #11573, #18262, .T. ) ;
#9618=AXIS2_PLACEMENT_3D ( 'NONE', #18883, #3221, #12623 ) ;
#9620=CARTESIAN_POINT ( 'NONE',  ( 14.94814811854963388, -76.83212392882496999, 248.9926560891072143 ) ) ;
#9622=CARTESIAN_POINT ( 'NONE',  ( 0.000000000000000000, 0.000000000000000000, 293.5832628385307999 ) ) ;
#9623=CARTESIAN_POINT ( 'NONE',  ( -79.75827554147308263, 9.767571684737763671E-15, 248.9926560891072143 ) ) ;
#9624=DIRECTION ( 'NONE',  ( 0.9993852124581887875, -0.03505990758545544927, 0.000000000000000000 ) ) ;
#9626=EDGE_LOOP ( 'NONE', ( #7457, #5430, #15077, #3240 ) ) ;
#9627=EDGE_CURVE ( 'NONE', #17740, #4738, #11327, .T. ) ;
#9628=DIRECTION ( 'NONE',  ( -0.6155349844899689060, 0.7881095627315620744, 0.000000000000000000 ) ) ;
#9630=ORIENTED_EDGE ( 'NONE', *, *, #14641, .F. ) ;
#9635=ORIENTED_EDGE ( 'NONE', *, *, #11168, .F. ) ;
#9640=AXIS2_PLACEMENT_3D ( 'NONE', #8870, #10601, #7340 ) ;
#9643=EDGE_CURVE ( 'NONE', #8342, #7122, #6526, .T. ) ;
#9647=FACE_OUTER_BOUND ( 'NONE', #864, .T. ) ;
#9651=EDGE_CURVE ( 'NONE', #10444, #937, #6193, .T. ) ;
#9653=DIRECTION ( 'NONE',  ( -0.000000000000000000, -0.000000000000000000, 1.000000000000000000 ) ) ;
#9656=EDGE_LOOP ( 'NONE', ( #4442, #7763, #16062, #19098 ) ) ;
#9659=EDGE_CURVE ( 'NONE', #19327, #13999, #10283, .T. ) ;
#9663=CIRCLE ( 'NONE', #12268, 62.91752772691707207 ) ;
#9664=CARTESIAN_POINT ( 'NONE',  ( 1.629865514042525776, 60.72073886220395877, 283.5832628385307999 ) ) ;
#9666=ADVANCED_FACE ( 'NONE', ( #7415 ), #16442, .F. ) ;
#9669=DIRECTION ( 'NONE',  ( 1.000000000000000000, 1.047444401652940164E-14, 0.000000000000000000 ) ) ;
#9680=DIRECTION ( 'NONE',  ( -0.000000000000000000, -0.000000000000000000, 1.000000000000000000 ) ) ;
#9681=VECTOR ( 'NONE', #8235, 1000.000000000000000 ) ;
#9683=CARTESIAN_POINT ( 'NONE',  ( -13.12769224524071277, -59.30917539369501412, 293.5832628385307999 ) ) ;
#9685=DIRECTION ( 'NONE',  ( -0.6692498792541777819, -0.7430374143461878633, 0.000000000000000000 ) ) ;
#9686=CARTESIAN_POINT ( 'NONE',  ( 57.94128254008182921, 9.381844291199925578, 112.0427633081291816 ) ) ;
#9688=DIRECTION ( 'NONE',  ( 1.000000000000000000, 0.000000000000000000, 0.000000000000000000 ) ) ;
#9690=VECTOR ( 'NONE', #9291, 1000.000000000000000 ) ;
#9691=VERTEX_POINT ( 'NONE', #8746 ) ;
#9692=DIRECTION ( 'NONE',  ( 1.000000000000000000, 0.000000000000000000, 0.000000000000000000 ) ) ;
#9695=DIRECTION ( 'NONE',  ( -0.000000000000000000, -0.000000000000000000, 1.000000000000000000 ) ) ;
#9697=FACE_OUTER_BOUND ( 'NONE', #16842, .T. ) ;
#9701=PLANE ( 'NONE',  #3061 ) ;
#9702=ORIENTED_EDGE ( 'NONE', *, *, #17917, .T. ) ;
#9703=EDGE_LOOP ( 'NONE', ( #1078, #5691, #18250, #16383 ) ) ;
#9704=CARTESIAN_POINT ( 'NONE',  ( 22.28973221005081484, 58.83691981461641518, 248.9926560891072143 ) ) ;
#9705=VERTEX_POINT ( 'NONE', #19594 ) ;
#9707=VECTOR ( 'NONE', #4178, 1000.000000000000114 ) ;
#9711=EDGE_CURVE ( 'NONE', #6026, #14067, #7480, .T. ) ;
#9714=LINE ( 'NONE', #4931, #13396 ) ;
#9716=ORIENTED_EDGE ( 'NONE', *, *, #764, .F. ) ;
#9718=DIRECTION ( 'NONE',  ( 0.000000000000000000, 0.000000000000000000, 1.000000000000000000 ) ) ;
#9720=DIRECTION ( 'NONE',  ( 0.9848077530122085754, -0.1736481776669273336, 0.000000000000000000 ) ) ;
#9721=AXIS2_PLACEMENT_3D ( 'NONE', #10090, #8349, #16336 ) ;
#9722=VERTEX_POINT ( 'NONE', #17977 ) ;
#9724=EDGE_CURVE ( 'NONE', #18854, #10141, #1609, .T. ) ;
#9727=AXIS2_PLACEMENT_3D ( 'NONE', #2605, #10455, #14968 ) ;
#9729=ORIENTED_EDGE ( 'NONE', *, *, #4787, .F. ) ;
#9731=VERTEX_POINT ( 'NONE', #873 ) ;
#9734=ORIENTED_EDGE ( 'NONE', *, *, #1218, .T. ) ;
#9736=PLANE ( 'NONE',  #12539 ) ;
#9743=DIRECTION ( 'NONE',  ( -0.000000000000000000, -0.000000000000000000, 1.000000000000000000 ) ) ;
#9747=DIRECTION ( 'NONE',  ( -0.000000000000000000, -0.000000000000000000, 1.000000000000000000 ) ) ;
#9750=DIRECTION ( 'NONE',  ( 0.9396926207859068736, 0.3420201433256726542, -0.000000000000000000 ) ) ;
#9752=EDGE_CURVE ( 'NONE', #15281, #6318, #11421, .T. ) ;
#9754=AXIS2_PLACEMENT_3D ( 'NONE', #7546, #18095, #18299 ) ;
#9755=VECTOR ( 'NONE', #526, 1000.000000000000000 ) ;
#9758=VERTEX_POINT ( 'NONE', #18267 ) ;
#9761=CARTESIAN_POINT ( 'NONE',  ( -1.379293853801755176, 62.91752772691707207, 248.9926560891072143 ) ) ;
#9762=CARTESIAN_POINT ( 'NONE',  ( 0.000000000000000000, 0.000000000000000000, 293.5832628385307999 ) ) ;
#9766=EDGE_CURVE ( 'NONE', #19640, #12693, #10475, .T. ) ;
#9768=AXIS2_PLACEMENT_3D ( 'NONE', #18201, #4185, #18072 ) ;
#9770=PLANE ( 'NONE',  #6201 ) ;
#9772=LINE ( 'NONE', #19194, #16910 ) ;
#9773=ORIENTED_EDGE ( 'NONE', *, *, #16163, .F. ) ;
#9774=EDGE_CURVE ( 'NONE', #14265, #5572, #12111, .T. ) ;
#9775=ADVANCED_FACE ( 'NONE', ( #14794 ), #779, .F. ) ;
#9776=CARTESIAN_POINT ( 'NONE',  ( 60.72279549541555355, -1.629937663769388090, 283.5832628385307999 ) ) ;
#9777=ORIENTED_EDGE ( 'NONE', *, *, #12340, .T. ) ;
#9779=EDGE_LOOP ( 'NONE', ( #11617, #9773, #5264, #16326 ) ) ;
#9780=ORIENTED_EDGE ( 'NONE', *, *, #4212, .T. ) ;
#9782=ORIENTED_EDGE ( 'NONE', *, *, #1273, .F. ) ;
#9783=ORIENTED_EDGE ( 'NONE', *, *, #7240, .F. ) ;
#9786=CARTESIAN_POINT ( 'NONE',  ( 0.2993243175132176415, -5.729042578294388122, 293.5832628385307999 ) ) ;
#9790=PLANE ( 'NONE',  #14364 ) ;
#9796=CARTESIAN_POINT ( 'NONE',  ( -5.729042578294540888, -0.2993243175132380696, 293.5832628385307999 ) ) ;
#9797=EDGE_CURVE ( 'NONE', #14568, #15800, #7822, .T. ) ;
#9802=EDGE_LOOP ( 'NONE', ( #8917, #2045, #15625, #13819 ) ) ;
#9804=VERTEX_POINT ( 'NONE', #6307 ) ;
#9805=ADVANCED_FACE ( 'NONE', ( #18575 ), #1285, .T. ) ;
#9806=ORIENTED_EDGE ( 'NONE', *, *, #14317, .F. ) ;
#9808=VERTEX_POINT ( 'NONE', #10788 ) ;
#9810=LINE ( 'NONE', #19233, #16982 ) ;
#9813=FILL_AREA_STYLE ('',( #14325 ) ) ;
#9819=DIRECTION ( 'NONE',  ( 0.9271237148521548344, -0.3747554100459928317, 0.000000000000000000 ) ) ;
#9820=CARTESIAN_POINT ( 'NONE',  ( 78.26059000578312919, -0.8220851292427129309, 112.7772637782949516 ) ) ;
#9822=DIRECTION ( 'NONE',  ( 1.000000000000000000, 0.000000000000000000, 0.000000000000000000 ) ) ;
#9825=ORIENTED_EDGE ( 'NONE', *, *, #19887, .T. ) ;
#9826=CARTESIAN_POINT ( 'NONE',  ( 20.69304990905149211, 6.063840362151302621, 248.9926560891072143 ) ) ;
#9832=EDGE_LOOP ( 'NONE', ( #18179, #4866, #9911 ) ) ;
#9833=VECTOR ( 'NONE', #19507, 1000.000000000000114 ) ;
#9834=DIRECTION ( 'NONE',  ( -0.3420201433256725987, 0.9396926207859068736, 0.000000000000000000 ) ) ;
#9835=ORIENTED_EDGE ( 'NONE', *, *, #18888, .T. ) ;
#9836=AXIS2_PLACEMENT_3D ( 'NONE', #18558, #10771, #19979 ) ;
#9840=ORIENTED_EDGE ( 'NONE', *, *, #1482, .F. ) ;
#9841=EDGE_CURVE ( 'NONE', #3178, #15284, #8796, .T. ) ;
#9843=AXIS2_PLACEMENT_3D ( 'NONE', #18871, #11285, #338 ) ;
#9845=CARTESIAN_POINT ( 'NONE',  ( 60.83768308848375739, -49.24833719034207036, 132.4711112102474146 ) ) ;
#9848=ORIENTED_EDGE ( 'NONE', *, *, #5556, .F. ) ;
#9852=EDGE_CURVE ( 'NONE', #1374, #2759, #7175, .T. ) ;
#9855=ORIENTED_EDGE ( 'NONE', *, *, #6042, .T. ) ;
#9856=ORIENTED_EDGE ( 'NONE', *, *, #12411, .F. ) ;
#9857=DIRECTION ( 'NONE',  ( -0.5060387318153625191, 0.000000000000000000, -0.8625107546591518348 ) ) ;
#9858=CARTESIAN_POINT ( 'NONE',  ( 0.000000000000000000, 0.000000000000000000, 283.5832628385307999 ) ) ;
#9859=ADVANCED_FACE ( 'NONE', ( #5998 ), #15504, .T. ) ;
#9860=DIRECTION ( 'NONE',  ( -0.6427876096865430267, 0.7660444431189749048, 0.000000000000000000 ) ) ;
#9863=EDGE_CURVE ( 'NONE', #5705, #17978, #12217, .T. ) ;
#9864=DIRECTION ( 'NONE',  ( 0.000000000000000000, 0.000000000000000000, -1.000000000000000000 ) ) ;
#9871=PLANE ( 'NONE',  #8379 ) ;
#9872=VERTEX_POINT ( 'NONE', #9261 ) ;
#9874=ORIENTED_EDGE ( 'NONE', *, *, #17847, .F. ) ;
#9875=EDGE_CURVE ( 'NONE', #4545, #5829, #4665, .T. ) ;
#9876=ORIENTED_EDGE ( 'NONE', *, *, #15198, .F. ) ;
#9877=VERTEX_POINT ( 'NONE', #9467 ) ;
#9878=PLANE ( 'NONE',  #11213 ) ;
#9880=CIRCLE ( 'NONE', #3683, 62.91752772691707207 ) ;
#9883=CARTESIAN_POINT ( 'NONE',  ( -38.78191089773041256, 44.07268132743711675, 110.7293897666001214 ) ) ;
#9887=EDGE_CURVE ( 'NONE', #1021, #1356, #15710, .T. ) ;
#9890=DIRECTION ( 'NONE',  ( 1.000000000000000000, 0.000000000000000000, 0.000000000000000000 ) ) ;
#9892=EDGE_CURVE ( 'NONE', #5311, #15181, #12314, .T. ) ;
#9897=CARTESIAN_POINT ( 'NONE',  ( 0.000000000000000000, 0.000000000000000000, 132.4711112102474146 ) ) ;
#9899=VECTOR ( 'NONE', #11260, 1000.000000000000000 ) ;
#9902=CARTESIAN_POINT ( 'NONE',  ( 39.80940113486020948, -48.72193424476463974, 248.9926560891072143 ) ) ;
#9904=ORIENTED_EDGE ( 'NONE', *, *, #4094, .F. ) ;
#9906=CARTESIAN_POINT ( 'NONE',  ( -67.36461649554505016, 39.84224160888970800, 248.9926560891072143 ) ) ;
#9911=ORIENTED_EDGE ( 'NONE', *, *, #12889, .T. ) ;
#9912=DIRECTION ( 'NONE',  ( 1.000000000000000000, 0.000000000000000000, -0.000000000000000000 ) ) ;
#9914=CIRCLE ( 'NONE', #17441, 62.91752772691707207 ) ;
#9916=EDGE_CURVE ( 'NONE', #8891, #13644, #14688, .T. ) ;
#9918=DIRECTION ( 'NONE',  ( 0.7430374143461900838, -0.6692498792541753394, 0.000000000000000000 ) ) ;
#9919=CYLINDRICAL_SURFACE ( 'NONE', #13597, 79.75827554147308263 ) ;
#9920=DIRECTION ( 'NONE',  ( 1.000000000000000000, 0.000000000000000000, 0.000000000000000000 ) ) ;
#9921=VECTOR ( 'NONE', #14490, 1000.000000000000000 ) ;
#9926=VECTOR ( 'NONE', #6455, 1000.000000000000114 ) ;
#9927=CARTESIAN_POINT ( 'NONE',  ( 0.000000000000000000, 0.000000000000000000, 293.5832628385307999 ) ) ;
#9928=LINE ( 'NONE', #14827, #3932 ) ;
#9930=VERTEX_POINT ( 'NONE', #3429 ) ;
#9933=EDGE_LOOP ( 'NONE', ( #4158, #7307, #18644, #9166 ) ) ;
#9935=ORIENTED_EDGE ( 'NONE', *, *, #480, .T. ) ;
#9939=ORIENTED_EDGE ( 'NONE', *, *, #18417, .T. ) ;
#9940=CARTESIAN_POINT ( 'NONE',  ( -59.39925916207558743, -20.74471755083584057, 293.5832628385307999 ) ) ;
#9944=CARTESIAN_POINT ( 'NONE',  ( -59.39925916207559453, -20.74471755083585478, 248.9926560891072143 ) ) ;
#9949=CARTESIAN_POINT ( 'NONE',  ( 0.000000000000000000, 0.000000000000000000, 293.5832628385307999 ) ) ;
#9952=CARTESIAN_POINT ( 'NONE',  ( -39.84224160888947353, -67.36461649554519227, 132.4711112102474146 ) ) ;
#9954=CARTESIAN_POINT ( 'NONE',  ( -54.89456854707564304, -30.74413178637171740, 248.9926560891072143 ) ) ;
#9958=VERTEX_POINT ( 'NONE', #4973 ) ;
#9959=AXIS2_PLACEMENT_3D ( 'NONE', #4297, #19841, #18118 ) ;
#9963=CARTESIAN_POINT ( 'NONE',  ( -73.82206860051547892, -25.99419088092166774, 132.4711112102474146 ) ) ;
#9964=DIRECTION ( 'NONE',  ( -0.7660444431189749048, -0.6427876096865430267, 0.000000000000000000 ) ) ;
#9965=FACE_OUTER_BOUND ( 'NONE', #12256, .T. ) ;
#9974=DIRECTION ( 'NONE',  ( -0.2080686897406911207, -0.9781142164131917394, 0.000000000000000000 ) ) ;
#9975=EDGE_LOOP ( 'NONE', ( #15334, #16282, #8733, #6994 ) ) ;
#9976=EDGE_LOOP ( 'NONE', ( #5088, #15101, #5265, #2633 ) ) ;
#9982=VERTEX_POINT ( 'NONE', #14376 ) ;
#9983=EDGE_CURVE ( 'NONE', #7218, #5595, #8431, .T. ) ;
#9984=LINE ( 'NONE', #11318, #16781 ) ;
#9985=VERTEX_POINT ( 'NONE', #461 ) ;
#9986=LINE ( 'NONE', #3841, #2711 ) ;
#9992=ADVANCED_FACE ( 'NONE', ( #6904 ), #6807, .F. ) ;
#9993=ORIENTED_EDGE ( 'NONE', *, *, #14981, .F. ) ;
#9994=DIRECTION ( 'NONE',  ( -0.9271237148521536131, 0.3747554100459959958, 0.000000000000000000 ) ) ;
#9997=VECTOR ( 'NONE', #4851, 1000.000000000000000 ) ;
#9998=DIRECTION ( 'NONE',  ( 1.000000000000000000, 0.000000000000000000, 0.000000000000000000 ) ) ;
#9999=DIRECTION ( 'NONE',  ( 0.3747554100459959958, 0.9271237148521535021, 0.000000000000000000 ) ) ;
#10000=LINE ( 'NONE', #11915, #12284 ) ;
#10001=ORIENTED_EDGE ( 'NONE', *, *, #7035, .F. ) ;
#10003=EDGE_CURVE ( 'NONE', #16270, #6781, #5369, .T. ) ;
#10006=EDGE_CURVE ( 'NONE', #9930, #5962, #10118, .T. ) ;
#10009=CARTESIAN_POINT ( 'NONE',  ( -51.23821591265114961, -28.63313560863453944, 110.9660488491356887 ) ) ;
#10010=VERTEX_POINT ( 'NONE', #15913 ) ;
#10011=VECTOR ( 'NONE', #14993, 1000.000000000000000 ) ;
#10017=ORIENTED_EDGE ( 'NONE', *, *, #6606, .T. ) ;
#10018=AXIS2_PLACEMENT_3D ( 'NONE', #13447, #693, #11811 ) ;
#10019=EDGE_CURVE ( 'NONE', #9389, #2196, #11737, .T. ) ;
#10021=CARTESIAN_POINT ( 'NONE',  ( -37.78198917157318704, 47.56244194535179304, 283.5832628385307999 ) ) ;
#10024=VERTEX_POINT ( 'NONE', #1894 ) ;
#10026=LINE ( 'NONE', #8684, #15248 ) ;
#10030=ORIENTED_EDGE ( 'NONE', *, *, #15787, .F. ) ;
#10031=VECTOR ( 'NONE', #19264, 1000.000000000000227 ) ;
#10032=DIRECTION ( 'NONE',  ( -0.000000000000000000, -0.000000000000000000, 1.000000000000000000 ) ) ;
#10035=VERTEX_POINT ( 'NONE', #8327 ) ;
#10036=EDGE_CURVE ( 'NONE', #1970, #3220, #7494, .T. ) ;
#10037=EDGE_CURVE ( 'NONE', #4265, #12970, #2694, .T. ) ;
#10038=VERTEX_POINT ( 'NONE', #7391 ) ;
#10039=AXIS2_PLACEMENT_3D ( 'NONE', #8187, #11152, #12580 ) ;
#10040=ORIENTED_EDGE ( 'NONE', *, *, #3241, .T. ) ;
#10042=EDGE_CURVE ( 'NONE', #18312, #12789, #8533, .T. ) ;
#10043=FACE_OUTER_BOUND ( 'NONE', #2763, .T. ) ;
#10045=DIRECTION ( 'NONE',  ( 0.7660444431189858960, -0.6427876096865300370, 0.000000000000000000 ) ) ;
#10046=DIRECTION ( 'NONE',  ( 0.2080686897406943681, 0.9781142164131909622, 0.000000000000000000 ) ) ;
#10048=ORIENTED_EDGE ( 'NONE', *, *, #9267, .F. ) ;
#10054=AXIS2_PLACEMENT_3D ( 'NONE', #17361, #6411, #18893 ) ;
#10055=CARTESIAN_POINT ( 'NONE',  ( 53.87178215532755132, 28.06680738835045119, 283.5832628385307999 ) ) ;
#10056=CARTESIAN_POINT ( 'NONE',  ( 48.17959877923549072, 36.99514631729036296, 293.5832628385307999 ) ) ;
#10057=ORIENTED_EDGE ( 'NONE', *, *, #14050, .F. ) ;
#10058=PLANE ( 'NONE',  #10063 ) ;
#10059=LINE ( 'NONE', #13205, #11191 ) ;
#10061=ORIENTED_EDGE ( 'NONE', *, *, #17555, .T. ) ;
#10062=ADVANCED_FACE ( 'NONE', ( #5564 ), #11785, .T. ) ;
#10063=AXIS2_PLACEMENT_3D ( 'NONE', #7280, #8811, #18127 ) ;
#10064=EDGE_LOOP ( 'NONE', ( #19200, #6646, #500, #7933 ) ) ;
#10065=LINE ( 'NONE', #9963, #2736 ) ;
#10068=PLANE ( 'NONE',  #7819 ) ;
#10074=CARTESIAN_POINT ( 'NONE',  ( 68.18670162478805707, 38.41834839689404646, 248.9926560891072143 ) ) ;
#10075=AXIS2_PLACEMENT_3D ( 'NONE', #9305, #14319, #7966 ) ;
#10079=ORIENTED_EDGE ( 'NONE', *, *, #4117, .T. ) ;
#10080=VERTEX_POINT ( 'NONE', #15167 ) ;
#10083=VECTOR ( 'NONE', #16360, 1000.000000000000114 ) ;
#10084=EDGE_LOOP ( 'NONE', ( #8384, #17130, #1491, #3443 ) ) ;
#10086=CIRCLE ( 'NONE', #10719, 62.91752772691707207 ) ;
#10089=DIRECTION ( 'NONE',  ( -0.5300553768524376430, -0.8479630283625698706, 0.000000000000000000 ) ) ;
#10090=CARTESIAN_POINT ( 'NONE',  ( 0.000000000000000000, 0.000000000000000000, 293.5832628385307999 ) ) ;
#10092=CARTESIAN_POINT ( 'NONE',  ( -18.77710619359115896, -55.62246070845775137, 132.4711112102474146 ) ) ;
#10094=VERTEX_POINT ( 'NONE', #1149 ) ;
#10095=DIRECTION ( 'NONE',  ( 0.6427876096865404731, -0.7660444431189771253, 0.000000000000000000 ) ) ;
#10099=DIRECTION ( 'NONE',  ( 1.000000000000000000, 0.000000000000000000, 0.000000000000000000 ) ) ;
#10100=VECTOR ( 'NONE', #17834, 1000.000000000000000 ) ;
#10103=DIRECTION ( 'NONE',  ( -0.9848077530122091305, 0.1736481776669241417, 0.000000000000000000 ) ) ;
#10104=AXIS2_PLACEMENT_3D ( 'NONE', #12528, #8030, #17251 ) ;
#10108=ORIENTED_EDGE ( 'NONE', *, *, #3131, .F. ) ;
#10109=ORIENTED_EDGE ( 'NONE', *, *, #9724, .F. ) ;
#10110=ADVANCED_FACE ( 'NONE', ( #10258 ), #10068, .F. ) ;
#10112=ORIENTED_EDGE ( 'NONE', *, *, #8758, .F. ) ;
#10113=DIRECTION ( 'NONE',  ( 0.6427876096865328126, 0.7660444431189835646, 0.000000000000000000 ) ) ;
#10117=VECTOR ( 'NONE', #14380, 1000.000000000000000 ) ;
#10118=CIRCLE ( 'NONE', #5225, 60.74260934110282051 ) ;
#10119=ORIENTED_EDGE ( 'NONE', *, *, #17449, .F. ) ;
#10120=EDGE_CURVE ( 'NONE', #7092, #16671, #13522, .T. ) ;
#10123=CARTESIAN_POINT ( 'NONE',  ( -3.123743752083691039, 4.811834253408552087, 283.5832628385307999 ) ) ;
#10124=EDGE_CURVE ( 'NONE', #5311, #13590, #4554, .T. ) ;
#10125=CARTESIAN_POINT ( 'NONE',  ( -25.47058595421602689, -74.01264520835145788, 132.4711112102474146 ) ) ;
#10130=DIRECTION ( 'NONE',  ( -0.4999999999999979461, -0.8660254037844398178, 0.000000000000000000 ) ) ;
#10133=CYLINDRICAL_SURFACE ( 'NONE', #8581, 60.74260934110282051 ) ;
#10138=VERTEX_POINT ( 'NONE', #5667 ) ;
#10141=VERTEX_POINT ( 'NONE', #16515 ) ;
#10146=ADVANCED_FACE ( 'NONE', ( #17955 ), #2398, .F. ) ;
#10147=PLANE ( 'NONE',  #3611 ) ;
#10148=DIRECTION ( 'NONE',  ( -0.000000000000000000, -0.000000000000000000, 1.000000000000000000 ) ) ;
#10149=CARTESIAN_POINT ( 'NONE',  ( 0.000000000000000000, 0.000000000000000000, 293.5832628385307999 ) ) ;
#10151=LINE ( 'NONE', #16399, #5965 ) ;
#10152=ORIENTED_EDGE ( 'NONE', *, *, #18096, .T. ) ;
#10155=VERTEX_POINT ( 'NONE', #16319 ) ;
#10158=VERTEX_POINT ( 'NONE', #18238 ) ;
#10160=CARTESIAN_POINT ( 'NONE',  ( -12.23146955673647618, -77.31114765718488968, 112.0427633081292385 ) ) ;
#10161=DIRECTION ( 'NONE',  ( 0.000000000000000000, 0.000000000000000000, 1.000000000000000000 ) ) ;
#10162=DIRECTION ( 'NONE',  ( 0.3420201433256630508, 0.9396926207859104263, 0.000000000000000000 ) ) ;
#10164=CARTESIAN_POINT ( 'NONE',  ( -73.25972925305610772, 27.53920554013711097, 132.4711112102474146 ) ) ;
#10165=DIRECTION ( 'NONE',  ( 1.000000000000000000, 0.000000000000000000, 0.000000000000000000 ) ) ;
#10167=DIRECTION ( 'NONE',  ( 0.000000000000000000, 0.000000000000000000, 1.000000000000000000 ) ) ;
#10168=VECTOR ( 'NONE', #407, 1000.000000000000227 ) ;
#10171=VECTOR ( 'NONE', #19273, 1000.000000000000000 ) ;
#10173=ADVANCED_FACE ( 'NONE', ( #13315 ), #8725, .T. ) ;
#10174=ORIENTED_EDGE ( 'NONE', *, *, #14282, .F. ) ;
#10177=ORIENTED_EDGE ( 'NONE', *, *, #20232, .F. ) ;
#10179=EDGE_LOOP ( 'NONE', ( #9542, #1239, #13570, #17214 ) ) ;
#10180=CARTESIAN_POINT ( 'NONE',  ( 57.65577537092158877, -11.00103590902891249, 112.0427633081292385 ) ) ;
#10181=CARTESIAN_POINT ( 'NONE',  ( 51.23821591265094355, 28.63313560863489471, 110.9660488491356887 ) ) ;
#10185=LINE ( 'NONE', #14886, #15879 ) ;
#10186=CARTESIAN_POINT ( 'NONE',  ( 59.42266395395792955, -50.93469132750283279, 110.7293897666001214 ) ) ;
#10188=PLANE ( 'NONE',  #3571 ) ;
#10193=PLANE ( 'NONE',  #10018 ) ;
#10194=EDGE_LOOP ( 'NONE', ( #3779, #5355, #3094 ) ) ;
#10197=VECTOR ( 'NONE', #2377, 1000.000000000000000 ) ;
#10198=ORIENTED_EDGE ( 'NONE', *, *, #19474, .F. ) ;
#10200=PLANE ( 'NONE',  #10543 ) ;
#10202=VECTOR ( 'NONE', #1961, 1000.000000000000000 ) ;
#10204=CARTESIAN_POINT ( 'NONE',  ( 22.29928840491074382, 56.50138340076680521, 283.5832628385307999 ) ) ;
#10205=CARTESIAN_POINT ( 'NONE',  ( 60.08127757648377099, 8.938941455415205795, 293.5832628385307999 ) ) ;
#10207=DIRECTION ( 'NONE',  ( -0.000000000000000000, -0.000000000000000000, 1.000000000000000000 ) ) ;
#10208=EDGE_LOOP ( 'NONE', ( #1607, #6718, #794, #15726 ) ) ;
#10209=CYLINDRICAL_SURFACE ( 'NONE', #11956, 62.91752772691707207 ) ;
#10210=LINE ( 'NONE', #8485, #5518 ) ;
#10213=DIRECTION ( 'NONE',  ( -0.9993852124581887875, 0.03505990758545545621, 0.000000000000000000 ) ) ;
#10214=LINE ( 'NONE', #16472, #5711 ) ;
#10216=CARTESIAN_POINT ( 'NONE',  ( -28.63313560863435825, 51.23821591265124198, 248.9926560891072143 ) ) ;
#10219=ORIENTED_EDGE ( 'NONE', *, *, #3861, .F. ) ;
#10220=LINE ( 'NONE', #19345, #3217 ) ;
#10223=EDGE_CURVE ( 'NONE', #6348, #9156, #12297, .T. ) ;
#10226=AXIS2_PLACEMENT_3D ( 'NONE', #16454, #5597, #5214 ) ;
#10229=EDGE_CURVE ( 'NONE', #16043, #7379, #10086, .T. ) ;
#10239=CYLINDRICAL_SURFACE ( 'NONE', #3362, 62.91752772691707207 ) ;
#10240=CARTESIAN_POINT ( 'NONE',  ( -1.629865514042508456, -60.72073886220396588, 283.5832628385307999 ) ) ;
#10242=DIRECTION ( 'NONE',  ( 1.000000000000000000, 0.000000000000000000, 0.000000000000000000 ) ) ;
#10244=CARTESIAN_POINT ( 'NONE',  ( 2.605298826210336927, 5.111158570922247790, 283.5832628385307999 ) ) ;
#10246=VECTOR ( 'NONE', #6482, 1000.000000000000341 ) ;
#10249=ADVANCED_FACE ( 'NONE', ( #5869 ), #13729, .T. ) ;
#10254=DIRECTION ( 'NONE',  ( 1.000000000000000000, 0.000000000000000000, 0.000000000000000000 ) ) ;
#10255=CARTESIAN_POINT ( 'NONE',  ( 25.47058595421554372, 74.01264520835162841, 111.4180192758974499 ) ) ;
#10258=FACE_OUTER_BOUND ( 'NONE', #19368, .T. ) ;
#10260=FACE_OUTER_BOUND ( 'NONE', #5813, .T. ) ;
#10263=DIRECTION ( 'NONE',  ( 1.000000000000000000, -0.000000000000000000, 0.000000000000000000 ) ) ;
#10264=VECTOR ( 'NONE', #1485, 999.9999999999998863 ) ;
#10265=CYLINDRICAL_SURFACE ( 'NONE', #8846, 62.91752772691707207 ) ;
#10266=DIRECTION ( 'NONE',  ( -0.000000000000000000, -0.000000000000000000, 1.000000000000000000 ) ) ;
#10267=DIRECTION ( 'NONE',  ( -0.000000000000000000, -0.000000000000000000, 1.000000000000000000 ) ) ;
#10269=ORIENTED_EDGE ( 'NONE', *, *, #2128, .T. ) ;
#10270=ORIENTED_EDGE ( 'NONE', *, *, #8404, .F. ) ;
#10271=ADVANCED_FACE ( 'NONE', ( #14046 ), #19973, .T. ) ;
#10277=ADVANCED_FACE ( 'NONE', ( #5971 ), #17509, .T. ) ;
#10280=ORIENTED_EDGE ( 'NONE', *, *, #14317, .T. ) ;
#10283=LINE ( 'NONE', #10186, #16320 ) ;
#10286=PLANE ( 'NONE',  #5138 ) ;
#10288=VECTOR ( 'NONE', #8833, 1000.000000000000114 ) ;
#10293=LINE ( 'NONE', #16351, #16776 ) ;
#10294=ORIENTED_EDGE ( 'NONE', *, *, #17507, .T. ) ;
#10295=ORIENTED_EDGE ( 'NONE', *, *, #4258, .T. ) ;
#10296=DIRECTION ( 'NONE',  ( -0.4693298356057531429, 0.8830229359480288309, 0.000000000000000000 ) ) ;
#10298=VERTEX_POINT ( 'NONE', #15268 ) ;
#10301=LINE ( 'NONE', #2248, #11612 ) ;
#10304=EDGE_LOOP ( 'NONE', ( #13512, #1879, #13546, #8473 ) ) ;
#10305=DIRECTION ( 'NONE',  ( -0.000000000000000000, -0.000000000000000000, 1.000000000000000000 ) ) ;
#10307=DIRECTION ( 'NONE',  ( 0.000000000000000000, 0.000000000000000000, 1.000000000000000000 ) ) ;
#10308=LINE ( 'NONE', #19722, #14522 ) ;
#10309=EDGE_LOOP ( 'NONE', ( #11805, #12954, #5189 ) ) ;
#10310=DIRECTION ( 'NONE',  ( -0.3420201433256726542, 0.9396926207859068736, 0.000000000000000000 ) ) ;
#10312=DIRECTION ( 'NONE',  ( 1.047444401652940164E-14, -1.000000000000000000, 0.000000000000000000 ) ) ;
#10313=VERTEX_POINT ( 'NONE', #12402 ) ;
#10314=CARTESIAN_POINT ( 'NONE',  ( 60.22232964560483737, 7.948937137877944537, 293.5832628385307999 ) ) ;
#10315=LINE ( 'NONE', #17916, #18383 ) ;
#10316=VERTEX_POINT ( 'NONE', #1954 ) ;
#10317=VECTOR ( 'NONE', #3774, 1000.000000000000227 ) ;
#10318=ORIENTED_EDGE ( 'NONE', *, *, #37, .F. ) ;
#10320=EDGE_LOOP ( 'NONE', ( #17532, #6420, #11775, #12493 ) ) ;
#10321=EDGE_CURVE ( 'NONE', #7913, #1356, #926, .T. ) ;
#10322=LINE ( 'NONE', #15039, #18573 ) ;
#10326=DIRECTION ( 'NONE',  ( -0.000000000000000000, -0.000000000000000000, 1.000000000000000000 ) ) ;
#10330=CIRCLE ( 'NONE', #559, 60.74260934110282051 ) ;
#10331=EDGE_CURVE ( 'NONE', #1274, #15008, #4428, .T. ) ;
#10332=DIRECTION ( 'NONE',  ( -0.000000000000000000, -0.000000000000000000, 1.000000000000000000 ) ) ;
#10334=LINE ( 'NONE', #18033, #6957 ) ;
#10335=ORIENTED_EDGE ( 'NONE', *, *, #2197, .F. ) ;
#10339=CARTESIAN_POINT ( 'NONE',  ( 0.000000000000000000, 0.000000000000000000, 283.5832628385307999 ) ) ;
#10340=ORIENTED_EDGE ( 'NONE', *, *, #4155, .F. ) ;
#10341=ORIENTED_EDGE ( 'NONE', *, *, #11853, .T. ) ;
#10344=ADVANCED_FACE ( 'NONE', ( #3108 ), #19238, .F. ) ;
#10345=LINE ( 'NONE', #16601, #9020 ) ;
#10356=LINE ( 'NONE', #2207, #18039 ) ;
#10358=DIRECTION ( 'NONE',  ( 1.000000000000000000, 0.000000000000000000, 0.000000000000000000 ) ) ;
#10359=CARTESIAN_POINT ( 'NONE',  ( 19.23677882349201695, -57.61823435390814296, 293.5832628385307999 ) ) ;
#10361=EDGE_CURVE ( 'NONE', #9422, #8266, #5130, .T. ) ;
#10364=ORIENTED_EDGE ( 'NONE', *, *, #17750, .T. ) ;
#10367=EDGE_CURVE ( 'NONE', #6205, #1414, #15966, .T. ) ;
#10368=VERTEX_POINT ( 'NONE', #10021 ) ;
#10370=DIRECTION ( 'NONE',  ( 1.000000000000000000, 0.000000000000000000, 0.000000000000000000 ) ) ;
#10374=CIRCLE ( 'NONE', #261, 60.74260934110282051 ) ;
#10379=EDGE_CURVE ( 'NONE', #4335, #9958, #10210, .T. ) ;
#10380=LINE ( 'NONE', #16642, #9833 ) ;
#10383=EDGE_CURVE ( 'NONE', #10900, #14067, #14820, .T. ) ;
#10384=LINE ( 'NONE', #4255, #7128 ) ;
#10386=DIRECTION ( 'NONE',  ( 1.000000000000000000, 0.000000000000000000, -0.000000000000000000 ) ) ;
#10387=AXIS2_PLACEMENT_3D ( 'NONE', #8867, #12130, #15107 ) ;
#10388=VERTEX_POINT ( 'NONE', #5517 ) ;
#10390=VECTOR ( 'NONE', #4319, 999.9999999999998863 ) ;
#10391=VERTEX_POINT ( 'NONE', #6757 ) ;
#10392=LINE ( 'NONE', #11919, #4011 ) ;
#10393=VECTOR ( 'NONE', #6512, 1000.000000000000000 ) ;
#10394=ORIENTED_EDGE ( 'NONE', *, *, #17917, .F. ) ;
#10395=VERTEX_POINT ( 'NONE', #17709 ) ;
#10397=DIRECTION ( 'NONE',  ( -0.7071067811865472397, 8.659560562354930393E-17, 0.7071067811865479058 ) ) ;
#10398=DIRECTION ( 'NONE',  ( -0.000000000000000000, -0.000000000000000000, 1.000000000000000000 ) ) ;
#10399=LINE ( 'NONE', #12239, #4492 ) ;
#10400=DIRECTION ( 'NONE',  ( 0.000000000000000000, 0.000000000000000000, 1.000000000000000000 ) ) ;
#10401=CARTESIAN_POINT ( 'NONE',  ( -60.08127757648377099, -8.938941455415186255, 283.5832628385307999 ) ) ;
#10402=VERTEX_POINT ( 'NONE', #3681 ) ;
#10404=DIRECTION ( 'NONE',  ( 0.000000000000000000, 0.000000000000000000, 1.000000000000000000 ) ) ;
#10408=PLANE ( 'NONE',  #20075 ) ;
#10409=VECTOR ( 'NONE', #8727, 1000.000000000000000 ) ;
#10411=CARTESIAN_POINT ( 'NONE',  ( 38.41834839689379777, -68.18670162478818497, 248.9926560891072143 ) ) ;
#10415=ORIENTED_EDGE ( 'NONE', *, *, #2615, .T. ) ;
#10419=ORIENTED_EDGE ( 'NONE', *, *, #5112, .T. ) ;
#10420=DIRECTION ( 'NONE',  ( -0.000000000000000000, -0.000000000000000000, 1.000000000000000000 ) ) ;
#10422=VECTOR ( 'NONE', #11269, 1000.000000000000114 ) ;
#10425=LINE ( 'NONE', #16682, #15581 ) ;
#10427=DIRECTION ( 'NONE',  ( -0.3420201433256568335, -0.9396926207859126468, 0.000000000000000000 ) ) ;
#10430=CARTESIAN_POINT ( 'NONE',  ( 0.000000000000000000, 0.000000000000000000, 283.5832628385307999 ) ) ;
#10433=DIRECTION ( 'NONE',  ( 1.000000000000000000, 0.000000000000000000, 0.000000000000000000 ) ) ;
#10436=EDGE_LOOP ( 'NONE', ( #16406, #15620, #2537, #16625 ) ) ;
#10438=DIRECTION ( 'NONE',  ( 0.9848077530122097967, -0.1736481776669206722, 0.000000000000000000 ) ) ;
#10444=VERTEX_POINT ( 'NONE', #408 ) ;
#10445=CIRCLE ( 'NONE', #12741, 62.91752772691707207 ) ;
#10449=DIRECTION ( 'NONE',  ( -0.000000000000000000, -0.000000000000000000, 1.000000000000000000 ) ) ;
#10455=DIRECTION ( 'NONE',  ( -0.7881095627315619634, -0.6155349844899687950, 0.000000000000000000 ) ) ;
#10456=CARTESIAN_POINT ( 'NONE',  ( 44.79940644582654841, -41.02350267428983699, 293.5832628385307999 ) ) ;
#10457=ADVANCED_FACE ( 'NONE', ( #1001 ), #19925, .T. ) ;
#10458=EDGE_LOOP ( 'NONE', ( #17766, #16693 ) ) ;
#10459=ADVANCED_FACE ( 'NONE', ( #1314 ), #19822, .T. ) ;
#10463=EDGE_LOOP ( 'NONE', ( #16404, #13688, #8172, #5246 ) ) ;
#10464=ORIENTED_EDGE ( 'NONE', *, *, #4080, .T. ) ;
#10466=VERTEX_POINT ( 'NONE', #16861 ) ;
#10467=EDGE_CURVE ( 'NONE', #16270, #5054, #6823, .T. ) ;
#10468=ADVANCED_FACE ( 'NONE', ( #19719 ), #11930, .F. ) ;
#10470=CARTESIAN_POINT ( 'NONE',  ( -0.8220851292435327196, -62.91215678473957240, 248.9926560891072143 ) ) ;
#10471=FACE_OUTER_BOUND ( 'NONE', #12125, .T. ) ;
#10472=EDGE_LOOP ( 'NONE', ( #6234, #16108, #15311 ) ) ;
#10473=AXIS2_PLACEMENT_3D ( 'NONE', #549, #12914, #6390 ) ;
#10474=DIRECTION ( 'NONE',  ( 1.000000000000000000, 0.000000000000000000, 0.000000000000000000 ) ) ;
#10475=LINE ( 'NONE', #10575, #18609 ) ;
#10479=DIRECTION ( 'NONE',  ( -0.3420201433256694901, 0.9396926207859082059, 0.000000000000000000 ) ) ;
#10480=CARTESIAN_POINT ( 'NONE',  ( -10.52001906124801778, 3.255534882825997123, 248.9926560891072143 ) ) ;
#10481=EDGE_CURVE ( 'NONE', #8663, #10934, #8777, .T. ) ;
#10485=ORIENTED_EDGE ( 'NONE', *, *, #838, .T. ) ;
#10486=CARTESIAN_POINT ( 'NONE',  ( -18.92519137117329109, 56.02932139001825362, 248.9926560891072143 ) ) ;
#10489=LINE ( 'NONE', #18486, #15803 ) ;
#10493=EDGE_CURVE ( 'NONE', #11632, #7001, #8973, .T. ) ;
#10494=EDGE_CURVE ( 'NONE', #11413, #7733, #18194, .T. ) ;
#10495=CARTESIAN_POINT ( 'NONE',  ( 0.000000000000000000, 0.000000000000000000, 283.5832628385307999 ) ) ;
#10498=CARTESIAN_POINT ( 'NONE',  ( 0.000000000000000000, 0.000000000000000000, 248.9926560891072143 ) ) ;
#10499=DIRECTION ( 'NONE',  ( 0.000000000000000000, 0.000000000000000000, 1.000000000000000000 ) ) ;
#10502=CARTESIAN_POINT ( 'NONE',  ( -32.62092819947992695, -51.24245927909985454, 293.5832628385307999 ) ) ;
#10505=EDGE_CURVE ( 'NONE', #16088, #9468, #2853, .T. ) ;
#10508=CARTESIAN_POINT ( 'NONE',  ( -18.77710619359115896, -55.62246070845775137, 111.4180192758973931 ) ) ;
#10511=LINE ( 'NONE', #2963, #7776 ) ;
#10512=DIRECTION ( 'NONE',  ( 1.000000000000000000, 0.000000000000000000, -0.000000000000000000 ) ) ;
#10513=ORIENTED_EDGE ( 'NONE', *, *, #2365, .T. ) ;
#10514=ORIENTED_EDGE ( 'NONE', *, *, #2001, .T. ) ;
#10518=DIRECTION ( 'NONE',  ( -0.000000000000000000, -0.000000000000000000, 1.000000000000000000 ) ) ;
#10519=LINE ( 'NONE', #5835, #439 ) ;
#10520=CIRCLE ( 'NONE', #12486, 62.91752772691707207 ) ;
#10521=EDGE_LOOP ( 'NONE', ( #8764, #77, #18413, #15179 ) ) ;
#10524=CARTESIAN_POINT ( 'NONE',  ( -30.74413178637153976, 54.89456854707572830, 293.5832628385307999 ) ) ;
#10525=EDGE_CURVE ( 'NONE', #14438, #1213, #18401, .T. ) ;
#10526=AXIS2_PLACEMENT_3D ( 'NONE', #8808, #13402, #10242 ) ;
#10527=CARTESIAN_POINT ( 'NONE',  ( -5.281164089014727558, -2.240720816136031690, 293.5832628385307999 ) ) ;
#10528=CARTESIAN_POINT ( 'NONE',  ( 53.40245231972179596, 28.94983032429848535, 293.5832628385307999 ) ) ;
#10529=DIRECTION ( 'NONE',  ( 0.000000000000000000, 0.000000000000000000, 1.000000000000000000 ) ) ;
#10533=DIRECTION ( 'NONE',  ( 0.3420201433256630508, 0.9396926207859104263, -0.000000000000000000 ) ) ;
#10534=ORIENTED_EDGE ( 'NONE', *, *, #145, .F. ) ;
#10536=CARTESIAN_POINT ( 'NONE',  ( 0.000000000000000000, 0.000000000000000000, 283.5832628385307999 ) ) ;
#10537=DIRECTION ( 'NONE',  ( -0.000000000000000000, -0.000000000000000000, 1.000000000000000000 ) ) ;
#10538=VECTOR ( 'NONE', #3296, 1000.000000000000114 ) ;
#10539=CIRCLE ( 'NONE', #13469, 60.74260934110282051 ) ;
#10541=VERTEX_POINT ( 'NONE', #13784 ) ;
#10543=AXIS2_PLACEMENT_3D ( 'NONE', #10009, #13067, #17794 ) ;
#10545=LINE ( 'NONE', #14136, #5120 ) ;
#10547=ORIENTED_EDGE ( 'NONE', *, *, #4535, .T. ) ;
#10548=DIRECTION ( 'NONE',  ( -0.9848077530122092416, 0.1736481776669241694, 0.000000000000000000 ) ) ;
#10551=DIRECTION ( 'NONE',  ( 1.000000000000000000, 0.000000000000000000, 0.000000000000000000 ) ) ;
#10555=ORIENTED_EDGE ( 'NONE', *, *, #4589, .T. ) ;
#10560=CARTESIAN_POINT ( 'NONE',  ( 12.28122767885846400, -61.70726652483821084, 293.5832628385307999 ) ) ;
#10563=VERTEX_POINT ( 'NONE', #2750 ) ;
#10566=EDGE_LOOP ( 'NONE', ( #11443, #5490, #16527, #4160 ) ) ;
#10571=DIRECTION ( 'NONE',  ( -0.9271237148521547233, 0.3747554100459928872, 0.000000000000000000 ) ) ;
#10572=PLANE ( 'NONE',  #595 ) ;
#10573=ORIENTED_EDGE ( 'NONE', *, *, #9752, .T. ) ;
#10575=CARTESIAN_POINT ( 'NONE',  ( 44.79787735033391272, -41.02212542604627288, 283.5832628385307999 ) ) ;
#10576=ORIENTED_EDGE ( 'NONE', *, *, #4155, .T. ) ;
#10577=DIRECTION ( 'NONE',  ( -0.000000000000000000, -0.000000000000000000, 1.000000000000000000 ) ) ;
#10580=PLANE ( 'NONE',  #15725 ) ;
#10582=EDGE_CURVE ( 'NONE', #17735, #16054, #5195, .T. ) ;
#10584=VECTOR ( 'NONE', #2549, 1000.000000000000000 ) ;
#10585=DIRECTION ( 'NONE',  ( 1.000000000000000000, 3.491481338843133355E-15, -0.000000000000000000 ) ) ;
#10586=ORIENTED_EDGE ( 'NONE', *, *, #506, .F. ) ;
#10590=VERTEX_POINT ( 'NONE', #7647 ) ;
#10591=VERTEX_POINT ( 'NONE', #3357 ) ;
#10595=EDGE_CURVE ( 'NONE', #7405, #19299, #7751, .T. ) ;
#10596=LINE ( 'NONE', #1408, #2254 ) ;
#10597=LINE ( 'NONE', #12338, #5169 ) ;
#10599=AXIS2_PLACEMENT_3D ( 'NONE', #11227, #6545, #4803 ) ;
#10600=DIRECTION ( 'NONE',  ( 0.000000000000000000, 0.000000000000000000, -1.000000000000000000 ) ) ;
#10601=DIRECTION ( 'NONE',  ( -0.8479630283625698706, 0.5300553768524376430, 0.000000000000000000 ) ) ;
#10602=EDGE_LOOP ( 'NONE', ( #5880, #4905, #1348 ) ) ;
#10606=ORIENTED_EDGE ( 'NONE', *, *, #2283, .T. ) ;
#10607=EDGE_CURVE ( 'NONE', #15125, #18959, #1717, .T. ) ;
#10608=CARTESIAN_POINT ( 'NONE',  ( 41.02212542604613077, 44.79787735033405482, 283.5832628385307999 ) ) ;
#10609=EDGE_CURVE ( 'NONE', #2886, #17034, #15737, .T. ) ;
#10611=CIRCLE ( 'NONE', #4757, 62.91752772691707207 ) ;
#10612=CARTESIAN_POINT ( 'NONE',  ( -62.90240729679781850, -1.379293853801974779, 293.5832628385307999 ) ) ;
#10613=ORIENTED_EDGE ( 'NONE', *, *, #3022, .T. ) ;
#10615=CARTESIAN_POINT ( 'NONE',  ( -50.93469132750304595, -59.42266395395774481, 248.9926560891072143 ) ) ;
#10616=LINE ( 'NONE', #4596, #4354 ) ;
#10625=STYLED_ITEM ( 'NONE', ( #16067 ), #8201 ) ;
#10627=LINE ( 'NONE', #1333, #2774 ) ;
#10629=FACE_OUTER_BOUND ( 'NONE', #13987, .T. ) ;
#10632=ADVANCED_FACE ( 'NONE', ( #17179 ), #3060, .F. ) ;
#10634=EDGE_CURVE ( 'NONE', #4813, #7427, #5004, .T. ) ;
#10635=DIRECTION ( 'NONE',  ( -0.000000000000000000, -0.000000000000000000, 1.000000000000000000 ) ) ;
#10636=ADVANCED_FACE ( 'NONE', ( #1520 ), #15841, .F. ) ;
#10639=EDGE_CURVE ( 'NONE', #11211, #6009, #8055, .T. ) ;
#10641=DIRECTION ( 'NONE',  ( -0.4693298356057531429, 0.8830229359480288309, 0.000000000000000000 ) ) ;
#10642=CARTESIAN_POINT ( 'NONE',  ( 73.06915264522001507, 28.06281046684300762, 248.9926560891072143 ) ) ;
#10643=ORIENTED_EDGE ( 'NONE', *, *, #9774, .F. ) ;
#10644=ADVANCED_FACE ( 'NONE', ( #11023 ), #6541, .T. ) ;
#10649=ORIENTED_EDGE ( 'NONE', *, *, #10037, .T. ) ;
#10650=FACE_BOUND ( 'NONE', #4237, .T. ) ;
#10653=VECTOR ( 'NONE', #19115, 999.9999999999998863 ) ;
#10656=CARTESIAN_POINT ( 'NONE',  ( -37.93579148621510200, -68.46530598706782200, 110.9660488491356887 ) ) ;
#10658=CARTESIAN_POINT ( 'NONE',  ( 38.35506425062457225, 44.43084819159290788, 248.9926560891072143 ) ) ;
#10664=PLANE ( 'NONE',  #11777 ) ;
#10668=CARTESIAN_POINT ( 'NONE',  ( 0.000000000000000000, 0.000000000000000000, 283.5832628385307999 ) ) ;
#10669=ADVANCED_FACE ( 'NONE', ( #17281 ), #9394, .T. ) ;
#10671=ORIENTED_EDGE ( 'NONE', *, *, #16534, .F. ) ;
#10673=CIRCLE ( 'NONE', #11662, 60.74260934110282051 ) ;
#10678=ORIENTED_EDGE ( 'NONE', *, *, #8774, .F. ) ;
#10680=DIRECTION ( 'NONE',  ( 0.9993852124581887875, -0.03505990758545544927, 0.000000000000000000 ) ) ;
#10683=DIRECTION ( 'NONE',  ( 0.000000000000000000, 0.000000000000000000, -1.000000000000000000 ) ) ;
#10686=CARTESIAN_POINT ( 'NONE',  ( 57.55901709132171362, 11.54977938102105028, 132.4711112102474146 ) ) ;
#10687=VECTOR ( 'NONE', #19591, 1000.000000000000000 ) ;
#10689=AXIS2_PLACEMENT_3D ( 'NONE', #8438, #9974, #2008 ) ;
#10692=EDGE_LOOP ( 'NONE', ( #5958, #14907, #3387 ) ) ;
#10694=ORIENTED_EDGE ( 'NONE', *, *, #4334, .F. ) ;
#10698=DIRECTION ( 'NONE',  ( 1.000000000000000000, 0.000000000000000000, 0.000000000000000000 ) ) ;
#10699=ORIENTED_EDGE ( 'NONE', *, *, #16004, .F. ) ;
#10701=VECTOR ( 'NONE', #11902, 1000.000000000000000 ) ;
#10704=EDGE_CURVE ( 'NONE', #1551, #6246, #9453, .T. ) ;
#10707=ORIENTED_EDGE ( 'NONE', *, *, #8387, .T. ) ;
#10709=CARTESIAN_POINT ( 'NONE',  ( 2.244911526960062012E-13, -1.379293853801755176, 248.9926560891072143 ) ) ;
#10710=EDGE_LOOP ( 'NONE', ( #12553, #3468, #16818, #13618 ) ) ;
#10712=DIRECTION ( 'NONE',  ( 0.000000000000000000, 0.000000000000000000, 1.000000000000000000 ) ) ;
#10713=CARTESIAN_POINT ( 'NONE',  ( -50.93469132750304595, -59.42266395395774481, 110.7293897666001214 ) ) ;
#10714=VECTOR ( 'NONE', #8963, 1000.000000000000000 ) ;
#10716=CARTESIAN_POINT ( 'NONE',  ( 8.833100819207578169, 58.03804081968171147, 112.0427633081292953 ) ) ;
#10717=DIRECTION ( 'NONE',  ( 1.000000000000000000, 0.000000000000000000, 0.000000000000000000 ) ) ;
#10718=VECTOR ( 'NONE', #947, 1000.000000000000000 ) ;
#10719=AXIS2_PLACEMENT_3D ( 'NONE', #20077, #9338, #3481 ) ;
#10721=EDGE_CURVE ( 'NONE', #16961, #739, #15428, .T. ) ;
#10724=CARTESIAN_POINT ( 'NONE',  ( 49.67518383744835120, -60.47951622432768204, 132.4711112102474146 ) ) ;
#10726=EDGE_LOOP ( 'NONE', ( #9142, #14781, #560 ) ) ;
#10727=DIRECTION ( 'NONE',  ( 0.3088643371590157338, -0.9511061040868794558, 0.000000000000000000 ) ) ;
#10730=EDGE_CURVE ( 'NONE', #18597, #12303, #15982, .T. ) ;
#10731=CARTESIAN_POINT ( 'NONE',  ( -3.453261854573022482, -4.581103194069998885, 293.5832628385307999 ) ) ;
#10736=AXIS2_PLACEMENT_3D ( 'NONE', #12858, #5101, #11431 ) ;
#10739=DIRECTION ( 'NONE',  ( -0.7430374143461878633, 0.6692498792541777819, 0.000000000000000000 ) ) ;
#10747=EDGE_CURVE ( 'NONE', #55, #10158, #19506, .T. ) ;
#10749=CARTESIAN_POINT ( 'NONE',  ( -25.47058595421603044, -74.01264520835145788, 111.4180192758973931 ) ) ;
#10750=VERTEX_POINT ( 'NONE', #3752 ) ;
#10752=AXIS2_PLACEMENT_3D ( 'NONE', #3057, #6332, #18603 ) ;
#10753=EDGE_LOOP ( 'NONE', ( #11133, #11727, #3574, #4468 ) ) ;
#10755=ORIENTED_EDGE ( 'NONE', *, *, #7850, .T. ) ;
#10756=CARTESIAN_POINT ( 'NONE',  ( 51.24245927909996112, -32.62092819947974220, 283.5832628385307999 ) ) ;
#10757=FACE_BOUND ( 'NONE', #14856, .T. ) ;
#10763=DIRECTION ( 'NONE',  ( 0.8660254037844380415, 0.5000000000000009992, 0.000000000000000000 ) ) ;
#10767=AXIS2_PLACEMENT_3D ( 'NONE', #8923, #18047, #3824 ) ;
#10771=DIRECTION ( 'NONE',  ( -0.8660254037844415942, 0.4999999999999950040, 0.000000000000000000 ) ) ;
#10772=DIRECTION ( 'NONE',  ( -0.4999999999999888978, -0.8660254037844449249, 0.000000000000000000 ) ) ;
#10774=ORIENTED_EDGE ( 'NONE', *, *, #7850, .F. ) ;
#10775=EDGE_CURVE ( 'NONE', #10444, #7454, #585, .T. ) ;
#10781=ORIENTED_EDGE ( 'NONE', *, *, #12363, .F. ) ;
#10785=CARTESIAN_POINT ( 'NONE',  ( 0.000000000000000000, 0.000000000000000000, 83.57543755549745867 ) ) ;
#10786=ORIENTED_EDGE ( 'NONE', *, *, #12166, .T. ) ;
#10788=CARTESIAN_POINT ( 'NONE',  ( 61.70726652483817531, 12.28122767885865763, 248.9926560891072143 ) ) ;
#10793=LINE ( 'NONE', #9265, #11404 ) ;
#10794=CARTESIAN_POINT ( 'NONE',  ( 0.000000000000000000, 0.000000000000000000, 293.5832628385307999 ) ) ;
#10796=DIRECTION ( 'NONE',  ( 0.000000000000000000, 0.000000000000000000, -1.000000000000000000 ) ) ;
#10797=ORIENTED_EDGE ( 'NONE', *, *, #19603, .F. ) ;
#10799=ORIENTED_EDGE ( 'NONE', *, *, #9852, .T. ) ;
#10800=ORIENTED_EDGE ( 'NONE', *, *, #3663, .F. ) ;
#10801=DIRECTION ( 'NONE',  ( -0.1736481776669340227, 0.9848077530122073542, 0.000000000000000000 ) ) ;
#10805=AXIS2_PLACEMENT_3D ( 'NONE', #3417, #17232, #9552 ) ;
#10806=CARTESIAN_POINT ( 'NONE',  ( 0.000000000000000000, 0.000000000000000000, 83.57543755549745867 ) ) ;
#10809=ORIENTED_EDGE ( 'NONE', *, *, #15652, .T. ) ;
#10810=CARTESIAN_POINT ( 'NONE',  ( 37.78198917157319414, -47.56244194535177172, 283.5832628385307999 ) ) ;
#10813=AXIS2_PLACEMENT_3D ( 'NONE', #15697, #14153, #17641 ) ;
#10814=LINE ( 'NONE', #1416, #3803 ) ;
#10817=AXIS2_PLACEMENT_3D ( 'NONE', #12662, #19748, #11125 ) ;
#10819=CARTESIAN_POINT ( 'NONE',  ( 3.453261854573465683, 4.581103194070611728, 283.5832628385307999 ) ) ;
#10822=DIRECTION ( 'NONE',  ( 1.047444401652940007E-14, -1.000000000000000000, 0.000000000000000000 ) ) ;
#10823=ORIENTED_EDGE ( 'NONE', *, *, #3986, .F. ) ;
#10828=LINE ( 'NONE', #4499, #4034 ) ;
#10831=CARTESIAN_POINT ( 'NONE',  ( -19.74955734591987522, 8.656064874776506102, 248.9926560891072143 ) ) ;
#10834=LINE ( 'NONE', #10941, #16686 ) ;
#10840=ADVANCED_FACE ( 'NONE', ( #11715 ), #16343, .F. ) ;
#10841=CARTESIAN_POINT ( 'NONE',  ( -32.03743494504725930, 36.03492788066173347, 248.9926560891072143 ) ) ;
#10843=ORIENTED_EDGE ( 'NONE', *, *, #3104, .F. ) ;
#10844=EDGE_CURVE ( 'NONE', #5911, #13255, #17943, .T. ) ;
#10846=LINE ( 'NONE', #17101, #17747 ) ;
#10847=ADVANCED_FACE ( 'NONE', ( #6932 ), #8558, .F. ) ;
#10850=EDGE_CURVE ( 'NONE', #7403, #7735, #9100, .T. ) ;
#10851=ORIENTED_EDGE ( 'NONE', *, *, #14893, .T. ) ;
#10853=VECTOR ( 'NONE', #4826, 1000.000000000000114 ) ;
#10854=EDGE_LOOP ( 'NONE', ( #13661, #12227, #2662, #3794 ) ) ;
#10856=DIRECTION ( 'NONE',  ( 0.000000000000000000, 0.000000000000000000, -1.000000000000000000 ) ) ;
#10859=DIRECTION ( 'NONE',  ( -0.8830229359480288309, -0.4693298356057531984, 0.000000000000000000 ) ) ;
#10860=LINE ( 'NONE', #17223, #6681 ) ;
#10861=DIRECTION ( 'NONE',  ( 0.000000000000000000, 0.000000000000000000, 1.000000000000000000 ) ) ;
#10865=DIRECTION ( 'NONE',  ( 1.000000000000000000, 0.000000000000000000, 0.000000000000000000 ) ) ;
#10866=DIRECTION ( 'NONE',  ( 1.000000000000000000, 0.000000000000000000, 0.000000000000000000 ) ) ;
#10867=DIRECTION ( 'NONE',  ( 0.4693298356057564180, -0.8830229359480272766, 0.000000000000000000 ) ) ;
#10869=VECTOR ( 'NONE', #17003, 1000.000000000000000 ) ;
#10870=AXIS2_PLACEMENT_3D ( 'NONE', #9883, #16133, #17869 ) ;
#10875=CARTESIAN_POINT ( 'NONE',  ( -0.8220851292435327196, -78.26059000578311498, 132.4711112102474146 ) ) ;
#10876=ADVANCED_FACE ( 'NONE', ( #3660 ), #19116, .F. ) ;
#10877=VECTOR ( 'NONE', #1913, 1000.000000000000227 ) ;
#10878=ADVANCED_FACE ( 'NONE', ( #6733 ), #5104, .F. ) ;
#10881=VECTOR ( 'NONE', #14002, 1000.000000000000114 ) ;
#10882=EDGE_LOOP ( 'NONE', ( #10694, #16179, #15161, #12939 ) ) ;
#10885=CARTESIAN_POINT ( 'NONE',  ( 0.8220851292435327196, 78.26059000578311498, 132.4711112102474146 ) ) ;
#10888=LINE ( 'NONE', #17145, #19164 ) ;
#10889=DIRECTION ( 'NONE',  ( -0.7430374143461878633, 0.6692498792541777819, 0.000000000000000000 ) ) ;
#10890=DIRECTION ( 'NONE',  ( 0.000000000000000000, 0.000000000000000000, 1.000000000000000000 ) ) ;
#10891=CARTESIAN_POINT ( 'NONE',  ( 0.000000000000000000, 0.000000000000000000, 283.5832628385307999 ) ) ;
#10894=CARTESIAN_POINT ( 'NONE',  ( 0.8220851292435327196, 62.91215678473957240, 293.5832628385307999 ) ) ;
#10900=VERTEX_POINT ( 'NONE', #18074 ) ;
#10901=ORIENTED_EDGE ( 'NONE', *, *, #14008, .T. ) ;
#10903=VECTOR ( 'NONE', #14042, 1000.000000000000000 ) ;
#10904=EDGE_CURVE ( 'NONE', #13329, #8156, #4052, .T. ) ;
#10907=VECTOR ( 'NONE', #18570, 999.9999999999998863 ) ;
#10910=CARTESIAN_POINT ( 'NONE',  ( 41.02350267428969488, 44.79940644582669051, 283.5832628385307999 ) ) ;
#10911=DIRECTION ( 'NONE',  ( 1.000000000000000000, 0.000000000000000000, -0.000000000000000000 ) ) ;
#10912=FACE_OUTER_BOUND ( 'NONE', #3144, .T. ) ;
#10914=EDGE_LOOP ( 'NONE', ( #13363, #843, #16823, #8440 ) ) ;
#10916=DIRECTION ( 'NONE',  ( -0.1736481776669306920, 0.9848077530122080203, 0.000000000000000000 ) ) ;
#10917=ORIENTED_EDGE ( 'NONE', *, *, #9774, .T. ) ;
#10919=DIRECTION ( 'NONE',  ( -0.9271237148521547233, 0.3747554100459928872, 0.000000000000000000 ) ) ;
#10920=DIRECTION ( 'NONE',  ( 0.9396926207859114255, -0.3420201433256601642, 0.000000000000000000 ) ) ;
#10921=AXIS2_PLACEMENT_3D ( 'NONE', #7979, #19142, #412 ) ;
#10925=CARTESIAN_POINT ( 'NONE',  ( -10.11498556985118924, 62.09913334491134407, 248.9926560891072143 ) ) ;
#10931=VERTEX_POINT ( 'NONE', #16734 ) ;
#10932=CARTESIAN_POINT ( 'NONE',  ( -23.22718332831480481, -56.12853591711337486, 293.5832628385307999 ) ) ;
#10933=CIRCLE ( 'NONE', #2132, 62.91752772691707207 ) ;
#10934=VERTEX_POINT ( 'NONE', #2723 ) ;
#10936=DIRECTION ( 'NONE',  ( 1.000000000000000000, 0.000000000000000000, 0.000000000000000000 ) ) ;
#10939=DIRECTION ( 'NONE',  ( 1.000000000000000000, 0.000000000000000000, -0.000000000000000000 ) ) ;
#10941=CARTESIAN_POINT ( 'NONE',  ( 39.84224160888901167, 67.36461649554546227, 110.9660488491356887 ) ) ;
#10942=CARTESIAN_POINT ( 'NONE',  ( 45.46865632508072963, -40.28046525994365368, 283.5832628385307999 ) ) ;
#10947=CYLINDRICAL_SURFACE ( 'NONE', #12206, 62.91752772691707207 ) ;
#10950=CARTESIAN_POINT ( 'NONE',  ( 78.26059000578310076, 1.379293853802574077, 248.9926560891072143 ) ) ;
#10951=CARTESIAN_POINT ( 'NONE',  ( 0.000000000000000000, 0.000000000000000000, 283.5832628385307999 ) ) ;
#10952=ORIENTED_EDGE ( 'NONE', *, *, #6756, .T. ) ;
#10954=ORIENTED_EDGE ( 'NONE', *, *, #605, .T. ) ;
#10955=VERTEX_POINT ( 'NONE', #19599 ) ;
#10961=ORIENTED_EDGE ( 'NONE', *, *, #7900, .T. ) ;
#10962=LINE ( 'NONE', #4845, #5989 ) ;
#10964=CARTESIAN_POINT ( 'NONE',  ( -1.629937663769596368, -60.72279549541552512, 283.5832628385307999 ) ) ;
#10972=CARTESIAN_POINT ( 'NONE',  ( 12.23146955673593794, 77.31114765718498916, 132.4711112102474146 ) ) ;
#10976=ORIENTED_EDGE ( 'NONE', *, *, #6559, .T. ) ;
#10978=DIRECTION ( 'NONE',  ( 0.9396926207859068736, 0.3420201433256725987, 0.000000000000000000 ) ) ;
#10979=EDGE_CURVE ( 'NONE', #9227, #2560, #3950, .T. ) ;
#10983=VERTEX_POINT ( 'NONE', #2521 ) ;
#10986=CARTESIAN_POINT ( 'NONE',  ( -18.28503710798546678, 57.92514141135458772, 283.5832628385307999 ) ) ;
#10988=CARTESIAN_POINT ( 'NONE',  ( -51.77076963420845601, 31.77187437101486367, 283.5832628385307999 ) ) ;
#10992=DIRECTION ( 'NONE',  ( -0.3747554100459928317, -0.9271237148521548344, 0.000000000000000000 ) ) ;
#10996=ORIENTED_EDGE ( 'NONE', *, *, #5021, .T. ) ;
#10997=VECTOR ( 'NONE', #723, 999.9999999999998863 ) ;
#11001=CIRCLE ( 'NONE', #19508, 60.74260934110282051 ) ;
#11002=ORIENTED_EDGE ( 'NONE', *, *, #19983, .F. ) ;
#11003=ADVANCED_FACE ( 'NONE', ( #257 ), #6409, .T. ) ;
#11006=CYLINDRICAL_SURFACE ( 'NONE', #14476, 62.91752772691707207 ) ;
#11009=DIRECTION ( 'NONE',  ( 0.000000000000000000, 0.000000000000000000, 1.000000000000000000 ) ) ;
#11013=VERTEX_POINT ( 'NONE', #13962 ) ;
#11017=EDGE_CURVE ( 'NONE', #2887, #182, #7924, .T. ) ;
#11021=AXIS2_PLACEMENT_3D ( 'NONE', #162, #4128, #7105 ) ;
#11023=FACE_OUTER_BOUND ( 'NONE', #17968, .T. ) ;
#11024=PLANE ( 'NONE',  #11277 ) ;
#11026=LINE ( 'NONE', #16051, #18981 ) ;
#11028=EDGE_LOOP ( 'NONE', ( #4190, #13022, #5087, #9993 ) ) ;
#11030=EDGE_CURVE ( 'NONE', #9508, #15527, #10793, .T. ) ;
#11031=EDGE_LOOP ( 'NONE', ( #10671, #3273, #18087, #5676 ) ) ;
#11032=VECTOR ( 'NONE', #1619, 1000.000000000000000 ) ;
#11038=DIRECTION ( 'NONE',  ( 1.000000000000000000, 0.000000000000000000, -0.000000000000000000 ) ) ;
#11039=ORIENTED_EDGE ( 'NONE', *, *, #13054, .F. ) ;
#11040=EDGE_CURVE ( 'NONE', #4473, #5793, #7722, .T. ) ;
#11042=DIRECTION ( 'NONE',  ( 0.000000000000000000, 0.000000000000000000, 1.000000000000000000 ) ) ;
#11047=CIRCLE ( 'NONE', #2892, 60.74260934110282051 ) ;
#11048=VERTEX_POINT ( 'NONE', #3033 ) ;
#11054=CARTESIAN_POINT ( 'NONE',  ( -8.833100819207983179, -58.03804081968163331, 132.4711112102474146 ) ) ;
#11058=EDGE_LOOP ( 'NONE', ( #18307, #17672, #11314, #4570 ) ) ;
#11065=CARTESIAN_POINT ( 'NONE',  ( -26.04958516073518382, 47.87779272208825176, 248.9926560891072143 ) ) ;
#11066=EDGE_LOOP ( 'NONE', ( #16243, #15824, #9245, #3142 ) ) ;
#11068=CARTESIAN_POINT ( 'NONE',  ( 0.000000000000000000, 0.000000000000000000, 293.5832628385307999 ) ) ;
#11072=DIRECTION ( 'NONE',  ( -0.9396926207859057634, -0.3420201433256757073, 0.000000000000000000 ) ) ;
#11077=AXIS2_PLACEMENT_3D ( 'NONE', #385, #16142, #13245 ) ;
#11081=CARTESIAN_POINT ( 'NONE',  ( 38.41834839689379777, -68.18670162478817076, 132.4711112102474146 ) ) ;
#11083=ORIENTED_EDGE ( 'NONE', *, *, #14050, .T. ) ;
#11085=AXIS2_PLACEMENT_3D ( 'NONE', #19837, #5834, #13286 ) ;
#11088=FACE_OUTER_BOUND ( 'NONE', #20175, .T. ) ;
#11089=DIRECTION ( 'NONE',  ( 1.000000000000000000, 0.000000000000000000, 0.000000000000000000 ) ) ;
#11090=CARTESIAN_POINT ( 'NONE',  ( 0.000000000000000000, 0.000000000000000000, 293.5832628385307999 ) ) ;
#11091=EDGE_CURVE ( 'NONE', #19300, #3549, #15815, .T. ) ;
#11093=CARTESIAN_POINT ( 'NONE',  ( -44.43084819159250287, 38.35506425062501989, 248.9926560891072143 ) ) ;
#11094=DIRECTION ( 'NONE',  ( 0.000000000000000000, 0.000000000000000000, 1.000000000000000000 ) ) ;
#11098=ORIENTED_EDGE ( 'NONE', *, *, #4298, .F. ) ;
#11103=EDGE_LOOP ( 'NONE', ( #17472, #17317, #7213, #13925 ) ) ;
#11105=ORIENTED_EDGE ( 'NONE', *, *, #16479, .F. ) ;
#11109=DIRECTION ( 'NONE',  ( 1.000000000000000000, 0.000000000000000000, 0.000000000000000000 ) ) ;
#11110=EDGE_LOOP ( 'NONE', ( #8171, #3154, #19936 ) ) ;
#11113=VECTOR ( 'NONE', #5328, 1000.000000000000000 ) ;
#11115=EDGE_CURVE ( 'NONE', #15357, #108, #5352, .T. ) ;
#11119=DIRECTION ( 'NONE',  ( -0.5000000000000039968, 0.8660254037844363761, 0.000000000000000000 ) ) ;
#11120=CARTESIAN_POINT ( 'NONE',  ( 0.000000000000000000, 0.000000000000000000, 132.4711112102474146 ) ) ;
#11122=VERTEX_POINT ( 'NONE', #6102 ) ;
#11124=DIRECTION ( 'NONE',  ( -0.3420201433256602197, -0.9396926207859115365, 0.000000000000000000 ) ) ;
#11125=DIRECTION ( 'NONE',  ( 1.000000000000000000, 0.000000000000000000, 0.000000000000000000 ) ) ;
#11126=CARTESIAN_POINT ( 'NONE',  ( 0.000000000000000000, 0.000000000000000000, 269.6944534026102360 ) ) ;
#11127=CARTESIAN_POINT ( 'NONE',  ( 50.93469132750264095, 59.42266395395811429, 132.4711112102474146 ) ) ;
#11131=AXIS2_PLACEMENT_3D ( 'NONE', #9897, #690, #586 ) ;
#11132=FACE_OUTER_BOUND ( 'NONE', #2695, .T. ) ;
#11133=ORIENTED_EDGE ( 'NONE', *, *, #10361, .F. ) ;
#11134=ADVANCED_FACE ( 'NONE', ( #6311 ), #9770, .T. ) ;
#11135=VECTOR ( 'NONE', #7158, 1000.000000000000000 ) ;
#11136=ORIENTED_EDGE ( 'NONE', *, *, #10493, .T. ) ;
#11139=ORIENTED_EDGE ( 'NONE', *, *, #10124, .T. ) ;
#11142=VERTEX_POINT ( 'NONE', #16221 ) ;
#11143=DIRECTION ( 'NONE',  ( 1.000000000000000000, 0.000000000000000000, 0.000000000000000000 ) ) ;
#11145=VECTOR ( 'NONE', #14938, 1000.000000000000114 ) ;
#11146=EDGE_CURVE ( 'NONE', #15308, #18601, #12933, .T. ) ;
#11147=VECTOR ( 'NONE', #16919, 1000.000000000000000 ) ;
#11148=DIRECTION ( 'NONE',  ( -0.7660444431189835646, 0.6427876096865328126, 0.000000000000000000 ) ) ;
#11149=DIRECTION ( 'NONE',  ( -0.000000000000000000, -0.000000000000000000, 1.000000000000000000 ) ) ;
#11150=ORIENTED_EDGE ( 'NONE', *, *, #9209, .F. ) ;
#11151=DIRECTION ( 'NONE',  ( 0.7660444431189792347, -0.6427876096865379196, 0.000000000000000000 ) ) ;
#11152=DIRECTION ( 'NONE',  ( -0.000000000000000000, -0.000000000000000000, 1.000000000000000000 ) ) ;
#11156=LINE ( 'NONE', #9826, #5826 ) ;
#11158=EDGE_CURVE ( 'NONE', #5962, #5133, #15917, .T. ) ;
#11159=ORIENTED_EDGE ( 'NONE', *, *, #15739, .T. ) ;
#11163=ORIENTED_EDGE ( 'NONE', *, *, #18932, .T. ) ;
#11164=EDGE_CURVE ( 'NONE', #9389, #9422, #8436, .T. ) ;
#11166=CARTESIAN_POINT ( 'NONE',  ( -45.84586732611835913, 36.66871011346426457, 132.4711112102474146 ) ) ;
#11167=ORIENTED_EDGE ( 'NONE', *, *, #705, .F. ) ;
#11168=EDGE_CURVE ( 'NONE', #14479, #4599, #5182, .T. ) ;
#11171=DIRECTION ( 'NONE',  ( 0.000000000000000000, 0.000000000000000000, 1.000000000000000000 ) ) ;
#11172=CARTESIAN_POINT ( 'NONE',  ( 62.18629025319814474, -9.564549117045299198, 293.5832628385307999 ) ) ;
#11174=CARTESIAN_POINT ( 'NONE',  ( 5.281164089014827923, 2.240720816136096083, 283.5832628385307999 ) ) ;
#11175=DIRECTION ( 'NONE',  ( 0.4999999999999950040, 0.8660254037844415942, 0.000000000000000000 ) ) ;
#11177=CARTESIAN_POINT ( 'NONE',  ( 38.35506425062457225, 44.43084819159290788, 110.7293897666001214 ) ) ;
#11179=CARTESIAN_POINT ( 'NONE',  ( 0.000000000000000000, 0.000000000000000000, 293.5832628385307999 ) ) ;
#11181=DIRECTION ( 'NONE',  ( -0.000000000000000000, -0.000000000000000000, 1.000000000000000000 ) ) ;
#11183=VECTOR ( 'NONE', #17851, 1000.000000000000114 ) ;
#11188=ORIENTED_EDGE ( 'NONE', *, *, #13518, .T. ) ;
#11191=VECTOR ( 'NONE', #5356, 1000.000000000000000 ) ;
#11192=PLANE ( 'NONE',  #6813 ) ;
#11194=DIRECTION ( 'NONE',  ( -0.000000000000000000, -0.000000000000000000, 1.000000000000000000 ) ) ;
#11198=CIRCLE ( 'NONE', #15451, 62.91752772691707207 ) ;
#11201=VERTEX_POINT ( 'NONE', #17461 ) ;
#11203=DIRECTION ( 'NONE',  ( -0.9993852124581887875, 0.03505990758545545621, 0.000000000000000000 ) ) ;
#11204=ORIENTED_EDGE ( 'NONE', *, *, #13216, .F. ) ;
#11205=VECTOR ( 'NONE', #2040, 1000.000000000000000 ) ;
#11207=ORIENTED_EDGE ( 'NONE', *, *, #20167, .F. ) ;
#11208=ORIENTED_EDGE ( 'NONE', *, *, #9603, .T. ) ;
#11210=DIRECTION ( 'NONE',  ( 0.03505990758545895342, 0.9993852124581886764, 0.000000000000000000 ) ) ;
#11211=VERTEX_POINT ( 'NONE', #3730 ) ;
#11212=CARTESIAN_POINT ( 'NONE',  ( -11.54977938102048007, 57.55901709132182731, 112.0427633081291816 ) ) ;
#11213=AXIS2_PLACEMENT_3D ( 'NONE', #16127, #2118, #19305 ) ;
#11215=FACE_OUTER_BOUND ( 'NONE', #17553, .T. ) ;
#11217=ORIENTED_EDGE ( 'NONE', *, *, #6244, .F. ) ;
#11219=CARTESIAN_POINT ( 'NONE',  ( 3.123743752084413128, -4.811834253409454476, 283.5832628385307999 ) ) ;
#11221=EDGE_CURVE ( 'NONE', #10541, #1274, #12833, .T. ) ;
#11222=CARTESIAN_POINT ( 'NONE',  ( -4.196299268919082337, -3.911853314815666671, 293.5832628385307999 ) ) ;
#11223=CARTESIAN_POINT ( 'NONE',  ( 0.000000000000000000, 0.000000000000000000, 132.4711112102474146 ) ) ;
#11225=CARTESIAN_POINT ( 'NONE',  ( -49.67518383744793908, 60.47951622432801599, 248.9926560891072143 ) ) ;
#11226=ADVANCED_FACE ( 'NONE', ( #19092 ), #16117, .T. ) ;
#11227=CARTESIAN_POINT ( 'NONE',  ( -36.66871011346412246, -45.84586732611848703, 110.7293897666001214 ) ) ;
#11228=DIRECTION ( 'NONE',  ( 0.03505990758545895342, 0.9993852124581886764, 0.000000000000000000 ) ) ;
#11229=VECTOR ( 'NONE', #11858, 1000.000000000000000 ) ;
#11230=CARTESIAN_POINT ( 'NONE',  ( -54.07248341783231638, 32.16802499836798290, 248.9926560891072143 ) ) ;
#11235=EDGE_LOOP ( 'NONE', ( #2745, #5990, #4945, #9170 ) ) ;
#11236=VERTEX_POINT ( 'NONE', #2208 ) ;
#11237=ADVANCED_FACE ( 'NONE', ( #11502 ), #665, .T. ) ;
#11247=AXIS2_PLACEMENT_3D ( 'NONE', #17656, #10161, #2201 ) ;
#11250=EDGE_CURVE ( 'NONE', #12652, #15683, #1951, .T. ) ;
#11252=CARTESIAN_POINT ( 'NONE',  ( 0.000000000000000000, 0.000000000000000000, 248.9926560891072143 ) ) ;
#11253=EDGE_LOOP ( 'NONE', ( #1606, #19828, #452 ) ) ;
#11254=FACE_OUTER_BOUND ( 'NONE', #2116, .T. ) ;
#11255=CARTESIAN_POINT ( 'NONE',  ( -12.23146955673647795, -77.31114765718486126, 248.9926560891072143 ) ) ;
#11259=DIRECTION ( 'NONE',  ( 0.000000000000000000, 0.000000000000000000, 1.000000000000000000 ) ) ;
#11260=DIRECTION ( 'NONE',  ( -0.000000000000000000, -0.000000000000000000, 1.000000000000000000 ) ) ;
#11261=EDGE_LOOP ( 'NONE', ( #19694, #10079, #8185, #13769 ) ) ;
#11264=ORIENTED_EDGE ( 'NONE', *, *, #20219, .T. ) ;
#11268=EDGE_CURVE ( 'NONE', #3720, #17381, #221, .T. ) ;
#11269=DIRECTION ( 'NONE',  ( 0.8660254037844449249, -0.4999999999999888423, 0.000000000000000000 ) ) ;
#11274=LINE ( 'NONE', #6587, #19720 ) ;
#11276=EDGE_CURVE ( 'NONE', #1059, #1114, #6376, .T. ) ;
#11277=AXIS2_PLACEMENT_3D ( 'NONE', #4910, #7956, #186 ) ;
#11285=DIRECTION ( 'NONE',  ( -0.000000000000000000, -0.000000000000000000, 1.000000000000000000 ) ) ;
#11286=DIRECTION ( 'NONE',  ( 1.000000000000000000, 0.000000000000000000, 0.000000000000000000 ) ) ;
#11292=ORIENTED_EDGE ( 'NONE', *, *, #1732, .F. ) ;
#11293=ORIENTED_EDGE ( 'NONE', *, *, #15044, .T. ) ;
#11296=AXIS2_PLACEMENT_3D ( 'NONE', #1298, #4360, #10386 ) ;
#11299=EDGE_CURVE ( 'NONE', #15754, #13585, #1864, .T. ) ;
#11310=PLANE ( 'NONE',  #16926 ) ;
#11313=ORIENTED_EDGE ( 'NONE', *, *, #17847, .T. ) ;
#11314=ORIENTED_EDGE ( 'NONE', *, *, #13037, .T. ) ;
#11315=CLOSED_SHELL ( 'NONE', ( #19654, #3355, #5052, #14738, #12724, #10271, #1216, #4718, #13645, #8744, #5464, #1013, #4133, #18392, #10669, #19616, #12618, #7786, #7641, #10847, #18875, #4466, #2039, #10062, #11003, #11955, #8889, #11486, #1122, #17009, #2869, #3092, #12004, #16784, #16526, #2480, #2114, #12791, #11371, #8147, #2666, #2554, #10468, #603, #4919, #16607, #8827, #18475, #18762, #6620, #841, #10457, #2028, #11226, #16162, #3914, #1842, #15738, #5268, #10344, #6402, #12287, #11879, #14294, #7658, #8975, #3546, #8987, #10878, #11134, #4897, #9407, #849, #3766, #7481, #19842, #8422, #13262, #12513, #11745, #793, #19738, #2229, #4867, #9037, #10459, #2219, #13496, #9120, #1605, #14896, #1016, #8505, #10277, #9384, #7116, #15553, #13719, #18518, #19745, #10644, #9859, #3627, #11585, #14541, #5283, #16358, #18615, #6148, #2655, #16773, #5629, #2990, #19596, #18000, #12810, #16709, #3437, #5732, #20078, #6308, #10840, #1497, #8849, #16847, #6107, #16648, #12612, #400, #14760, #6894, #12634, #8909, #146, #20026, #4518, #523, #1631, #13739, #14741, #9293, #18377, #7760, #16409, #7257, #2412, #7387, #15985, #7874, #15356, #16250, #6111, #1882, #15902, #19351, #16033, #1227, #19066, #10110, #9666, #6677, #13744, #4130, #15119, #469, #13483, #1158, #15353, #17604, #14402, #8286, #7041, #15358, #15145, #14604, #20023, #11899, #2522, #3722, #972, #9992, #1791, #16304, #13589, #3342, #13890, #18782, #14627, #10876, #18306, #16738, #3359, #13387, #10632, #2742, #717, #7474, #4923, #11758, #16554, #7695, #14545, #14672, #2374, #15096, #10636, #2049, #7732, #12913, #5900, #16024, #16046, #7587, #12471, #9486, #10146, #14844, #1635, #14873, #1241, #12538, #16236, #18750, #19195, #15383, #20154, #8107, #5503, #2813, #20155, #1246, #148, #4924, #3040, #17646, #3661, #13953, #20111, #1737, #17865, #9153, #7967, #19242, #1127, #13017, #5886, #7865, #951, #15037, #6564, #2713, #2025, #17022, #19971, #11504, #6473, #17154, #13241, #901, #18208, #18026, #16263, #18747, #2642, #7609, #19042, #16969, #14867, #1404, #3521, #9805, #2733, #16720, #6736, #16401, #1909, #18112, #12921, #10249, #15619, #2117, #20088, #19187, #19154, #6505, #5489, #4858, #13270, #2112, #2795, #10173, #11237, #17775, #124, #7374, #6413, #9775, #17637, #16661, #4547, #17798, #43, #17296, #5039, #2413, #11354 ) ) ;
#11318=CARTESIAN_POINT ( 'NONE',  ( 49.67518383744835120, -60.47951622432767493, 132.4711112102474146 ) ) ;
#11321=CARTESIAN_POINT ( 'NONE',  ( 73.06915264522001507, 28.06281046684300406, 111.4180192758973362 ) ) ;
#11324=DIRECTION ( 'NONE',  ( -0.1390141521205912334, 0.9902903945359629034, 0.000000000000000000 ) ) ;
#11327=LINE ( 'NONE', #17583, #16630 ) ;
#11328=AXIS2_PLACEMENT_3D ( 'NONE', #17981, #9994, #13244 ) ;
#11329=ORIENTED_EDGE ( 'NONE', *, *, #23, .F. ) ;
#11330=AXIS2_PLACEMENT_3D ( 'NONE', #16293, #5632, #2276 ) ;
#11332=CARTESIAN_POINT ( 'NONE',  ( 0.000000000000000000, 0.000000000000000000, 283.5832628385307999 ) ) ;
#11333=CARTESIAN_POINT ( 'NONE',  ( 0.000000000000000000, 0.000000000000000000, 283.5832628385307999 ) ) ;
#11335=DIRECTION ( 'NONE',  ( 0.000000000000000000, 0.000000000000000000, 1.000000000000000000 ) ) ;
#11338=CARTESIAN_POINT ( 'NONE',  ( 60.68567895461851691, -2.629250726500488078, 293.5832628385307999 ) ) ;
#11340=ORIENTED_EDGE ( 'NONE', *, *, #10979, .T. ) ;
#11341=DIRECTION ( 'NONE',  ( 1.000000000000000000, 0.000000000000000000, 0.000000000000000000 ) ) ;
#11342=EDGE_LOOP ( 'NONE', ( #12773, #1764, #2141, #13820 ) ) ;
#11343=EDGE_LOOP ( 'NONE', ( #14686, #15254, #13919, #19354 ) ) ;
#11345=EDGE_CURVE ( 'NONE', #7430, #12535, #6581, .T. ) ;
#11347=DIRECTION ( 'NONE',  ( -0.7881095627315599650, -0.6155349844899714595, 0.000000000000000000 ) ) ;
#11348=CIRCLE ( 'NONE', #13621, 60.74260934110282051 ) ;
#11350=ORIENTED_EDGE ( 'NONE', *, *, #13614, .T. ) ;
#11351=CYLINDRICAL_SURFACE ( 'NONE', #15865, 62.91752772691707207 ) ;
#11354=ADVANCED_FACE ( 'NONE', ( #5150 ), #8600, .T. ) ;
#11355=DIRECTION ( 'NONE',  ( 1.000000000000000000, 0.000000000000000000, 0.000000000000000000 ) ) ;
#11356=DIRECTION ( 'NONE',  ( -0.000000000000000000, -0.000000000000000000, 1.000000000000000000 ) ) ;
#11357=EDGE_CURVE ( 'NONE', #998, #8067, #13000, .T. ) ;
#11360=CARTESIAN_POINT ( 'NONE',  ( 28.94983032429829350, -53.40245231972188833, 283.5832628385307999 ) ) ;
#11363=ORIENTED_EDGE ( 'NONE', *, *, #9892, .T. ) ;
#11364=VECTOR ( 'NONE', #2934, 1000.000000000000227 ) ;
#11365=FACE_OUTER_BOUND ( 'NONE', #2862, .T. ) ;
#11366=CARTESIAN_POINT ( 'NONE',  ( -49.07263256785925876, 39.37628763770471352, 293.5832628385307999 ) ) ;
#11367=ORIENTED_EDGE ( 'NONE', *, *, #8758, .T. ) ;
#11369=ORIENTED_EDGE ( 'NONE', *, *, #1685, .F. ) ;
#11371=ADVANCED_FACE ( 'NONE', ( #14643 ), #8300, .T. ) ;
#11374=EDGE_CURVE ( 'NONE', #4761, #10591, #534, .T. ) ;
#11378=DIRECTION ( 'NONE',  ( 0.7660444431189835646, -0.6427876096865328126, 0.000000000000000000 ) ) ;
#11381=CIRCLE ( 'NONE', #19537, 60.74260934110282051 ) ;
#11384=EDGE_CURVE ( 'NONE', #11211, #2196, #14446, .T. ) ;
#11391=CIRCLE ( 'NONE', #8448, 60.74260934110282051 ) ;
#11394=VERTEX_POINT ( 'NONE', #14546 ) ;
#11397=EDGE_CURVE ( 'NONE', #1972, #11122, #7071, .T. ) ;
#11398=VERTEX_POINT ( 'NONE', #432 ) ;
#11399=CARTESIAN_POINT ( 'NONE',  ( 20.74471755083603952, -59.39925916207552348, 132.4711112102474146 ) ) ;
#11401=CARTESIAN_POINT ( 'NONE',  ( -51.51682027493045979, 28.15057869795642986, 132.4711112102474146 ) ) ;
#11402=VECTOR ( 'NONE', #7471, 999.9999999999998863 ) ;
#11404=VECTOR ( 'NONE', #14277, 1000.000000000000114 ) ;
#11405=AXIS2_PLACEMENT_3D ( 'NONE', #16832, #16729, #19898 ) ;
#11406=CARTESIAN_POINT ( 'NONE',  ( -30.74413178637154687, 54.89456854707574252, 132.4711112102474146 ) ) ;
#11407=AXIS2_PLACEMENT_3D ( 'NONE', #9132, #18240, #4228 ) ;
#11408=EDGE_CURVE ( 'NONE', #9389, #5911, #3985, .T. ) ;
#11409=DIRECTION ( 'NONE',  ( -0.5300553768524376430, -0.8479630283625698706, 0.000000000000000000 ) ) ;
#11410=DIRECTION ( 'NONE',  ( 0.000000000000000000, 0.000000000000000000, 1.000000000000000000 ) ) ;
#11413=VERTEX_POINT ( 'NONE', #8696 ) ;
#11414=DIRECTION ( 'NONE',  ( -0.000000000000000000, -0.000000000000000000, 1.000000000000000000 ) ) ;
#11416=ORIENTED_EDGE ( 'NONE', *, *, #1658, .F. ) ;
#11417=ORIENTED_EDGE ( 'NONE', *, *, #2895, .F. ) ;
#11419=EDGE_CURVE ( 'NONE', #2611, #6324, #12054, .T. ) ;
#11421=CIRCLE ( 'NONE', #13697, 60.74260934110282051 ) ;
#11423=ORIENTED_EDGE ( 'NONE', *, *, #18462, .F. ) ;
#11425=EDGE_CURVE ( 'NONE', #195, #18230, #2465, .T. ) ;
#11426=DIRECTION ( 'NONE',  ( 0.1736481776669207000, 0.9848077530122097967, 0.000000000000000000 ) ) ;
#11427=DIRECTION ( 'NONE',  ( 0.1736481776669241417, 0.9848077530122091305, 0.000000000000000000 ) ) ;
#11429=EDGE_LOOP ( 'NONE', ( #18835, #15386, #19864, #19205 ) ) ;
#11431=DIRECTION ( 'NONE',  ( 1.000000000000000000, 0.000000000000000000, 0.000000000000000000 ) ) ;
#11434=DIRECTION ( 'NONE',  ( 1.000000000000000000, 0.000000000000000000, 0.000000000000000000 ) ) ;
#11436=DIRECTION ( 'NONE',  ( -0.7660444431189707970, -0.6427876096865481337, 0.000000000000000000 ) ) ;
#11438=DIRECTION ( 'NONE',  ( -0.5300553768524376430, -0.8479630283625698706, 0.000000000000000000 ) ) ;
#11441=CARTESIAN_POINT ( 'NONE',  ( -78.26059000578311498, 0.8220851292432594937, 132.4711112102474146 ) ) ;
#11442=VERTEX_POINT ( 'NONE', #15134 ) ;
#11443=ORIENTED_EDGE ( 'NONE', *, *, #6675, .T. ) ;
#11444=CARTESIAN_POINT ( 'NONE',  ( 0.000000000000000000, 0.000000000000000000, 293.5832628385307999 ) ) ;
#11448=FACE_OUTER_BOUND ( 'NONE', #8596, .T. ) ;
#11451=LINE ( 'NONE', #4530, #9519 ) ;
#11462=ORIENTED_EDGE ( 'NONE', *, *, #12123, .F. ) ;
#11466=ORIENTED_EDGE ( 'NONE', *, *, #14377, .F. ) ;
#11469=EDGE_CURVE ( 'NONE', #4599, #11965, #5944, .T. ) ;
#11470=AXIS2_PLACEMENT_3D ( 'NONE', #11716, #3951, #7131 ) ;
#11473=CIRCLE ( 'NONE', #13751, 12.50000000000006750 ) ;
#11476=VERTEX_POINT ( 'NONE', #19941 ) ;
#11479=EDGE_CURVE ( 'NONE', #1034, #14947, #11757, .T. ) ;
#11480=CARTESIAN_POINT ( 'NONE',  ( 18.28503710798548454, -57.92514141135459482, 293.5832628385307999 ) ) ;
#11484=FACE_OUTER_BOUND ( 'NONE', #7879, .T. ) ;
#11486=ADVANCED_FACE ( 'NONE', ( #11849 ), #12158, .T. ) ;
#11487=DIRECTION ( 'NONE',  ( 1.000000000000000000, -0.000000000000000000, -0.000000000000000000 ) ) ;
#11488=ORIENTED_EDGE ( 'NONE', *, *, #11419, .F. ) ;
#11489=ORIENTED_EDGE ( 'NONE', *, *, #12737, .T. ) ;
#11498=LINE ( 'NONE', #2205, #5858 ) ;
#11501=CARTESIAN_POINT ( 'NONE',  ( -1.379293853801755176, 58.69016442926522359, 112.7772637782949943 ) ) ;
#11502=FACE_OUTER_BOUND ( 'NONE', #7196, .T. ) ;
#11503=AXIS2_PLACEMENT_3D ( 'NONE', #19191, #10992, #17562 ) ;
#11504=ADVANCED_FACE ( 'NONE', ( #15232 ), #1221, .F. ) ;
#11506=CARTESIAN_POINT ( 'NONE',  ( -31.77187437101504486, -51.77076963420836364, 283.5832628385307999 ) ) ;
#11510=ORIENTED_EDGE ( 'NONE', *, *, #247, .F. ) ;
#11520=PLANE ( 'NONE',  #12321 ) ;
#11528=EDGE_CURVE ( 'NONE', #15281, #16710, #10322, .T. ) ;
#11534=LINE ( 'NONE', #19511, #11949 ) ;
#11535=EDGE_CURVE ( 'NONE', #3199, #1414, #18939, .T. ) ;
#11536=VERTEX_POINT ( 'NONE', #3374 ) ;
#11539=VERTEX_POINT ( 'NONE', #6046 ) ;
#11540=VECTOR ( 'NONE', #11210, 1000.000000000000114 ) ;
#11541=EDGE_LOOP ( 'NONE', ( #8445, #4997, #19607 ) ) ;
#11544=ORIENTED_EDGE ( 'NONE', *, *, #13641, .F. ) ;
#11545=DIRECTION ( 'NONE',  ( -0.9902903945359624593, -0.1390141521205945918, 0.000000000000000000 ) ) ;
#11549=DIRECTION ( 'NONE',  ( 1.000000000000000000, 0.000000000000000000, 0.000000000000000000 ) ) ;
#11552=DIRECTION ( 'NONE',  ( 1.047444401652940164E-14, -1.000000000000000000, 0.000000000000000000 ) ) ;
#11554=CARTESIAN_POINT ( 'NONE',  ( 76.92888220842485225, -14.39940464655733976, 132.4711112102474146 ) ) ;
#11555=LINE ( 'NONE', #7057, #10584 ) ;
#11557=PLANE ( 'NONE',  #13135 ) ;
#11558=CARTESIAN_POINT ( 'NONE',  ( -73.82206860051547892, -25.99419088092166774, 248.9926560891072143 ) ) ;
#11562=EDGE_LOOP ( 'NONE', ( #13091, #19261, #17573, #11942 ) ) ;
#11563=DIRECTION ( 'NONE',  ( 0.000000000000000000, 0.000000000000000000, 1.000000000000000000 ) ) ;
#11566=ORIENTED_EDGE ( 'NONE', *, *, #18004, .F. ) ;
#11567=VERTEX_POINT ( 'NONE', #17399 ) ;
#11568=AXIS2_PLACEMENT_3D ( 'NONE', #16295, #8205, #5345 ) ;
#11569=ORIENTED_EDGE ( 'NONE', *, *, #11397, .F. ) ;
#11571=DIRECTION ( 'NONE',  ( -0.8660254037844344888, -0.5000000000000069944, 0.000000000000000000 ) ) ;
#11573=VERTEX_POINT ( 'NONE', #9410 ) ;
#11574=CARTESIAN_POINT ( 'NONE',  ( -7.948651060879021735, 60.22029172860445101, 293.5832628385307999 ) ) ;
#11577=EDGE_LOOP ( 'NONE', ( #13825, #11363, #18805 ) ) ;
#11578=LINE ( 'NONE', #19460, #4253 ) ;
#11579=CARTESIAN_POINT ( 'NONE',  ( -77.21438937758510690, -12.78021302872823384, 132.4711112102474146 ) ) ;
#11581=VECTOR ( 'NONE', #12377, 1000.000000000000000 ) ;
#11582=LINE ( 'NONE', #13200, #978 ) ;
#11585=ADVANCED_FACE ( 'NONE', ( #99 ), #1731, .T. ) ;
#11587=DIRECTION ( 'NONE',  ( -0.9993852124581887875, 0.03505990758545545621, 0.000000000000000000 ) ) ;
#11588=AXIS2_PLACEMENT_3D ( 'NONE', #20052, #1120, #924 ) ;
#11590=EDGE_CURVE ( 'NONE', #7769, #13278, #14371, .T. ) ;
#11592=VECTOR ( 'NONE', #15117, 1000.000000000000114 ) ;
#11594=DIRECTION ( 'NONE',  ( 0.000000000000000000, 0.000000000000000000, -1.000000000000000000 ) ) ;
#11595=LINE ( 'NONE', #658, #7448 ) ;
#11596=DIRECTION ( 'NONE',  ( 0.1736481776669404620, -0.9848077530122062440, 0.000000000000000000 ) ) ;
#11601=CIRCLE ( 'NONE', #13225, 62.91752772691707207 ) ;
#11602=CARTESIAN_POINT ( 'NONE',  ( 38.41834839689379777, -68.18670162478818497, 110.9660488491356887 ) ) ;
#11604=ORIENTED_EDGE ( 'NONE', *, *, #4334, .T. ) ;
#11606=ORIENTED_EDGE ( 'NONE', *, *, #9559, .T. ) ;
#11609=CARTESIAN_POINT ( 'NONE',  ( 8.939227532413712041, -60.08331549348429235, 293.5832628385307999 ) ) ;
#11611=ORIENTED_EDGE ( 'NONE', *, *, #6486, .T. ) ;
#11612=VECTOR ( 'NONE', #4171, 1000.000000000000000 ) ;
#11614=LINE ( 'NONE', #8346, #16450 ) ;
#11615=FACE_OUTER_BOUND ( 'NONE', #14100, .T. ) ;
#11617=ORIENTED_EDGE ( 'NONE', *, *, #13698, .F. ) ;
#11618=CARTESIAN_POINT ( 'NONE',  ( 0.000000000000000000, 0.000000000000000000, 293.5832628385307999 ) ) ;
#11619=CARTESIAN_POINT ( 'NONE',  ( 18.28503710798548099, -57.92514141135459482, 283.5832628385307999 ) ) ;
#11620=VERTEX_POINT ( 'NONE', #13801 ) ;
#11621=DIRECTION ( 'NONE',  ( -0.7660444431189771253, -0.6427876096865404731, 0.000000000000000000 ) ) ;
#11622=CARTESIAN_POINT ( 'NONE',  ( 58.83691981461632992, -22.28973221005101024, 293.5832628385307999 ) ) ;
#11624=CARTESIAN_POINT ( 'NONE',  ( 0.000000000000000000, 0.000000000000000000, 248.9926560891072143 ) ) ;
#11625=AXIS2_PLACEMENT_3D ( 'NONE', #11618, #872, #16538 ) ;
#11628=CARTESIAN_POINT ( 'NONE',  ( 76.83212392882491315, 14.94814811854986658, 112.0427633081291816 ) ) ;
#11629=FACE_OUTER_BOUND ( 'NONE', #15920, .T. ) ;
#11630=EDGE_LOOP ( 'NONE', ( #17645, #5342, #17311, #5682 ) ) ;
#11632=VERTEX_POINT ( 'NONE', #15444 ) ;
#11633=ORIENTED_EDGE ( 'NONE', *, *, #15285, .T. ) ;
#11635=ORIENTED_EDGE ( 'NONE', *, *, #1789, .T. ) ;
#11636=EDGE_CURVE ( 'NONE', #15281, #18849, #1434, .T. ) ;
#11637=VECTOR ( 'NONE', #2230, 1000.000000000000000 ) ;
#11638=EDGE_CURVE ( 'NONE', #9538, #14807, #6147, .T. ) ;
#11644=ORIENTED_EDGE ( 'NONE', *, *, #13878, .F. ) ;
#11645=VECTOR ( 'NONE', #11414, 1000.000000000000000 ) ;
#11646=DIRECTION ( 'NONE',  ( 0.3420201433256663259, 0.9396926207859093161, 0.000000000000000000 ) ) ;
#11648=FACE_OUTER_BOUND ( 'NONE', #16191, .T. ) ;
#11650=PLANE ( 'NONE',  #5651 ) ;
#11654=CARTESIAN_POINT ( 'NONE',  ( 58.69016442926523069, -0.8220851292429179891, 112.7772637782949516 ) ) ;
#11660=ORIENTED_EDGE ( 'NONE', *, *, #10003, .T. ) ;
#11662=AXIS2_PLACEMENT_3D ( 'NONE', #7300, #4232, #16715 ) ;
#11663=EDGE_CURVE ( 'NONE', #11539, #9195, #9810, .T. ) ;
#11665=CARTESIAN_POINT ( 'NONE',  ( -21.36933070621726571, 54.67896814532662830, 111.4180192758973931 ) ) ;
#11666=VERTEX_POINT ( 'NONE', #5219 ) ;
#11670=EDGE_CURVE ( 'NONE', #19563, #10038, #14617, .T. ) ;
#11671=AXIS2_PLACEMENT_3D ( 'NONE', #3349, #5098, #9388 ) ;
#11677=LINE ( 'NONE', #4001, #19568 ) ;
#11681=CARTESIAN_POINT ( 'NONE',  ( 60.72279549541555355, -1.629937663769388090, 283.5832628385307999 ) ) ;
#11682=EDGE_LOOP ( 'NONE', ( #2838, #3148, #15441 ) ) ;
#11687=DIRECTION ( 'NONE',  ( 1.000000000000000000, 0.000000000000000000, -0.000000000000000000 ) ) ;
#11688=CARTESIAN_POINT ( 'NONE',  ( 45.46865632508072963, -40.28046525994365368, 293.5832628385307999 ) ) ;
#11689=DIRECTION ( 'NONE',  ( -3.491481338843133355E-15, 1.000000000000000000, 0.000000000000000000 ) ) ;
#11690=ORIENTED_EDGE ( 'NONE', *, *, #2497, .T. ) ;
#11691=DIRECTION ( 'NONE',  ( -0.6427876096865481337, 0.7660444431189707970, 0.000000000000000000 ) ) ;
#11694=DIRECTION ( 'NONE',  ( 1.000000000000000000, 0.000000000000000000, 0.000000000000000000 ) ) ;
#11695=DIRECTION ( 'NONE',  ( -0.5000000000000069944, 0.8660254037844345998, 0.000000000000000000 ) ) ;
#11696=VECTOR ( 'NONE', #2561, 1000.000000000000000 ) ;
#11697=VERTEX_POINT ( 'NONE', #6846 ) ;
#11699=ORIENTED_EDGE ( 'NONE', *, *, #4359, .T. ) ;
#11700=ORIENTED_EDGE ( 'NONE', *, *, #13848, .F. ) ;
#11702=ORIENTED_EDGE ( 'NONE', *, *, #17799, .T. ) ;
#11703=AXIS2_PLACEMENT_3D ( 'NONE', #11332, #17588, #14602 ) ;
#11705=DIRECTION ( 'NONE',  ( 1.000000000000000000, 0.000000000000000000, 0.000000000000000000 ) ) ;
#11706=AXIS2_PLACEMENT_3D ( 'NONE', #7028, #11621, #10095 ) ;
#11709=ORIENTED_EDGE ( 'NONE', *, *, #9766, .T. ) ;
#11711=DIRECTION ( 'NONE',  ( 0.000000000000000000, 0.000000000000000000, 1.000000000000000000 ) ) ;
#11715=FACE_OUTER_BOUND ( 'NONE', #1785, .T. ) ;
#11716=CARTESIAN_POINT ( 'NONE',  ( 67.36461649554532016, -39.84224160888924615, 110.9660488491357455 ) ) ;
#11717=VECTOR ( 'NONE', #14658, 1000.000000000000227 ) ;
#11721=PLANE ( 'NONE',  #2835 ) ;
#11725=EDGE_CURVE ( 'NONE', #5887, #4216, #16164, .T. ) ;
#11726=DIRECTION ( 'NONE',  ( 0.2080686897406943681, 0.9781142164131909622, 0.000000000000000000 ) ) ;
#11727=ORIENTED_EDGE ( 'NONE', *, *, #15789, .T. ) ;
#11728=EDGE_LOOP ( 'NONE', ( #19858, #5069, #14516 ) ) ;
#11732=FACE_OUTER_BOUND ( 'NONE', #16209, .T. ) ;
#11733=DIRECTION ( 'NONE',  ( 0.000000000000000000, 0.000000000000000000, 1.000000000000000000 ) ) ;
#11737=CIRCLE ( 'NONE', #16983, 62.91752772691707207 ) ;
#11738=ORIENTED_EDGE ( 'NONE', *, *, #14526, .F. ) ;
#11739=CARTESIAN_POINT ( 'NONE',  ( 0.000000000000000000, 0.000000000000000000, 283.5832628385307999 ) ) ;
#11742=DIRECTION ( 'NONE',  ( -0.000000000000000000, -0.000000000000000000, 1.000000000000000000 ) ) ;
#11744=DIRECTION ( 'NONE',  ( -0.9271237148521547233, 0.3747554100459928872, 0.000000000000000000 ) ) ;
#11745=ADVANCED_FACE ( 'NONE', ( #15957 ), #17703, .T. ) ;
#11746=CYLINDRICAL_SURFACE ( 'NONE', #1978, 60.74260934110282051 ) ;
#11751=CARTESIAN_POINT ( 'NONE',  ( 28.06680738835026290, -53.87178215532764369, 293.5832628385307999 ) ) ;
#11753=EDGE_LOOP ( 'NONE', ( #7144, #2867, #4920 ) ) ;
#11757=LINE ( 'NONE', #5631, #15678 ) ;
#11758=ADVANCED_FACE ( 'NONE', ( #8068 ), #17500, .F. ) ;
#11759=LINE ( 'NONE', #5737, #16560 ) ;
#11760=ORIENTED_EDGE ( 'NONE', *, *, #14480, .F. ) ;
#11764=DIRECTION ( 'NONE',  ( 0.8660254037844380415, 0.5000000000000009992, 0.000000000000000000 ) ) ;
#11770=ORIENTED_EDGE ( 'NONE', *, *, #4787, .T. ) ;
#11775=ORIENTED_EDGE ( 'NONE', *, *, #8019, .T. ) ;
#11777=AXIS2_PLACEMENT_3D ( 'NONE', #4645, #13942, #2701 ) ;
#11780=ORIENTED_EDGE ( 'NONE', *, *, #1653, .T. ) ;
#11785=PLANE ( 'NONE',  #10767 ) ;
#11790=CARTESIAN_POINT ( 'NONE',  ( 0.000000000000000000, 0.000000000000000000, 132.4711112102474146 ) ) ;
#11791=AXIS2_PLACEMENT_3D ( 'NONE', #5162, #15797, #1876 ) ;
#11792=LINE ( 'NONE', #18054, #6456 ) ;
#11799=CARTESIAN_POINT ( 'NONE',  ( -49.07263256785926586, 39.37628763770471352, 248.9926560891072143 ) ) ;
#11800=CARTESIAN_POINT ( 'NONE',  ( -51.77076963420847022, 31.77187437101487077, 283.5832628385307999 ) ) ;
#11801=ORIENTED_EDGE ( 'NONE', *, *, #4132, .F. ) ;
#11802=VECTOR ( 'NONE', #8633, 1000.000000000000000 ) ;
#11805=ORIENTED_EDGE ( 'NONE', *, *, #12464, .T. ) ;
#11806=DIRECTION ( 'NONE',  ( 0.9396926207859058744, 0.3420201433256757628, 0.000000000000000000 ) ) ;
#11811=DIRECTION ( 'NONE',  ( 0.9993852124581887875, -0.03505990758545544927, 0.000000000000000000 ) ) ;
#11812=ORIENTED_EDGE ( 'NONE', *, *, #17554, .T. ) ;
#11814=LINE ( 'NONE', #11441, #5351 ) ;
#11816=AXIS2_PLACEMENT_3D ( 'NONE', #9622, #14226, #15765 ) ;
#11817=EDGE_LOOP ( 'NONE', ( #7627, #16927, #1267, #18561 ) ) ;
#11821=ORIENTED_EDGE ( 'NONE', *, *, #11469, .T. ) ;
#11822=VECTOR ( 'NONE', #16691, 1000.000000000000000 ) ;
#11823=DIRECTION ( 'NONE',  ( -0.000000000000000000, -0.000000000000000000, 1.000000000000000000 ) ) ;
#11824=EDGE_CURVE ( 'NONE', #9575, #14755, #5119, .T. ) ;
#11830=CARTESIAN_POINT ( 'NONE',  ( 18.28567271940513450, -57.92709869106715814, 283.5832628385307999 ) ) ;
#11834=PLANE ( 'NONE',  #7522 ) ;
#11836=ORIENTED_EDGE ( 'NONE', *, *, #18417, .F. ) ;
#11837=DIRECTION ( 'NONE',  ( 1.000000000000000000, 0.000000000000000000, 0.000000000000000000 ) ) ;
#11838=VECTOR ( 'NONE', #8472, 1000.000000000000000 ) ;
#11839=CARTESIAN_POINT ( 'NONE',  ( -58.83691981461618781, 22.28973221005139749, 293.5832628385307999 ) ) ;
#11841=ORIENTED_EDGE ( 'NONE', *, *, #401, .T. ) ;
#11842=EDGE_CURVE ( 'NONE', #18228, #14365, #16461, .T. ) ;
#11843=DIRECTION ( 'NONE',  ( 0.1390141521205946196, -0.9902903945359624593, 0.000000000000000000 ) ) ;
#11846=EDGE_LOOP ( 'NONE', ( #14010, #13798, #8606 ) ) ;
#11849=FACE_OUTER_BOUND ( 'NONE', #14281, .T. ) ;
#11850=EDGE_CURVE ( 'NONE', #14775, #5152, #15012, .T. ) ;
#11851=PLANE ( 'NONE',  #11330 ) ;
#11852=VERTEX_POINT ( 'NONE', #15205 ) ;
#11853=EDGE_CURVE ( 'NONE', #19783, #14388, #2441, .T. ) ;
#11858=DIRECTION ( 'NONE',  ( -0.000000000000000000, -0.000000000000000000, 1.000000000000000000 ) ) ;
#11862=ORIENTED_EDGE ( 'NONE', *, *, #12464, .F. ) ;
#11865=CARTESIAN_POINT ( 'NONE',  ( 1.289614712049185874, -5.590028426173808462, 293.5832628385307999 ) ) ;
#11867=VECTOR ( 'NONE', #8705, 1000.000000000000000 ) ;
#11869=CIRCLE ( 'NONE', #8934, 60.74260934110282051 ) ;
#11870=ORIENTED_EDGE ( 'NONE', *, *, #11164, .T. ) ;
#11871=DIRECTION ( 'NONE',  ( -0.000000000000000000, -1.000000000000000000, -0.000000000000000000 ) ) ;
#11872=ORIENTED_EDGE ( 'NONE', *, *, #10904, .T. ) ;
#11875=EDGE_CURVE ( 'NONE', #12652, #18954, #1190, .T. ) ;
#11879=ADVANCED_FACE ( 'NONE', ( #11732 ), #13563, .F. ) ;
#11880=LINE ( 'NONE', #15164, #5930 ) ;
#11884=ORIENTED_EDGE ( 'NONE', *, *, #7900, .F. ) ;
#11887=VECTOR ( 'NONE', #14169, 1000.000000000000000 ) ;
#11889=LINE ( 'NONE', #10074, #12323 ) ;
#11892=EDGE_CURVE ( 'NONE', #10368, #6110, #16617, .T. ) ;
#11895=ORIENTED_EDGE ( 'NONE', *, *, #15760, .T. ) ;
#11896=AXIS2_PLACEMENT_3D ( 'NONE', #12663, #11335, #15641 ) ;
#11899=ADVANCED_FACE ( 'NONE', ( #13460 ), #2743, .F. ) ;
#11902=DIRECTION ( 'NONE',  ( -0.000000000000000000, -0.000000000000000000, 1.000000000000000000 ) ) ;
#11903=ORIENTED_EDGE ( 'NONE', *, *, #4921, .T. ) ;
#11905=DIRECTION ( 'NONE',  ( -0.3420201433256630508, -0.9396926207859104263, 0.000000000000000000 ) ) ;
#11908=ORIENTED_EDGE ( 'NONE', *, *, #14125, .T. ) ;
#11910=DIRECTION ( 'NONE',  ( 1.000000000000000000, 0.000000000000000000, 0.000000000000000000 ) ) ;
#11915=CARTESIAN_POINT ( 'NONE',  ( 49.24833719034187851, 60.83768308848395634, 110.7293897666001214 ) ) ;
#11919=CARTESIAN_POINT ( 'NONE',  ( -58.03804081968160489, 8.833100819208169696, 132.4711112102474146 ) ) ;
#11921=VERTEX_POINT ( 'NONE', #16655 ) ;
#11926=DIRECTION ( 'NONE',  ( -0.9848077530122073542, -0.1736481776669340227, 0.000000000000000000 ) ) ;
#11930=CYLINDRICAL_SURFACE ( 'NONE', #17609, 60.74260934110282051 ) ;
#11931=FACE_OUTER_BOUND ( 'NONE', #1637, .T. ) ;
#11933=DIRECTION ( 'NONE',  ( -0.9396926207859068736, -0.3420201433256725987, 0.000000000000000000 ) ) ;
#11937=CARTESIAN_POINT ( 'NONE',  ( -76.92888220842476699, 14.39940464655786201, 112.0427633081292385 ) ) ;
#11939=EDGE_CURVE ( 'NONE', #13503, #8985, #19916, .T. ) ;
#11941=DIRECTION ( 'NONE',  ( -0.6427876096865456912, 0.7660444431189725734, -0.000000000000000000 ) ) ;
#11942=ORIENTED_EDGE ( 'NONE', *, *, #13485, .T. ) ;
#11944=VERTEX_POINT ( 'NONE', #10204 ) ;
#11949=VECTOR ( 'NONE', #8756, 999.9999999999998863 ) ;
#11950=CARTESIAN_POINT ( 'NONE',  ( 0.000000000000000000, 0.000000000000000000, 293.5832628385307999 ) ) ;
#11954=EDGE_CURVE ( 'NONE', #5657, #19395, #8672, .T. ) ;
#11955=ADVANCED_FACE ( 'NONE', ( #19617 ), #18598, .T. ) ;
#11956=AXIS2_PLACEMENT_3D ( 'NONE', #5715, #6949, #16468 ) ;
#11958=DIRECTION ( 'NONE',  ( 0.3088643371590125142, -0.9511061040868803440, 0.000000000000000000 ) ) ;
#11960=VECTOR ( 'NONE', #5438, 1000.000000000000114 ) ;
#11961=CARTESIAN_POINT ( 'NONE',  ( -44.43084819159250287, 38.35506425062501989, 110.7293897666001214 ) ) ;
#11962=DIRECTION ( 'NONE',  ( -0.2080686897406943958, -0.9781142164131909622, 0.000000000000000000 ) ) ;
#11963=DIRECTION ( 'NONE',  ( -0.6427876096865405842, 0.7660444431189771253, 0.000000000000000000 ) ) ;
#11964=CARTESIAN_POINT ( 'NONE',  ( -19.23614321207234923, 57.61627707419557254, 283.5832628385307999 ) ) ;
#11965=VERTEX_POINT ( 'NONE', #12443 ) ;
#11969=CARTESIAN_POINT ( 'NONE',  ( 57.61823435390807902, 19.23677882349220880, 293.5832628385307999 ) ) ;
#11974=( NAMED_UNIT ( * ) PLANE_ANGLE_UNIT ( ) SI_UNIT ( $, .RADIAN. ) );
#11976=CARTESIAN_POINT ( 'NONE',  ( -49.67518383744793908, 60.47951622432801599, 110.7293897666001214 ) ) ;
#11977=ORIENTED_EDGE ( 'NONE', *, *, #508, .T. ) ;
#11984=DIRECTION ( 'NONE',  ( -0.9848077530122062440, -0.1736481776669404620, 0.000000000000000000 ) ) ;
#11985=VERTEX_POINT ( 'NONE', #17170 ) ;
#11986=DIRECTION ( 'NONE',  ( 0.000000000000000000, -1.000000000000000000, 0.000000000000000000 ) ) ;
#11989=CARTESIAN_POINT ( 'NONE',  ( 0.000000000000000000, 0.000000000000000000, 0.000000000000000000 ) ) ;
#11990=PLANE ( 'NONE',  #9727 ) ;
#11993=CARTESIAN_POINT ( 'NONE',  ( -74.01264520835137262, 25.47058595421627913, 132.4711112102474146 ) ) ;
#11994=EDGE_CURVE ( 'NONE', #15923, #12841, #18924, .T. ) ;
#11995=AXIS2_PLACEMENT_3D ( 'NONE', #13565, #5812, #12031 ) ;
#11997=EDGE_CURVE ( 'NONE', #17740, #16088, #15524, .T. ) ;
#11999=ORIENTED_EDGE ( 'NONE', *, *, #8638, .T. ) ;
#12000=ORIENTED_EDGE ( 'NONE', *, *, #12516, .T. ) ;
#12001=ORIENTED_EDGE ( 'NONE', *, *, #11250, .F. ) ;
#12002=VERTEX_POINT ( 'NONE', #7740 ) ;
#12004=ADVANCED_FACE ( 'NONE', ( #20018 ), #12649, .T. ) ;
#12005=CARTESIAN_POINT ( 'NONE',  ( -32.16802499836779106, -54.07248341783242296, 132.4711112102474146 ) ) ;
#12006=DIRECTION ( 'NONE',  ( -0.000000000000000000, -0.000000000000000000, 1.000000000000000000 ) ) ;
#12009=DIRECTION ( 'NONE',  ( 1.000000000000000000, 0.000000000000000000, 0.000000000000000000 ) ) ;
#12012=DIRECTION ( 'NONE',  ( -0.6692498792541753394, -0.7430374143461900838, 0.000000000000000000 ) ) ;
#12014=DIRECTION ( 'NONE',  ( -0.000000000000000000, -0.000000000000000000, 1.000000000000000000 ) ) ;
#12018=LINE ( 'NONE', #16548, #15955 ) ;
#12022=AXIS2_PLACEMENT_3D ( 'NONE', #7841, #4687, #20119 ) ;
#12029=ORIENTED_EDGE ( 'NONE', *, *, #16350, .T. ) ;
#12031=DIRECTION ( 'NONE',  ( 1.000000000000000000, 0.000000000000000000, 0.000000000000000000 ) ) ;
#12033=CARTESIAN_POINT ( 'NONE',  ( -62.90240729679781850, -1.379293853801974779, 132.4711112102474146 ) ) ;
#12036=DIRECTION ( 'NONE',  ( 1.000000000000000000, 0.000000000000000000, 0.000000000000000000 ) ) ;
#12041=ORIENTED_EDGE ( 'NONE', *, *, #2613, .F. ) ;
#12044=FACE_OUTER_BOUND ( 'NONE', #118, .T. ) ;
#12045=VERTEX_POINT ( 'NONE', #15420 ) ;
#12047=CARTESIAN_POINT ( 'NONE',  ( 0.000000000000000000, 0.000000000000000000, 283.5832628385307999 ) ) ;
#12048=ORIENTED_EDGE ( 'NONE', *, *, #20022, .T. ) ;
#12049=ORIENTED_EDGE ( 'NONE', *, *, #12363, .T. ) ;
#12051=ORIENTED_EDGE ( 'NONE', *, *, #18427, .F. ) ;
#12052=VECTOR ( 'NONE', #19192, 1000.000000000000000 ) ;
#12053=VECTOR ( 'NONE', #8553, 1000.000000000000114 ) ;
#12054=LINE ( 'NONE', #13699, #7818 ) ;
#12055=DIRECTION ( 'NONE',  ( -0.6427876096865456912, 0.7660444431189726844, 0.000000000000000000 ) ) ;
#12056=ORIENTED_EDGE ( 'NONE', *, *, #13598, .T. ) ;
#12059=DIRECTION ( 'NONE',  ( -0.4999999999999888978, -0.8660254037844449249, 0.000000000000000000 ) ) ;
#12060=PLANE ( 'NONE',  #6582 ) ;
#12061=CARTESIAN_POINT ( 'NONE',  ( 4.196299268919053915, 3.911853314815666671, 283.5832628385307999 ) ) ;
#12067=CARTESIAN_POINT ( 'NONE',  ( -27.53920554013687649, -73.25972925305620720, 132.4711112102474146 ) ) ;
#12070=EDGE_CURVE ( 'NONE', #14186, #10466, #10596, .T. ) ;
#12072=( LENGTH_UNIT ( ) NAMED_UNIT ( * ) SI_UNIT ( .MILLI., .METRE. ) );
#12074=FACE_BOUND ( 'NONE', #13068, .T. ) ;
#12077=VECTOR ( 'NONE', #2904, 1000.000000000000000 ) ;
#12078=PLANE ( 'NONE',  #9241 ) ;
#12079=LINE ( 'NONE', #3409, #5029 ) ;
#12081=EDGE_CURVE ( 'NONE', #10931, #13585, #16851, .T. ) ;
#12083=EDGE_CURVE ( 'NONE', #4164, #347, #6120, .T. ) ;
#12084=CARTESIAN_POINT ( 'NONE',  ( -19.30071112029641967, 55.43188410062188609, 248.9926560891072143 ) ) ;
#12086=EDGE_CURVE ( 'NONE', #1114, #17034, #15474, .T. ) ;
#12087=DIRECTION ( 'NONE',  ( -0.000000000000000000, -0.000000000000000000, 1.000000000000000000 ) ) ;
#12090=CARTESIAN_POINT ( 'NONE',  ( -30.25670013172253192, -55.16472960512360402, 293.5832628385307999 ) ) ;
#12091=DIRECTION ( 'NONE',  ( 0.1390141521205912056, -0.9902903945359629034, 0.000000000000000000 ) ) ;
#12093=VERTEX_POINT ( 'NONE', #13828 ) ;
#12094=AXIS2_PLACEMENT_3D ( 'NONE', #10430, #12168, #16888 ) ;
#12096=CONICAL_SURFACE ( 'NONE', #17360, 17.50000000000001066, 0.7853981633974479459 ) ;
#12098=VERTEX_POINT ( 'NONE', #16705 ) ;
#12099=ORIENTED_EDGE ( 'NONE', *, *, #430, .F. ) ;
#12100=ORIENTED_EDGE ( 'NONE', *, *, #14549, .T. ) ;
#12104=LINE ( 'NONE', #18161, #475 ) ;
#12105=EDGE_CURVE ( 'NONE', #13503, #1969, #4115, .T. ) ;
#12106=CARTESIAN_POINT ( 'NONE',  ( -79.75827554147308263, 9.767571684737763671E-15, 293.5832628385307999 ) ) ;
#12111=LINE ( 'NONE', #18370, #12053 ) ;
#12113=ORIENTED_EDGE ( 'NONE', *, *, #14110, .T. ) ;
#12115=CARTESIAN_POINT ( 'NONE',  ( 23.22641211976289100, 56.12662799072080588, 283.5832628385307999 ) ) ;
#12121=ORIENTED_EDGE ( 'NONE', *, *, #3755, .T. ) ;
#12122=VERTEX_POINT ( 'NONE', #4218 ) ;
#12123=EDGE_CURVE ( 'NONE', #9378, #8067, #9125, .T. ) ;
#12124=CARTESIAN_POINT ( 'NONE',  ( 45.46712722958809394, -40.27908801170008246, 293.5832628385307999 ) ) ;
#12125=EDGE_LOOP ( 'NONE', ( #19808, #16308, #9780, #9840 ) ) ;
#12126=ORIENTED_EDGE ( 'NONE', *, *, #14997, .T. ) ;
#12130=DIRECTION ( 'NONE',  ( 0.000000000000000000, 0.000000000000000000, 1.000000000000000000 ) ) ;
#12132=DIRECTION ( 'NONE',  ( 0.000000000000000000, 0.000000000000000000, 1.000000000000000000 ) ) ;
#12133=ORIENTED_EDGE ( 'NONE', *, *, #13591, .T. ) ;
#12134=EDGE_CURVE ( 'NONE', #18587, #15066, #4424, .T. ) ;
#12139=VERTEX_POINT ( 'NONE', #18600 ) ;
#12140=DIRECTION ( 'NONE',  ( -0.7881095627315599650, -0.6155349844899714595, 0.000000000000000000 ) ) ;
#12142=DIRECTION ( 'NONE',  ( -0.7660444431189813441, 0.6427876096865353661, 0.000000000000000000 ) ) ;
#12143=ORIENTED_EDGE ( 'NONE', *, *, #17181, .F. ) ;
#12146=LINE ( 'NONE', #18406, #16908 ) ;
#12152=ORIENTED_EDGE ( 'NONE', *, *, #5127, .F. ) ;
#12153=AXIS2_PLACEMENT_3D ( 'NONE', #8981, #14099, #10717 ) ;
#12158=PLANE ( 'NONE',  #18280 ) ;
#12159=CARTESIAN_POINT ( 'NONE',  ( 60.68773558783009747, -2.629322876227576433, 293.5832628385307999 ) ) ;
#12160=CIRCLE ( 'NONE', #17427, 62.91752772691707207 ) ;
#12164=CARTESIAN_POINT ( 'NONE',  ( 53.40063514825077107, 28.94886449118924432, 283.5832628385307999 ) ) ;
#12166=EDGE_CURVE ( 'NONE', #19334, #9872, #17584, .T. ) ;
#12167=LINE ( 'NONE', #2775, #7846 ) ;
#12168=DIRECTION ( 'NONE',  ( 0.000000000000000000, 0.000000000000000000, 1.000000000000000000 ) ) ;
#12171=DIRECTION ( 'NONE',  ( -0.000000000000000000, -0.000000000000000000, 1.000000000000000000 ) ) ;
#12174=VERTEX_POINT ( 'NONE', #19815 ) ;
#12175=CARTESIAN_POINT ( 'NONE',  ( -1.629937663769596368, -60.72279549541552512, 293.5832628385307999 ) ) ;
#12176=DIRECTION ( 'NONE',  ( 1.000000000000000000, 0.000000000000000000, 0.000000000000000000 ) ) ;
#12179=ORIENTED_EDGE ( 'NONE', *, *, #8132, .F. ) ;
#12180=VERTEX_POINT ( 'NONE', #6122 ) ;
#12182=ORIENTED_EDGE ( 'NONE', *, *, #18681, .T. ) ;
#12183=FACE_BOUND ( 'NONE', #11577, .T. ) ;
#12185=VERTEX_POINT ( 'NONE', #2646 ) ;
#12186=DIRECTION ( 'NONE',  ( 0.4693298356057531984, -0.8830229359480288309, 0.000000000000000000 ) ) ;
#12188=DIRECTION ( 'NONE',  ( -0.000000000000000000, -0.000000000000000000, 1.000000000000000000 ) ) ;
#12189=LINE ( 'NONE', #13415, #12785 ) ;
#12193=EDGE_CURVE ( 'NONE', #5152, #3741, #10597, .T. ) ;
#12194=ORIENTED_EDGE ( 'NONE', *, *, #11997, .F. ) ;
#12196=CYLINDRICAL_SURFACE ( 'NONE', #8022, 60.74260934110282051 ) ;
#12198=VECTOR ( 'NONE', #9857, 1000.000000000000000 ) ;
#12200=CARTESIAN_POINT ( 'NONE',  ( 60.47951622432751151, 49.67518383744852883, 248.9926560891072143 ) ) ;
#12202=ORIENTED_EDGE ( 'NONE', *, *, #18418, .T. ) ;
#12206=AXIS2_PLACEMENT_3D ( 'NONE', #3188, #18952, #9822 ) ;
#12209=EDGE_LOOP ( 'NONE', ( #9316, #9702, #18912, #13332 ) ) ;
#12212=DIRECTION ( 'NONE',  ( -0.000000000000000000, -0.000000000000000000, 1.000000000000000000 ) ) ;
#12213=CIRCLE ( 'NONE', #11247, 60.74260934110282051 ) ;
#12217=LINE ( 'NONE', #1490, #320 ) ;
#12219=EDGE_LOOP ( 'NONE', ( #4260, #20038, #15939, #9806 ) ) ;
#12221=CARTESIAN_POINT ( 'NONE',  ( -17.50000000000001066, 2.143131898507869431E-15, 83.57543755549745867 ) ) ;
#12223=CARTESIAN_POINT ( 'NONE',  ( 49.07263256785952166, -39.37628763770437956, 293.5832628385307999 ) ) ;
#12224=CARTESIAN_POINT ( 'NONE',  ( 51.77251465595239921, -31.77296517111717478, 293.5832628385307999 ) ) ;
#12225=CIRCLE ( 'NONE', #6043, 60.74260934110282051 ) ;
#12226=CARTESIAN_POINT ( 'NONE',  ( 20.21777810286675958, 59.58067424803633116, 293.5832628385307999 ) ) ;
#12227=ORIENTED_EDGE ( 'NONE', *, *, #6373, .T. ) ;
#12230=FACE_OUTER_BOUND ( 'NONE', #16792, .T. ) ;
#12233=EDGE_CURVE ( 'NONE', #10391, #4654, #7742, .T. ) ;
#12239=CARTESIAN_POINT ( 'NONE',  ( 21.51741588379836756, 55.08582882688782689, 248.9926560891072143 ) ) ;
#12241=CIRCLE ( 'NONE', #8967, 79.75827554147308263 ) ;
#12242=CARTESIAN_POINT ( 'NONE',  ( -2.629322876227788264, -60.68773558783006905, 293.5832628385307999 ) ) ;
#12243=DIRECTION ( 'NONE',  ( 1.000000000000000000, 0.000000000000000000, -0.000000000000000000 ) ) ;
#12244=ORIENTED_EDGE ( 'NONE', *, *, #8393, .T. ) ;
#12245=EDGE_CURVE ( 'NONE', #3122, #15949, #20179, .T. ) ;
#12246=CARTESIAN_POINT ( 'NONE',  ( -23.22718332831480481, -56.12853591711337486, 293.5832628385307999 ) ) ;
#12248=CARTESIAN_POINT ( 'NONE',  ( 21.36933070621763164, -54.67896814532648619, 132.4711112102474146 ) ) ;
#12252=CARTESIAN_POINT ( 'NONE',  ( -4.581103194069770623, 3.453261854572849288, 293.5832628385307999 ) ) ;
#12254=CARTESIAN_POINT ( 'NONE',  ( -50.93469132750304595, -59.42266395395774481, 132.4711112102474146 ) ) ;
#12255=DIRECTION ( 'NONE',  ( 0.3088643371590125142, -0.9511061040868803440, 0.000000000000000000 ) ) ;
#12256=EDGE_LOOP ( 'NONE', ( #15399, #19315, #246, #8911 ) ) ;
#12259=ORIENTED_EDGE ( 'NONE', *, *, #5515, .F. ) ;
#12260=EDGE_CURVE ( 'NONE', #9227, #9534, #13291, .T. ) ;
#12261=PRODUCT_DEFINITION ( 'UNKNOWN', '', #3289, #1518 ) ;
#12262=DIRECTION ( 'NONE',  ( 1.000000000000000000, 0.000000000000000000, 0.000000000000000000 ) ) ;
#12263=ORIENTED_EDGE ( 'NONE', *, *, #19119, .F. ) ;
#12267=EDGE_LOOP ( 'NONE', ( #8957, #3650, #8467, #10294, #13956, #14841, #3398, #17368, #18748, #1453, #2019, #16651, #12315, #15805, #7235, #8062, #596, #16696, #11999, #14951, #413, #2639, #3916, #3989, #14313, #5434, #14991, #17447, #3185, #19472, #11870, #12718, #6607, #5859, #3045, #18873, #8303, #11544, #2511, #9855, #20, #4633, #6372, #12425, #10061, #17077, #17964, #14120, #8447, #15312, #17859, #16073, #1938, #14645, #13652, #19824, #4141, #1556, #8504, #11163, #12924, #2951, #1802, #18142, #19452, #2070, #17260, #19100, #6150, #18448, #5985, #12383, #19753, #802, #16981, #12048, #2463, #1758, #14423, #3647, #13718, #18533, #17529, #18440, #12942, #13555, #4238, #11812, #10513, #17730, #12540, #1528, #12695, #17821, #3020, #8642, #574, #8048, #1211, #12100, #11770, #5851, #11340, #10419, #3400, #8578, #12056, #2399, #8136, #19210, #19986, #1312, #9478, #2451, #12698, #822, #12996, #4280, #15494, #7845, #19203, #16746, #15410, #5123, #4865, #3354, #4984, #5099, #12326, #3918, #11872, #3936, #15654, #1106, #192, #16207, #2407, #9147, #13800, #2608, #10901, #1992, #11136, #16340 ) ) ;
#12268=AXIS2_PLACEMENT_3D ( 'NONE', #19714, #8869, #16268 ) ;
#12270=DIRECTION ( 'NONE',  ( 0.8660254037844363761, 0.5000000000000039968, -0.000000000000000000 ) ) ;
#12272=CARTESIAN_POINT ( 'NONE',  ( -2.605298826210324936, -5.111158570922258448, 293.5832628385307999 ) ) ;
#12275=CARTESIAN_POINT ( 'NONE',  ( 0.000000000000000000, 0.000000000000000000, 293.5832628385307999 ) ) ;
#12280=FACE_OUTER_BOUND ( 'NONE', #4927, .T. ) ;
#12281=FACE_OUTER_BOUND ( 'NONE', #5437, .T. ) ;
#12282=EDGE_CURVE ( 'NONE', #12185, #5313, #10399, .T. ) ;
#12284=VECTOR ( 'NONE', #16254, 1000.000000000000000 ) ;
#12286=ORIENTED_EDGE ( 'NONE', *, *, #4921, .F. ) ;
#12287=ADVANCED_FACE ( 'NONE', ( #15109 ), #1089, .F. ) ;
#12293=AXIS2_PLACEMENT_3D ( 'NONE', #11739, #13571, #7343 ) ;
#12295=CARTESIAN_POINT ( 'NONE',  ( -57.94128254008190027, -9.381844291199545438, 248.9926560891072143 ) ) ;
#12297=LINE ( 'NONE', #12084, #12403 ) ;
#12301=PLANE ( 'NONE',  #9836 ) ;
#12303=VERTEX_POINT ( 'NONE', #4268 ) ;
#12304=DIRECTION ( 'NONE',  ( 1.000000000000000000, 0.000000000000000000, 0.000000000000000000 ) ) ;
#12305=ORIENTED_EDGE ( 'NONE', *, *, #8414, .F. ) ;
#12306=ORIENTED_EDGE ( 'NONE', *, *, #13672, .F. ) ;
#12307=VECTOR ( 'NONE', #12454, 1000.000000000000000 ) ;
#12308=ORIENTED_EDGE ( 'NONE', *, *, #7386, .F. ) ;
#12312=ORIENTED_EDGE ( 'NONE', *, *, #4109, .T. ) ;
#12314=LINE ( 'NONE', #18686, #647 ) ;
#12315=ORIENTED_EDGE ( 'NONE', *, *, #12515, .T. ) ;
#12319=CARTESIAN_POINT ( 'NONE',  ( 25.47058595421554372, 74.01264520835162841, 248.9926560891072143 ) ) ;
#12320=PLANE ( 'NONE',  #2653 ) ;
#12321=AXIS2_PLACEMENT_3D ( 'NONE', #6925, #19209, #2223 ) ;
#12322=AXIS2_PLACEMENT_3D ( 'NONE', #12838, #14948, #7189 ) ;
#12323=VECTOR ( 'NONE', #5469, 1000.000000000000000 ) ;
#12324=DIRECTION ( 'NONE',  ( -0.8660254037844432595, 0.4999999999999919509, 0.000000000000000000 ) ) ;
#12326=ORIENTED_EDGE ( 'NONE', *, *, #13024, .T. ) ;
#12329=ORIENTED_EDGE ( 'NONE', *, *, #12973, .F. ) ;
#12332=ORIENTED_EDGE ( 'NONE', *, *, #19518, .T. ) ;
#12333=LINE ( 'NONE', #4576, #16546 ) ;
#12334=AXIS2_PLACEMENT_3D ( 'NONE', #15809, #1793, #16112 ) ;
#12335=CARTESIAN_POINT ( 'NONE',  ( -28.15057869795625578, -51.51682027493055216, 132.4711112102474146 ) ) ;
#12336=VECTOR ( 'NONE', #4489, 1000.000000000000000 ) ;
#12338=CARTESIAN_POINT ( 'NONE',  ( -50.41613078340781584, 30.05702882063080494, 248.9926560891072143 ) ) ;
#12340=EDGE_CURVE ( 'NONE', #15515, #4038, #17172, .T. ) ;
#12342=CARTESIAN_POINT ( 'NONE',  ( 57.92514141135453087, 18.28503710798568349, 293.5832628385307999 ) ) ;
#12343=ORIENTED_EDGE ( 'NONE', *, *, #13761, .T. ) ;
#12347=DIRECTION ( 'NONE',  ( 0.000000000000000000, 0.000000000000000000, 1.000000000000000000 ) ) ;
#12351=AXIS2_PLACEMENT_3D ( 'NONE', #13070, #16264, #9912 ) ;
#12352=DIRECTION ( 'NONE',  ( -0.5300553768524346454, -0.8479630283625717579, 0.000000000000000000 ) ) ;
#12357=ORIENTED_EDGE ( 'NONE', *, *, #8872, .F. ) ;
#12361=ORIENTED_EDGE ( 'NONE', *, *, #11268, .F. ) ;
#12363=EDGE_CURVE ( 'NONE', #12139, #10138, #3556, .T. ) ;
#12364=CARTESIAN_POINT ( 'NONE',  ( 22.29928840491073672, 56.50138340076680521, 283.5832628385307999 ) ) ;
#12366=CARTESIAN_POINT ( 'NONE',  ( 47.56406379474552182, 37.78325588002191893, 283.5832628385307999 ) ) ;
#12367=DIRECTION ( 'NONE',  ( 1.000000000000000000, 0.000000000000000000, -0.000000000000000000 ) ) ;
#12368=ORIENTED_EDGE ( 'NONE', *, *, #1942, .T. ) ;
#12377=DIRECTION ( 'NONE',  ( 0.000000000000000000, 0.000000000000000000, -1.000000000000000000 ) ) ;
#12378=EDGE_LOOP ( 'NONE', ( #5605, #14613, #18410, #18538 ) ) ;
#12381=FACE_OUTER_BOUND ( 'NONE', #9933, .T. ) ;
#12383=ORIENTED_EDGE ( 'NONE', *, *, #8974, .T. ) ;
#12385=PLANE ( 'NONE',  #6319 ) ;
#12386=ORIENTED_EDGE ( 'NONE', *, *, #11017, .F. ) ;
#12390=EDGE_CURVE ( 'NONE', #7405, #9578, #16586, .T. ) ;
#12394=FACE_OUTER_BOUND ( 'NONE', #537, .T. ) ;
#12397=DIRECTION ( 'NONE',  ( -0.1390141521205912334, 0.9902903945359629034, 0.000000000000000000 ) ) ;
#12401=DIRECTION ( 'NONE',  ( -0.000000000000000000, -0.000000000000000000, 1.000000000000000000 ) ) ;
#12402=CARTESIAN_POINT ( 'NONE',  ( 59.06449708980161972, 51.36153797460926995, 248.9926560891072143 ) ) ;
#12403=VECTOR ( 'NONE', #6184, 999.9999999999998863 ) ;
#12405=CARTESIAN_POINT ( 'NONE',  ( 0.000000000000000000, 0.000000000000000000, 283.5832628385307999 ) ) ;
#12411=EDGE_CURVE ( 'NONE', #6110, #244, #17580, .T. ) ;
#12415=VECTOR ( 'NONE', #4806, 1000.000000000000000 ) ;
#12417=AXIS2_PLACEMENT_3D ( 'NONE', #12405, #18665, #4641 ) ;
#12419=ORIENTED_EDGE ( 'NONE', *, *, #6854, .F. ) ;
#12420=DIRECTION ( 'NONE',  ( -0.000000000000000000, -0.000000000000000000, 1.000000000000000000 ) ) ;
#12422=ORIENTED_EDGE ( 'NONE', *, *, #14367, .F. ) ;
#12425=ORIENTED_EDGE ( 'NONE', *, *, #1243, .T. ) ;
#12429=DIRECTION ( 'NONE',  ( 0.3420201433256790380, -0.9396926207859046531, 0.000000000000000000 ) ) ;
#12430=VECTOR ( 'NONE', #9268, 1000.000000000000227 ) ;
#12431=CARTESIAN_POINT ( 'NONE',  ( 20.21777810286676313, 59.58067424803633827, 248.9926560891072143 ) ) ;
#12434=EDGE_LOOP ( 'NONE', ( #5502, #7849, #3736 ) ) ;
#12435=ORIENTED_EDGE ( 'NONE', *, *, #3621, .T. ) ;
#12436=ORIENTED_EDGE ( 'NONE', *, *, #10120, .F. ) ;
#12438=CARTESIAN_POINT ( 'NONE',  ( 0.000000000000000000, 0.000000000000000000, 293.5832628385307999 ) ) ;
#12441=CARTESIAN_POINT ( 'NONE',  ( -1.629937663769596368, -60.72279549541552512, 293.5832628385307999 ) ) ;
#12443=CARTESIAN_POINT ( 'NONE',  ( 73.82206860051529418, 25.99419088092216867, 248.9926560891072143 ) ) ;
#12445=DIRECTION ( 'NONE',  ( -0.000000000000000000, -0.000000000000000000, 1.000000000000000000 ) ) ;
#12446=ORIENTED_EDGE ( 'NONE', *, *, #13211, .T. ) ;
#12448=DIRECTION ( 'NONE',  ( -0.000000000000000000, -0.000000000000000000, 1.000000000000000000 ) ) ;
#12454=DIRECTION ( 'NONE',  ( -0.9396926207859046531, -0.3420201433256790380, -0.000000000000000000 ) ) ;
#12455=CARTESIAN_POINT ( 'NONE',  ( 39.80940113486020238, -48.72193424476462553, 293.5832628385307999 ) ) ;
#12457=ORIENTED_EDGE ( 'NONE', *, *, #19387, .F. ) ;
#12463=EDGE_LOOP ( 'NONE', ( #4548, #11002, #13847, #1833, #3472, #19680, #11416, #14315, #2796, #4037, #716, #6467, #6768, #14859, #4375, #1370, #5485, #991, #18265, #20222, #14584, #12179, #5702, #917, #18367, #8425, #7747, #15857, #3691, #14199, #19036, #2622, #6800, #10643, #6321, #6422, #3287, #13562, #13080, #1473, #8078, #1207, #16557, #10364, #7988, #2148, #18037, #10606, #434, #16255, #13288, #14244, #2144, #6393, #17990, #9192, #6294, #1171, #2610, #17545, #19495, #9066, #13047, #16628, #19807, #12596, #7027, #8862, #16904, #4985, #15602, #16233, #4012, #8315, #6896, #268, #9169, #6169, #2120, #1649, #396, #6941, #12457, #17742, #1137, #2686, #4837, #18333, #1183, #8271, #16698, #10576, #8687, #7788, #13440, #12723, #3696, #6866, #19954, #13386, #17069, #13464, #4500, #17829, #4074, #16216, #9461, #7373, #6424, #12286, #8887, #18356, #19397, #18749, #6796, #591, #468, #7817, #623, #10809, #7991, #15812, #9635, #10555, #1090, #2882, #12041, #18175, #3076, #10119, #8544, #2564, #8954, #6578, #210, #1481, #8792, #11569, #17674, #1350, #1912, #13489, #5781, #19963 ) ) ;
#12464=EDGE_CURVE ( 'NONE', #18654, #17774, #17479, .T. ) ;
#12465=DIRECTION ( 'NONE',  ( -0.000000000000000000, -0.000000000000000000, 1.000000000000000000 ) ) ;
#12468=DIRECTION ( 'NONE',  ( -0.9271237148521547233, 0.3747554100459928872, 0.000000000000000000 ) ) ;
#12469=CARTESIAN_POINT ( 'NONE',  ( -10.11498556985118746, 62.09913334491134407, 132.4711112102474146 ) ) ;
#12471=ADVANCED_FACE ( 'NONE', ( #7946 ), #15835, .F. ) ;
#12472=DIRECTION ( 'NONE',  ( 0.6155349844899715706, -0.7881095627315598540, 0.000000000000000000 ) ) ;
#12473=DIRECTION ( 'NONE',  ( -0.3420201433256790380, 0.9396926207859046531, 0.000000000000000000 ) ) ;
#12476=FACE_OUTER_BOUND ( 'NONE', #11429, .T. ) ;
#12477=CARTESIAN_POINT ( 'NONE',  ( 60.83768308848377160, -49.24833719034207036, 110.7293897666001214 ) ) ;
#12480=PLANE ( 'NONE',  #1567 ) ;
#12481=CARTESIAN_POINT ( 'NONE',  ( -49.24833719034228352, -60.83768308848358686, 132.4711112102474146 ) ) ;
#12486=AXIS2_PLACEMENT_3D ( 'NONE', #17448, #9653, #3421 ) ;
#12489=ORIENTED_EDGE ( 'NONE', *, *, #4686, .T. ) ;
#12490=EDGE_CURVE ( 'NONE', #4348, #9722, #4830, .T. ) ;
#12492=FACE_BOUND ( 'NONE', #1895, .T. ) ;
#12493=ORIENTED_EDGE ( 'NONE', *, *, #1880, .F. ) ;
#12494=VECTOR ( 'NONE', #7447, 1000.000000000000000 ) ;
#12506=CYLINDRICAL_SURFACE ( 'NONE', #15598, 60.74260934110282051 ) ;
#12511=AXIS2_PLACEMENT_3D ( 'NONE', #17086, #1435, #10936 ) ;
#12513=ADVANCED_FACE ( 'NONE', ( #968 ), #11520, .T. ) ;
#12514=ORIENTED_EDGE ( 'NONE', *, *, #7240, .T. ) ;
#12515=EDGE_CURVE ( 'NONE', #17279, #14612, #2322, .T. ) ;
#12516=EDGE_CURVE ( 'NONE', #8307, #13307, #11381, .T. ) ;
#12519=AXIS2_PLACEMENT_3D ( 'NONE', #12047, #4287, #10512 ) ;
#12521=FACE_OUTER_BOUND ( 'NONE', #6762, .T. ) ;
#12526=LINE ( 'NONE', #18786, #2913 ) ;
#12528=CARTESIAN_POINT ( 'NONE',  ( 0.000000000000000000, 0.000000000000000000, 283.5832628385307999 ) ) ;
#12530=LINE ( 'NONE', #5615, #12430 ) ;
#12532=ORIENTED_EDGE ( 'NONE', *, *, #2845, .T. ) ;
#12534=CARTESIAN_POINT ( 'NONE',  ( 0.000000000000000000, 0.000000000000000000, 283.5832628385307999 ) ) ;
#12535=VERTEX_POINT ( 'NONE', #11800 ) ;
#12537=VERTEX_POINT ( 'NONE', #18066 ) ;
#12538=ADVANCED_FACE ( 'NONE', ( #7022 ), #8452, .F. ) ;
#12539=AXIS2_PLACEMENT_3D ( 'NONE', #15989, #2182, #17635 ) ;
#12540=ORIENTED_EDGE ( 'NONE', *, *, #5515, .T. ) ;
#12541=DIRECTION ( 'NONE',  ( 0.5000000000000009992, -0.8660254037844380415, 0.000000000000000000 ) ) ;
#12543=ORIENTED_EDGE ( 'NONE', *, *, #6119, .T. ) ;
#12544=DIRECTION ( 'NONE',  ( -0.3420201433256568335, -0.9396926207859127578, 0.000000000000000000 ) ) ;
#12545=EDGE_CURVE ( 'NONE', #17498, #16184, #10374, .T. ) ;
#12548=LINE ( 'NONE', #6532, #3080 ) ;
#12553=ORIENTED_EDGE ( 'NONE', *, *, #4222, .F. ) ;
#12559=LINE ( 'NONE', #18823, #12415 ) ;
#12562=DIRECTION ( 'NONE',  ( 0.9396926207859127578, -0.3420201433256568335, 0.000000000000000000 ) ) ;
#12566=CARTESIAN_POINT ( 'NONE',  ( -61.81362617575094021, 11.73417718768112294, 293.5832628385307999 ) ) ;
#12567=VECTOR ( 'NONE', #17072, 1000.000000000000114 ) ;
#12568=ORIENTED_EDGE ( 'NONE', *, *, #8660, .F. ) ;
#12569=CARTESIAN_POINT ( 'NONE',  ( -0.8220851292435327196, -58.69016442926522359, 248.9926560891072143 ) ) ;
#12570=CARTESIAN_POINT ( 'NONE',  ( 0.000000000000000000, 0.000000000000000000, 248.9926560891072143 ) ) ;
#12573=DIRECTION ( 'NONE',  ( 1.000000000000000000, 0.000000000000000000, 0.000000000000000000 ) ) ;
#12576=PLANE ( 'NONE',  #15704 ) ;
#12577=LINE ( 'NONE', #18840, #18446 ) ;
#12578=ORIENTED_EDGE ( 'NONE', *, *, #12976, .F. ) ;
#12579=CARTESIAN_POINT ( 'NONE',  ( 56.50329132715945235, -22.30005961346246579, 283.5832628385307999 ) ) ;
#12580=DIRECTION ( 'NONE',  ( 1.000000000000000000, 0.000000000000000000, 0.000000000000000000 ) ) ;
#12583=VERTEX_POINT ( 'NONE', #14884 ) ;
#12584=DIRECTION ( 'NONE',  ( 0.4999999999999949485, 0.8660254037844415942, -0.000000000000000000 ) ) ;
#12587=AXIS2_PLACEMENT_3D ( 'NONE', #4642, #10867, #15587 ) ;
#12590=CIRCLE ( 'NONE', #515, 60.74260934110282051 ) ;
#12591=ORIENTED_EDGE ( 'NONE', *, *, #6786, .F. ) ;
#12595=DIRECTION ( 'NONE',  ( -0.7660444431189792347, 0.6427876096865379196, 0.000000000000000000 ) ) ;
#12596=ORIENTED_EDGE ( 'NONE', *, *, #1601, .F. ) ;
#12597=FACE_OUTER_BOUND ( 'NONE', #4269, .T. ) ;
#12598=FACE_OUTER_BOUND ( 'NONE', #13639, .T. ) ;
#12599=CARTESIAN_POINT ( 'NONE',  ( -2.240720816136042348, 5.281164089014786178, 283.5832628385307999 ) ) ;
#12602=AXIS2_PLACEMENT_3D ( 'NONE', #5892, #16935, #5997 ) ;
#12604=DIRECTION ( 'NONE',  ( -0.6427876096865300370, -0.7660444431189858960, 0.000000000000000000 ) ) ;
#12611=VERTEX_POINT ( 'NONE', #5199 ) ;
#12612=ADVANCED_FACE ( 'NONE', ( #3654 ), #13978, .T. ) ;
#12614=CARTESIAN_POINT ( 'NONE',  ( 0.8220851292435327196, 78.26059000578311498, 248.9926560891072143 ) ) ;
#12615=ORIENTED_EDGE ( 'NONE', *, *, #10383, .F. ) ;
#12618=ADVANCED_FACE ( 'NONE', ( #3843 ), #17871, .T. ) ;
#12619=VECTOR ( 'NONE', #2687, 1000.000000000000000 ) ;
#12620=ORIENTED_EDGE ( 'NONE', *, *, #9158, .F. ) ;
#12622=VECTOR ( 'NONE', #4807, 1000.000000000000000 ) ;
#12623=DIRECTION ( 'NONE',  ( 1.000000000000000000, 0.000000000000000000, 0.000000000000000000 ) ) ;
#12624=FACE_OUTER_BOUND ( 'NONE', #16208, .T. ) ;
#12626=DIRECTION ( 'NONE',  ( -0.000000000000000000, -0.000000000000000000, 1.000000000000000000 ) ) ;
#12628=CARTESIAN_POINT ( 'NONE',  ( 68.46530598706793569, -37.93579148621486041, 248.9926560891072143 ) ) ;
#12629=CARTESIAN_POINT ( 'NONE',  ( 30.25670013172214468, 55.16472960512381718, 293.5832628385307999 ) ) ;
#12630=EDGE_CURVE ( 'NONE', #16844, #18605, #8844, .T. ) ;
#12632=LINE ( 'NONE', #6613, #15941 ) ;
#12633=VECTOR ( 'NONE', #18471, 1000.000000000000000 ) ;
#12634=ADVANCED_FACE ( 'NONE', ( #10471 ), #10572, .F. ) ;
#12637=CIRCLE ( 'NONE', #4815, 60.74260934110282051 ) ;
#12643=ORIENTED_EDGE ( 'NONE', *, *, #6854, .T. ) ;
#12647=CARTESIAN_POINT ( 'NONE',  ( -51.77076963420845601, 31.77187437101486367, 293.5832628385307999 ) ) ;
#12649=PLANE ( 'NONE',  #12022 ) ;
#12652=VERTEX_POINT ( 'NONE', #13435 ) ;
#12653=LINE ( 'NONE', #18914, #7378 ) ;
#12654=DIRECTION ( 'NONE',  ( -0.8830229359480271656, -0.4693298356057563625, 0.000000000000000000 ) ) ;
#12655=VECTOR ( 'NONE', #12445, 1000.000000000000000 ) ;
#12662=CARTESIAN_POINT ( 'NONE',  ( 0.000000000000000000, 0.000000000000000000, 283.5832628385307999 ) ) ;
#12663=CARTESIAN_POINT ( 'NONE',  ( 0.000000000000000000, 0.000000000000000000, 293.5832628385307999 ) ) ;
#12668=LINE ( 'NONE', #1940, #11205 ) ;
#12670=AXIS2_PLACEMENT_3D ( 'NONE', #10785, #12006, #13647 ) ;
#12671=VERTEX_POINT ( 'NONE', #8942 ) ;
#12672=CARTESIAN_POINT ( 'NONE',  ( -47.66508197439443961, 41.06890862491521688, 248.9926560891072143 ) ) ;
#12676=CARTESIAN_POINT ( 'NONE',  ( 0.000000000000000000, 0.000000000000000000, 283.5832628385307999 ) ) ;
#12678=LINE ( 'NONE', #9204, #18838 ) ;
#12679=CARTESIAN_POINT ( 'NONE',  ( -12.78021302872797449, 77.21438937758516374, 248.9926560891072143 ) ) ;
#12680=VECTOR ( 'NONE', #10397, 999.9999999999998863 ) ;
#12682=DIRECTION ( 'NONE',  ( 0.7881095627315598540, 0.6155349844899715706, 0.000000000000000000 ) ) ;
#12683=CYLINDRICAL_SURFACE ( 'NONE', #19101, 62.91752772691707207 ) ;
#12684=AXIS2_PLACEMENT_3D ( 'NONE', #10314, #11843, #914 ) ;
#12685=VERTEX_POINT ( 'NONE', #1282 ) ;
#12687=FACE_OUTER_BOUND ( 'NONE', #19757, .T. ) ;
#12690=VERTEX_POINT ( 'NONE', #15185 ) ;
#12693=VERTEX_POINT ( 'NONE', #18162 ) ;
#12695=ORIENTED_EDGE ( 'NONE', *, *, #15530, .T. ) ;
#12696=VECTOR ( 'NONE', #1510, 1000.000000000000000 ) ;
#12698=ORIENTED_EDGE ( 'NONE', *, *, #13026, .T. ) ;
#12704=CARTESIAN_POINT ( 'NONE',  ( 0.000000000000000000, 0.000000000000000000, 283.5832628385307999 ) ) ;
#12710=CARTESIAN_POINT ( 'NONE',  ( 47.29944656917758294, 41.48948842197133757, 248.9926560891072143 ) ) ;
#12716=VECTOR ( 'NONE', #6537, 1000.000000000000000 ) ;
#12717=EDGE_CURVE ( 'NONE', #1375, #9156, #15279, .T. ) ;
#12718=ORIENTED_EDGE ( 'NONE', *, *, #10361, .T. ) ;
#12722=EDGE_CURVE ( 'NONE', #7860, #6960, #1226, .T. ) ;
#12723=ORIENTED_EDGE ( 'NONE', *, *, #16163, .T. ) ;
#12724=ADVANCED_FACE ( 'NONE', ( #7412 ), #18894, .T. ) ;
#12727=EDGE_CURVE ( 'NONE', #16043, #11394, #9258, .T. ) ;
#12729=LINE ( 'NONE', #20198, #911 ) ;
#12733=LINE ( 'NONE', #5078, #17407 ) ;
#12736=DIRECTION ( 'NONE',  ( 1.000000000000000000, 0.000000000000000000, 0.000000000000000000 ) ) ;
#12737=EDGE_CURVE ( 'NONE', #15302, #10141, #19895, .T. ) ;
#12738=ORIENTED_EDGE ( 'NONE', *, *, #2640, .T. ) ;
#12741=AXIS2_PLACEMENT_3D ( 'NONE', #13834, #1466, #18449 ) ;
#12748=EDGE_CURVE ( 'NONE', #9808, #6926, #5890, .T. ) ;
#12750=DIRECTION ( 'NONE',  ( -0.2080686897406943958, -0.9781142164131909622, 0.000000000000000000 ) ) ;
#12759=CARTESIAN_POINT ( 'NONE',  ( 57.55901709132171362, 11.54977938102105028, 112.0427633081291816 ) ) ;
#12761=CARTESIAN_POINT ( 'NONE',  ( -25.99419088092141550, 73.82206860051556419, 248.9926560891072143 ) ) ;
#12762=CARTESIAN_POINT ( 'NONE',  ( 77.21438937758502163, 12.78021302872874010, 112.0427633081291816 ) ) ;
#12764=DIRECTION ( 'NONE',  ( -0.000000000000000000, -0.000000000000000000, 1.000000000000000000 ) ) ;
#12766=LINE ( 'NONE', #4698, #20164 ) ;
#12769=VECTOR ( 'NONE', #2524, 1000.000000000000000 ) ;
#12770=CYLINDRICAL_SURFACE ( 'NONE', #18416, 60.74260934110282051 ) ;
#12773=ORIENTED_EDGE ( 'NONE', *, *, #6486, .F. ) ;
#12774=CARTESIAN_POINT ( 'NONE',  ( 59.30716253403183913, -13.12726406102058441, 293.5832628385307999 ) ) ;
#12775=EDGE_CURVE ( 'NONE', #3096, #11476, #14272, .T. ) ;
#12777=EDGE_CURVE ( 'NONE', #7733, #9985, #154, .T. ) ;
#12779=CARTESIAN_POINT ( 'NONE',  ( 32.61983739937762294, 51.24071425735590424, 283.5832628385307999 ) ) ;
#12782=SURFACE_STYLE_USAGE ( .BOTH. , #6848 ) ;
#12783=CYLINDRICAL_SURFACE ( 'NONE', #13543, 60.74260934110282051 ) ;
#12785=VECTOR ( 'NONE', #8823, 1000.000000000000000 ) ;
#12787=LINE ( 'NONE', #805, #15365 ) ;
#12788=CARTESIAN_POINT ( 'NONE',  ( -77.21438937758510690, -12.78021302872823384, 112.0427633081291816 ) ) ;
#12789=VERTEX_POINT ( 'NONE', #15709 ) ;
#12791=ADVANCED_FACE ( 'NONE', ( #14170 ), #11192, .T. ) ;
#12795=ORIENTED_EDGE ( 'NONE', *, *, #17181, .T. ) ;
#12796=LINE ( 'NONE', #14126, #8751 ) ;
#12799=EDGE_LOOP ( 'NONE', ( #17593, #2536, #5436, #7964 ) ) ;
#12802=ORIENTED_EDGE ( 'NONE', *, *, #19418, .F. ) ;
#12805=ORIENTED_EDGE ( 'NONE', *, *, #6134, .T. ) ;
#12810=ADVANCED_FACE ( 'NONE', ( #12624 ), #18885, .T. ) ;
#12811=DIRECTION ( 'NONE',  ( 0.2080686897406943681, 0.9781142164131909622, 0.000000000000000000 ) ) ;
#12813=PLANE ( 'NONE',  #10805 ) ;
#12815=CARTESIAN_POINT ( 'NONE',  ( 0.000000000000000000, 0.000000000000000000, 248.9926560891072143 ) ) ;
#12818=VECTOR ( 'NONE', #13946, 1000.000000000000000 ) ;
#12819=AXIS2_PLACEMENT_3D ( 'NONE', #11961, #2574, #2778 ) ;
#12820=ORIENTED_EDGE ( 'NONE', *, *, #8781, .T. ) ;
#12822=VERTEX_POINT ( 'NONE', #17456 ) ;
#12824=CARTESIAN_POINT ( 'NONE',  ( 0.000000000000000000, 0.000000000000000000, 248.9926560891072143 ) ) ;
#12828=DIRECTION ( 'NONE',  ( 0.000000000000000000, 0.000000000000000000, 1.000000000000000000 ) ) ;
#12830=CARTESIAN_POINT ( 'NONE',  ( -11.00103590902911499, -57.65577537092155325, 112.0427633081292385 ) ) ;
#12833=LINE ( 'NONE', #8330, #2289 ) ;
#12835=FACE_OUTER_BOUND ( 'NONE', #11031, .T. ) ;
#12838=CARTESIAN_POINT ( 'NONE',  ( 0.000000000000000000, 0.000000000000000000, 248.9926560891072143 ) ) ;
#12841=VERTEX_POINT ( 'NONE', #1893 ) ;
#12845=ORIENTED_EDGE ( 'NONE', *, *, #19608, .T. ) ;
#12846=CARTESIAN_POINT ( 'NONE',  ( -49.07263256785925876, 39.37628763770471352, 132.4711112102474146 ) ) ;
#12848=CARTESIAN_POINT ( 'NONE',  ( 60.47951622432751151, 49.67518383744852883, 132.4711112102474146 ) ) ;
#12850=EDGE_CURVE ( 'NONE', #4753, #16956, #12729, .T. ) ;
#12853=PLANE ( 'NONE',  #15490 ) ;
#12854=VECTOR ( 'NONE', #13700, 999.9999999999998863 ) ;
#12855=DIRECTION ( 'NONE',  ( -0.9902903945359624593, -0.1390141521205945918, 0.000000000000000000 ) ) ;
#12858=CARTESIAN_POINT ( 'NONE',  ( 0.000000000000000000, 0.000000000000000000, 83.57543755549745867 ) ) ;
#12860=CARTESIAN_POINT ( 'NONE',  ( -38.35506425062487779, -44.43084819159262366, 132.4711112102474146 ) ) ;
#12862=FACE_OUTER_BOUND ( 'NONE', #9832, .T. ) ;
#12863=PLANE ( 'NONE',  #8322 ) ;
#12864=EDGE_CURVE ( 'NONE', #13055, #14795, #7713, .T. ) ;
#12866=VECTOR ( 'NONE', #539, 999.9999999999998863 ) ;
#12868=DIRECTION ( 'NONE',  ( 1.000000000000000000, 0.000000000000000000, -0.000000000000000000 ) ) ;
#12870=EDGE_CURVE ( 'NONE', #14947, #3300, #350, .T. ) ;
#12874=VERTEX_POINT ( 'NONE', #6604 ) ;
#12878=EDGE_CURVE ( 'NONE', #12535, #93, #14065, .T. ) ;
#12879=ORIENTED_EDGE ( 'NONE', *, *, #10042, .T. ) ;
#12880=VECTOR ( 'NONE', #10739, 1000.000000000000114 ) ;
#12885=FACE_OUTER_BOUND ( 'NONE', #305, .T. ) ;
#12886=CARTESIAN_POINT ( 'NONE',  ( 56.12853591711344592, -23.22718332831461652, 293.5832628385307999 ) ) ;
#12888=FACE_OUTER_BOUND ( 'NONE', #9516, .T. ) ;
#12889=EDGE_CURVE ( 'NONE', #2638, #182, #4504, .T. ) ;
#12894=DIRECTION ( 'NONE',  ( -0.9396926207859068736, -0.3420201433256725987, -0.000000000000000000 ) ) ;
#12896=ORIENTED_EDGE ( 'NONE', *, *, #8971, .T. ) ;
#12902=EDGE_CURVE ( 'NONE', #13894, #15468, #1486, .T. ) ;
#12909=VECTOR ( 'NONE', #16716, 999.9999999999998863 ) ;
#12912=EDGE_CURVE ( 'NONE', #18654, #1634, #3328, .T. ) ;
#12913=ADVANCED_FACE ( 'NONE', ( #7917 ), #9360, .F. ) ;
#12914=DIRECTION ( 'NONE',  ( 0.6155349844899715706, -0.7881095627315598540, 0.000000000000000000 ) ) ;
#12921=ADVANCED_FACE ( 'NONE', ( #9965 ), #14863, .F. ) ;
#12922=EDGE_LOOP ( 'NONE', ( #19322, #14062, #12999, #6708 ) ) ;
#12924=ORIENTED_EDGE ( 'NONE', *, *, #2057, .T. ) ;
#12926=VECTOR ( 'NONE', #19501, 1000.000000000000000 ) ;
#12928=LINE ( 'NONE', #2099, #276 ) ;
#12931=CARTESIAN_POINT ( 'NONE',  ( 79.75827554147308263, 0.000000000000000000, 248.9926560891072143 ) ) ;
#12933=LINE ( 'NONE', #17662, #12052 ) ;
#12935=DIRECTION ( 'NONE',  ( 0.000000000000000000, 0.000000000000000000, 1.000000000000000000 ) ) ;
#12936=ORIENTED_EDGE ( 'NONE', *, *, #11345, .T. ) ;
#12937=DIRECTION ( 'NONE',  ( 1.000000000000000000, 0.000000000000000000, 0.000000000000000000 ) ) ;
#12939=ORIENTED_EDGE ( 'NONE', *, *, #14655, .F. ) ;
#12940=ORIENTED_EDGE ( 'NONE', *, *, #1111, .T. ) ;
#12941=VECTOR ( 'NONE', #15419, 1000.000000000000000 ) ;
#12942=ORIENTED_EDGE ( 'NONE', *, *, #6366, .T. ) ;
#12944=CARTESIAN_POINT ( 'NONE',  ( 12.14914984460761360, 59.51523122377248853, 283.5832628385307999 ) ) ;
#12945=AXIS2_PLACEMENT_3D ( 'NONE', #19123, #8662, #18174 ) ;
#12946=ORIENTED_EDGE ( 'NONE', *, *, #4018, .F. ) ;
#12949=LINE ( 'NONE', #13339, #6356 ) ;
#12951=EDGE_LOOP ( 'NONE', ( #1781, #721, #18196, #2048 ) ) ;
#12954=ORIENTED_EDGE ( 'NONE', *, *, #1677, .T. ) ;
#12959=AXIS2_PLACEMENT_3D ( 'NONE', #14020, #5746, #11962 ) ;
#12965=CARTESIAN_POINT ( 'NONE',  ( 56.50138340076689047, -22.29928840491054132, 283.5832628385307999 ) ) ;
#12968=EDGE_CURVE ( 'NONE', #9508, #19079, #459, .T. ) ;
#12970=VERTEX_POINT ( 'NONE', #8224 ) ;
#12973=EDGE_CURVE ( 'NONE', #17837, #13913, #11595, .T. ) ;
#12974=CARTESIAN_POINT ( 'NONE',  ( -0.7000608949449729224, -5.693982670708925831, 293.5832628385307999 ) ) ;
#12975=VECTOR ( 'NONE', #13840, 1000.000000000000227 ) ;
#12976=EDGE_CURVE ( 'NONE', #18905, #18064, #12928, .T. ) ;
#12985=CARTESIAN_POINT ( 'NONE',  ( 0.000000000000000000, 0.000000000000000000, 283.5832628385307999 ) ) ;
#12991=EDGE_LOOP ( 'NONE', ( #1712, #13815, #12845, #16811 ) ) ;
#12992=EDGE_CURVE ( 'NONE', #3335, #19683, #13215, .T. ) ;
#12993=VECTOR ( 'NONE', #2884, 1000.000000000000000 ) ;
#12994=CARTESIAN_POINT ( 'NONE',  ( -1.379293853801755176, 58.69016442926522359, 132.4711112102474146 ) ) ;
#12996=ORIENTED_EDGE ( 'NONE', *, *, #3283, .T. ) ;
#12997=ORIENTED_EDGE ( 'NONE', *, *, #6252, .F. ) ;
#12998=EDGE_LOOP ( 'NONE', ( #17824, #7673, #16007, #20214 ) ) ;
#12999=ORIENTED_EDGE ( 'NONE', *, *, #11146, .T. ) ;
#13000=LINE ( 'NONE', #8403, #15322 ) ;
#13005=DIRECTION ( 'NONE',  ( -0.000000000000000000, -0.000000000000000000, 1.000000000000000000 ) ) ;
#13008=VECTOR ( 'NONE', #8124, 1000.000000000000000 ) ;
#13010=VECTOR ( 'NONE', #13479, 1000.000000000000000 ) ;
#13011=CARTESIAN_POINT ( 'NONE',  ( 48.17959877923549072, 36.99514631729036296, 283.5832628385307999 ) ) ;
#13014=DIRECTION ( 'NONE',  ( -0.000000000000000000, -0.000000000000000000, 1.000000000000000000 ) ) ;
#13017=ADVANCED_FACE ( 'NONE', ( #19479 ), #16318, .F. ) ;
#13020=VECTOR ( 'NONE', #9860, 1000.000000000000000 ) ;
#13022=ORIENTED_EDGE ( 'NONE', *, *, #8774, .T. ) ;
#13023=VERTEX_POINT ( 'NONE', #5177 ) ;
#13024=EDGE_CURVE ( 'NONE', #11048, #18614, #8532, .T. ) ;
#13025=CARTESIAN_POINT ( 'NONE',  ( 12.78021302872850562, -77.21438937758507848, 112.0427633081291816 ) ) ;
#13026=EDGE_CURVE ( 'NONE', #11442, #7743, #17953, .T. ) ;
#13028=CARTESIAN_POINT ( 'NONE',  ( 47.56406379474552182, 37.78325588002191893, 293.5832628385307999 ) ) ;
#13029=DIRECTION ( 'NONE',  ( -0.000000000000000000, -0.000000000000000000, 1.000000000000000000 ) ) ;
#13032=EDGE_LOOP ( 'NONE', ( #18941, #19296, #11821, #13947 ) ) ;
#13033=LINE ( 'NONE', #17561, #13338 ) ;
#13036=CARTESIAN_POINT ( 'NONE',  ( 19.74955734592081669, 8.656064874777317897, 248.9926560891072143 ) ) ;
#13037=EDGE_CURVE ( 'NONE', #2316, #18758, #848, .T. ) ;
#13040=ORIENTED_EDGE ( 'NONE', *, *, #11997, .T. ) ;
#13041=ORIENTED_EDGE ( 'NONE', *, *, #6092, .F. ) ;
#13045=VECTOR ( 'NONE', #16936, 1000.000000000000114 ) ;
#13046=ORIENTED_EDGE ( 'NONE', *, *, #5021, .F. ) ;
#13047=ORIENTED_EDGE ( 'NONE', *, *, #4532, .F. ) ;
#13049=DIRECTION ( 'NONE',  ( -0.4999999999999919509, -0.8660254037844432595, 0.000000000000000000 ) ) ;
#13050=DIRECTION ( 'NONE',  ( 0.000000000000000000, 0.000000000000000000, 1.000000000000000000 ) ) ;
#13054=EDGE_CURVE ( 'NONE', #7743, #10155, #3922, .T. ) ;
#13055=VERTEX_POINT ( 'NONE', #5366 ) ;
#13057=DIRECTION ( 'NONE',  ( 0.7660444431189835646, -0.6427876096865328126, 0.000000000000000000 ) ) ;
#13061=CARTESIAN_POINT ( 'NONE',  ( -54.86954475316242252, 20.84572577951219330, 111.4180192758973931 ) ) ;
#13062=ORIENTED_EDGE ( 'NONE', *, *, #15819, .F. ) ;
#13065=VERTEX_POINT ( 'NONE', #3823 ) ;
#13067=DIRECTION ( 'NONE',  ( 0.5000000000000039968, -0.8660254037844363761, 0.000000000000000000 ) ) ;
#13068=EDGE_LOOP ( 'NONE', ( #5038, #11188, #7070 ) ) ;
#13070=CARTESIAN_POINT ( 'NONE',  ( 0.000000000000000000, 0.000000000000000000, 283.5832628385307999 ) ) ;
#13074=EDGE_CURVE ( 'NONE', #6267, #11201, #7099, .T. ) ;
#13075=EDGE_LOOP ( 'NONE', ( #3218, #6298, #7382, #5806 ) ) ;
#13078=LINE ( 'NONE', #17905, #19947 ) ;
#13079=CARTESIAN_POINT ( 'NONE',  ( 41.06890862491472660, 47.66508197439486594, 248.9926560891072143 ) ) ;
#13080=ORIENTED_EDGE ( 'NONE', *, *, #20235, .F. ) ;
#13081=DIRECTION ( 'NONE',  ( 0.9271237148521548344, -0.3747554100459928317, 0.000000000000000000 ) ) ;
#13082=CARTESIAN_POINT ( 'NONE',  ( 73.82206860051529418, 25.99419088092216867, 111.4180192758973362 ) ) ;
#13085=CARTESIAN_POINT ( 'NONE',  ( -4.581103194068993467, 3.453261854572370559, 293.5832628385307999 ) ) ;
#13086=ORIENTED_EDGE ( 'NONE', *, *, #7162, .F. ) ;
#13090=ORIENTED_EDGE ( 'NONE', *, *, #9852, .F. ) ;
#13091=ORIENTED_EDGE ( 'NONE', *, *, #10481, .F. ) ;
#13092=ORIENTED_EDGE ( 'NONE', *, *, #8660, .T. ) ;
#13094=CARTESIAN_POINT ( 'NONE',  ( 61.81362617575102547, -11.73417718768070372, 293.5832628385307999 ) ) ;
#13095=VECTOR ( 'NONE', #4152, 1000.000000000000000 ) ;
#13098=PLANE ( 'NONE',  #5095 ) ;
#13099=CARTESIAN_POINT ( 'NONE',  ( -37.78198917157317993, 47.56244194535177883, 283.5832628385307999 ) ) ;
#13101=EDGE_CURVE ( 'NONE', #7659, #12671, #15371, .T. ) ;
#13103=FACE_OUTER_BOUND ( 'NONE', #10854, .T. ) ;
#13105=LINE ( 'NONE', #932, #10100 ) ;
#13109=DIRECTION ( 'NONE',  ( -0.000000000000000000, -0.000000000000000000, 1.000000000000000000 ) ) ;
#13111=ORIENTED_EDGE ( 'NONE', *, *, #13114, .F. ) ;
#13114=EDGE_CURVE ( 'NONE', #2315, #17279, #7292, .T. ) ;
#13117=DIRECTION ( 'NONE',  ( -0.9396926207859104263, 0.3420201433256630508, 0.000000000000000000 ) ) ;
#13119=DIRECTION ( 'NONE',  ( 1.000000000000000000, 0.000000000000000000, 0.000000000000000000 ) ) ;
#13123=PLANE ( 'NONE',  #572 ) ;
#13128=EDGE_CURVE ( 'NONE', #347, #18954, #9022, .T. ) ;
#13132=ORIENTED_EDGE ( 'NONE', *, *, #15155, .T. ) ;
#13133=CARTESIAN_POINT ( 'NONE',  ( 18.28503710798548454, -57.92514141135459482, 283.5832628385307999 ) ) ;
#13134=AXIS2_PLACEMENT_3D ( 'NONE', #15801, #14366, #3716 ) ;
#13135=AXIS2_PLACEMENT_3D ( 'NONE', #9820, #5325, #6859 ) ;
#13144=DIRECTION ( 'NONE',  ( -0.8479630283625716469, 0.5300553768524345344, 0.000000000000000000 ) ) ;
#13145=LINE ( 'NONE', #17685, #12716 ) ;
#13147=CARTESIAN_POINT ( 'NONE',  ( 0.000000000000000000, 0.000000000000000000, 283.5832628385307999 ) ) ;
#13148=LINE ( 'NONE', #5397, #7725 ) ;
#13150=DIRECTION ( 'NONE',  ( 1.000000000000000000, 0.000000000000000000, 0.000000000000000000 ) ) ;
#13157=DIRECTION ( 'NONE',  ( 0.000000000000000000, 0.000000000000000000, -1.000000000000000000 ) ) ;
#13160=EDGE_CURVE ( 'NONE', #14365, #1787, #4197, .T. ) ;
#13166=VECTOR ( 'NONE', #19225, 1000.000000000000227 ) ;
#13168=DIRECTION ( 'NONE',  ( -0.000000000000000000, -0.000000000000000000, 1.000000000000000000 ) ) ;
#13173=LINE ( 'NONE', #16568, #16359 ) ;
#13174=PLANE ( 'NONE',  #8658 ) ;
#13177=LINE ( 'NONE', #809, #14288 ) ;
#13178=DIRECTION ( 'NONE',  ( 1.000000000000000000, 0.000000000000000000, 0.000000000000000000 ) ) ;
#13179=CARTESIAN_POINT ( 'NONE',  ( 11.73417718768048701, 61.81362617575105389, 293.5832628385307999 ) ) ;
#13182=FACE_OUTER_BOUND ( 'NONE', #4226, .T. ) ;
#13186=AXIS2_PLACEMENT_3D ( 'NONE', #2573, #10148, #14843 ) ;
#13188=DIRECTION ( 'NONE',  ( 0.000000000000000000, 0.000000000000000000, -1.000000000000000000 ) ) ;
#13190=EDGE_LOOP ( 'NONE', ( #5916, #6436, #11903, #15617 ) ) ;
#13197=CARTESIAN_POINT ( 'NONE',  ( 1.379293853801755176, -78.26059000578310076, 248.9926560891072143 ) ) ;
#13199=VECTOR ( 'NONE', #5231, 1000.000000000000000 ) ;
#13200=CARTESIAN_POINT ( 'NONE',  ( 28.15057869795588985, 51.51682027493075111, 132.4711112102474146 ) ) ;
#13201=CARTESIAN_POINT ( 'NONE',  ( -78.26059000578311498, 0.8220851292432594937, 248.9926560891072143 ) ) ;
#13205=CARTESIAN_POINT ( 'NONE',  ( 17.50000000000001066, 0.000000000000000000, 293.5832628385307999 ) ) ;
#13207=VECTOR ( 'NONE', #9615, 1000.000000000000000 ) ;
#13210=AXIS2_PLACEMENT_3D ( 'NONE', #7856, #14407, #9395 ) ;
#13211=EDGE_CURVE ( 'NONE', #7403, #1374, #8794, .T. ) ;
#13214=EDGE_CURVE ( 'NONE', #11944, #321, #15131, .T. ) ;
#13215=LINE ( 'NONE', #563, #16937 ) ;
#13216=EDGE_CURVE ( 'NONE', #4335, #2635, #16620, .T. ) ;
#13217=CARTESIAN_POINT ( 'NONE',  ( 47.66508197439472383, -41.06890862491489003, 132.4711112102474146 ) ) ;
#13219=ORIENTED_EDGE ( 'NONE', *, *, #15285, .F. ) ;
#13223=DIRECTION ( 'NONE',  ( 0.000000000000000000, 0.000000000000000000, 1.000000000000000000 ) ) ;
#13224=CARTESIAN_POINT ( 'NONE',  ( -4.811834253408968642, -3.123743752084041425, 283.5832628385307999 ) ) ;
#13225=AXIS2_PLACEMENT_3D ( 'NONE', #604, #13168, #6849 ) ;
#13228=EDGE_CURVE ( 'NONE', #8156, #11394, #6143, .T. ) ;
#13234=CARTESIAN_POINT ( 'NONE',  ( -79.75827554147308263, 9.767571684737765249E-15, 112.9440587442963562 ) ) ;
#13235=FACE_OUTER_BOUND ( 'NONE', #6964, .T. ) ;
#13237=ORIENTED_EDGE ( 'NONE', *, *, #3247, .T. ) ;
#13240=CARTESIAN_POINT ( 'NONE',  ( 0.000000000000000000, 0.000000000000000000, 248.9926560891072143 ) ) ;
#13241=ADVANCED_FACE ( 'NONE', ( #18514 ), #7559, .T. ) ;
#13244=DIRECTION ( 'NONE',  ( -0.3747554100459959403, -0.9271237148521535021, 0.000000000000000000 ) ) ;
#13245=DIRECTION ( 'NONE',  ( 1.000000000000000000, 0.000000000000000000, 0.000000000000000000 ) ) ;
#13247=VECTOR ( 'NONE', #13117, 1000.000000000000000 ) ;
#13249=CARTESIAN_POINT ( 'NONE',  ( 55.16472960512370349, -30.25670013172234363, 248.9926560891072143 ) ) ;
#13250=EDGE_LOOP ( 'NONE', ( #4914, #10952, #8654, #19005 ) ) ;
#13252=EDGE_CURVE ( 'NONE', #9705, #4517, #1432, .T. ) ;
#13255=VERTEX_POINT ( 'NONE', #2664 ) ;
#13256=DIRECTION ( 'NONE',  ( 0.3747554100459959958, 0.9271237148521535021, 0.000000000000000000 ) ) ;
#13257=ORIENTED_EDGE ( 'NONE', *, *, #3793, .F. ) ;
#13259=DIRECTION ( 'NONE',  ( 0.4999999999999979461, 0.8660254037844397068, 0.000000000000000000 ) ) ;
#13262=ADVANCED_FACE ( 'NONE', ( #13586 ), #13899, .T. ) ;
#13264=DIRECTION ( 'NONE',  ( -0.000000000000000000, -0.000000000000000000, 1.000000000000000000 ) ) ;
#13266=ORIENTED_EDGE ( 'NONE', *, *, #16121, .F. ) ;
#13267=AXIS2_PLACEMENT_3D ( 'NONE', #15766, #14435, #17615 ) ;
#13269=DIRECTION ( 'NONE',  ( 1.000000000000000000, 0.000000000000000000, 0.000000000000000000 ) ) ;
#13270=ADVANCED_FACE ( 'NONE', ( #3276 ), #4707, .T. ) ;
#13271=CARTESIAN_POINT ( 'NONE',  ( 47.56244194535165093, 37.78198917157335757, 293.5832628385307999 ) ) ;
#13272=LINE ( 'NONE', #5424, #7989 ) ;
#13273=CARTESIAN_POINT ( 'NONE',  ( 56.50329132715945235, -22.30005961346246579, 293.5832628385307999 ) ) ;
#13276=DIRECTION ( 'NONE',  ( -1.000000000000000000, -1.047444401652940164E-14, 0.000000000000000000 ) ) ;
#13278=VERTEX_POINT ( 'NONE', #12672 ) ;
#13279=CARTESIAN_POINT ( 'NONE',  ( 60.68773558783009747, -2.629322876227576433, 293.5832628385307999 ) ) ;
#13280=CARTESIAN_POINT ( 'NONE',  ( 56.50138340076689047, -22.29928840491054132, 283.5832628385307999 ) ) ;
#13282=VERTEX_POINT ( 'NONE', #9704 ) ;
#13286=DIRECTION ( 'NONE',  ( 0.8479630283625716469, -0.5300553768524345344, 0.000000000000000000 ) ) ;
#13288=ORIENTED_EDGE ( 'NONE', *, *, #17969, .F. ) ;
#13291=CIRCLE ( 'NONE', #3520, 62.91752772691707207 ) ;
#13294=PLANE ( 'NONE',  #2416 ) ;
#13295=VECTOR ( 'NONE', #7445, 1000.000000000000000 ) ;
#13302=DIRECTION ( 'NONE',  ( -0.1736481776669172583, -0.9848077530122103518, 0.000000000000000000 ) ) ;
#13307=VERTEX_POINT ( 'NONE', #12774 ) ;
#13310=ORIENTED_EDGE ( 'NONE', *, *, #16128, .T. ) ;
#13311=CARTESIAN_POINT ( 'NONE',  ( 45.48770046196260353, 37.09555676057011908, 132.4711112102474146 ) ) ;
#13312=PLANE ( 'NONE',  #8941 ) ;
#13315=FACE_OUTER_BOUND ( 'NONE', #20122, .T. ) ;
#13318=CARTESIAN_POINT ( 'NONE',  ( -1.289614712049164114, 5.590028426173843101, 283.5832628385307999 ) ) ;
#13320=FACE_OUTER_BOUND ( 'NONE', #16667, .T. ) ;
#13322=DIRECTION ( 'NONE',  ( -0.000000000000000000, -0.000000000000000000, 1.000000000000000000 ) ) ;
#13326=AXIS2_PLACEMENT_3D ( 'NONE', #14429, #18664, #10865 ) ;
#13328=VECTOR ( 'NONE', #9628, 999.9999999999998863 ) ;
#13329=VERTEX_POINT ( 'NONE', #1531 ) ;
#13330=EDGE_CURVE ( 'NONE', #13976, #3773, #17608, .T. ) ;
#13332=ORIENTED_EDGE ( 'NONE', *, *, #772, .T. ) ;
#13334=VERTEX_POINT ( 'NONE', #9607 ) ;
#13336=AXIS2_PLACEMENT_3D ( 'NONE', #4147, #11711, #18165 ) ;
#13338=VECTOR ( 'NONE', #4769, 1000.000000000000114 ) ;
#13339=CARTESIAN_POINT ( 'NONE',  ( -57.65577537092151772, 11.00103590902930328, 132.4711112102474146 ) ) ;
#13345=EDGE_LOOP ( 'NONE', ( #1910, #5688, #1853, #14078 ) ) ;
#13346=FACE_OUTER_BOUND ( 'NONE', #19583, .T. ) ;
#13347=FACE_OUTER_BOUND ( 'NONE', #2740, .T. ) ;
#13351=DIRECTION ( 'NONE',  ( -0.9993852124581887875, 0.03505990758545896036, 0.000000000000000000 ) ) ;
#13353=VECTOR ( 'NONE', #19293, 1000.000000000000000 ) ;
#13354=VECTOR ( 'NONE', #7200, 999.9999999999998863 ) ;
#13355=EDGE_LOOP ( 'NONE', ( #18778, #3763, #3947 ) ) ;
#13356=EDGE_CURVE ( 'NONE', #9378, #4265, #3173, .T. ) ;
#13359=EDGE_CURVE ( 'NONE', #2297, #19640, #11391, .T. ) ;
#13360=ORIENTED_EDGE ( 'NONE', *, *, #370, .F. ) ;
#13362=EDGE_LOOP ( 'NONE', ( #101, #12001, #19311, #10464 ) ) ;
#13363=ORIENTED_EDGE ( 'NONE', *, *, #18257, .F. ) ;
#13364=DIRECTION ( 'NONE',  ( -0.1736481776669206722, -0.9848077530122097967, 0.000000000000000000 ) ) ;
#13365=FACE_OUTER_BOUND ( 'NONE', #15518, .T. ) ;
#13366=LINE ( 'NONE', #2647, #1488 ) ;
#13367=DIRECTION ( 'NONE',  ( 1.000000000000000000, 0.000000000000000000, 0.000000000000000000 ) ) ;
#13373=CARTESIAN_POINT ( 'NONE',  ( 0.000000000000000000, 0.000000000000000000, 248.9926560891072143 ) ) ;
#13375=DIRECTION ( 'NONE',  ( -0.9396926207859114255, 0.3420201433256601642, 0.000000000000000000 ) ) ;
#13378=CARTESIAN_POINT ( 'NONE',  ( 0.000000000000000000, 0.000000000000000000, 293.5832628385307999 ) ) ;
#13380=ORIENTED_EDGE ( 'NONE', *, *, #10844, .F. ) ;
#13382=CARTESIAN_POINT ( 'NONE',  ( 0.000000000000000000, 0.000000000000000000, 132.4711112102474146 ) ) ;
#13385=EDGE_CURVE ( 'NONE', #15515, #13023, #1834, .T. ) ;
#13386=ORIENTED_EDGE ( 'NONE', *, *, #9651, .T. ) ;
#13387=ADVANCED_FACE ( 'NONE', ( #96 ), #3072, .F. ) ;
#13388=ORIENTED_EDGE ( 'NONE', *, *, #13792, .F. ) ;
#13391=LINE ( 'NONE', #18210, #10997 ) ;
#13395=EDGE_CURVE ( 'NONE', #18230, #4188, #8066, .T. ) ;
#13396=VECTOR ( 'NONE', #11148, 999.9999999999998863 ) ;
#13397=CARTESIAN_POINT ( 'NONE',  ( -58.69016442926521648, -1.379293853801960124, 112.7772637782949516 ) ) ;
#13398=CARTESIAN_POINT ( 'NONE',  ( -30.53958573130872978, 50.13752642112859803, 132.4711112102474146 ) ) ;
#13401=CARTESIAN_POINT ( 'NONE',  ( 45.46865632508072963, -40.28046525994365368, 293.5832628385307999 ) ) ;
#13402=DIRECTION ( 'NONE',  ( -0.000000000000000000, -0.000000000000000000, 1.000000000000000000 ) ) ;
#13405=CARTESIAN_POINT ( 'NONE',  ( 0.000000000000000000, 0.000000000000000000, 248.9926560891072143 ) ) ;
#13406=EDGE_CURVE ( 'NONE', #6975, #9578, #6347, .T. ) ;
#13407=ORIENTED_EDGE ( 'NONE', *, *, #5928, .T. ) ;
#13408=VECTOR ( 'NONE', #490, 1000.000000000000000 ) ;
#13412=DIRECTION ( 'NONE',  ( -0.000000000000000000, -0.000000000000000000, 1.000000000000000000 ) ) ;
#13415=CARTESIAN_POINT ( 'NONE',  ( -38.41834839689332171, 68.18670162478844077, 110.9660488491356887 ) ) ;
#13417=DIRECTION ( 'NONE',  ( 0.000000000000000000, 0.000000000000000000, 1.000000000000000000 ) ) ;
#13418=ORIENTED_EDGE ( 'NONE', *, *, #10006, .T. ) ;
#13419=CARTESIAN_POINT ( 'NONE',  ( 45.48770046196260353, 37.09555676057011908, 110.7293897666001214 ) ) ;
#13422=PLANE ( 'NONE',  #4310 ) ;
#13425=DIRECTION ( 'NONE',  ( 1.000000000000000000, 0.000000000000000000, 0.000000000000000000 ) ) ;
#13426=CARTESIAN_POINT ( 'NONE',  ( 57.61627707419552280, 19.23614321207256239, 293.5832628385307999 ) ) ;
#13427=ORIENTED_EDGE ( 'NONE', *, *, #4068, .F. ) ;
#13428=EDGE_LOOP ( 'NONE', ( #18455, #12820, #17221, #3931 ) ) ;
#13429=ORIENTED_EDGE ( 'NONE', *, *, #13876, .F. ) ;
#13430=VERTEX_POINT ( 'NONE', #6844 ) ;
#13431=EDGE_CURVE ( 'NONE', #19763, #2611, #597, .T. ) ;
#13435=CARTESIAN_POINT ( 'NONE',  ( -30.25670013172252837, -55.16472960512360402, 248.9926560891072143 ) ) ;
#13436=ORIENTED_EDGE ( 'NONE', *, *, #10721, .F. ) ;
#13439=DIRECTION ( 'NONE',  ( 1.000000000000000000, 0.000000000000000000, 0.000000000000000000 ) ) ;
#13440=ORIENTED_EDGE ( 'NONE', *, *, #16547, .F. ) ;
#13443=DIRECTION ( 'NONE',  ( -0.7660444431189835646, 0.6427876096865328126, -0.000000000000000000 ) ) ;
#13446=DIRECTION ( 'NONE',  ( -0.1736481776669374366, 0.9848077530122066880, 0.000000000000000000 ) ) ;
#13447=CARTESIAN_POINT ( 'NONE',  ( 60.72279549541555355, -1.629937663769388090, 293.5832628385307999 ) ) ;
#13448=ORIENTED_EDGE ( 'NONE', *, *, #19988, .F. ) ;
#13449=CARTESIAN_POINT ( 'NONE',  ( 0.000000000000000000, 0.000000000000000000, 283.5832628385307999 ) ) ;
#13450=VECTOR ( 'NONE', #13109, 1000.000000000000000 ) ;
#13456=EDGE_CURVE ( 'NONE', #10750, #12303, #2044, .T. ) ;
#13459=AXIS2_PLACEMENT_3D ( 'NONE', #15027, #7255, #13477 ) ;
#13460=FACE_OUTER_BOUND ( 'NONE', #13766, .T. ) ;
#13463=DIRECTION ( 'NONE',  ( 0.5000000000000009992, -0.8660254037844380415, 0.000000000000000000 ) ) ;
#13464=ORIENTED_EDGE ( 'NONE', *, *, #17033, .F. ) ;
#13467=CARTESIAN_POINT ( 'NONE',  ( 0.000000000000000000, 0.000000000000000000, 283.5832628385307999 ) ) ;
#13469=AXIS2_PLACEMENT_3D ( 'NONE', #3553, #11009, #6531 ) ;
#13471=DIRECTION ( 'NONE',  ( 0.000000000000000000, 0.000000000000000000, -1.000000000000000000 ) ) ;
#13473=CARTESIAN_POINT ( 'NONE',  ( -54.67896814532655725, -21.36933070621745046, 111.4180192758973931 ) ) ;
#13476=PLANE ( 'NONE',  #9489 ) ;
#13477=DIRECTION ( 'NONE',  ( 1.000000000000000000, 0.000000000000000000, 0.000000000000000000 ) ) ;
#13479=DIRECTION ( 'NONE',  ( -0.000000000000000000, -0.000000000000000000, 1.000000000000000000 ) ) ;
#13480=DIRECTION ( 'NONE',  ( 1.000000000000000000, 0.000000000000000000, 0.000000000000000000 ) ) ;
#13483=ADVANCED_FACE ( 'NONE', ( #14810 ), #10200, .F. ) ;
#13485=EDGE_CURVE ( 'NONE', #13542, #10934, #18407, .T. ) ;
#13488=LINE ( 'NONE', #6969, #19181 ) ;
#13489=ORIENTED_EDGE ( 'NONE', *, *, #731, .F. ) ;
#13490=AXIS2_PLACEMENT_3D ( 'NONE', #769, #7017, #5480 ) ;
#13491=CARTESIAN_POINT ( 'NONE',  ( 0.000000000000000000, 0.000000000000000000, 283.5832628385307999 ) ) ;
#13496=ADVANCED_FACE ( 'NONE', ( #16061 ), #5217, .T. ) ;
#13498=PLANE ( 'NONE',  #151 ) ;
#13499=LINE ( 'NONE', #19750, #744 ) ;
#13500=DIRECTION ( 'NONE',  ( 1.000000000000000000, 0.000000000000000000, 0.000000000000000000 ) ) ;
#13503=VERTEX_POINT ( 'NONE', #17701 ) ;
#13505=CARTESIAN_POINT ( 'NONE',  ( -37.09555676056967144, 45.48770046196298011, 248.9926560891072143 ) ) ;
#13511=VECTOR ( 'NONE', #12212, 1000.000000000000000 ) ;
#13512=ORIENTED_EDGE ( 'NONE', *, *, #9001, .F. ) ;
#13516=LINE ( 'NONE', #19768, #15391 ) ;
#13517=DIRECTION ( 'NONE',  ( -0.000000000000000000, -0.000000000000000000, 1.000000000000000000 ) ) ;
#13518=EDGE_CURVE ( 'NONE', #16088, #11620, #16355, .T. ) ;
#13522=LINE ( 'NONE', #1044, #13354 ) ;
#13532=ORIENTED_EDGE ( 'NONE', *, *, #19369, .T. ) ;
#13533=DIRECTION ( 'NONE',  ( -0.000000000000000000, -0.000000000000000000, 1.000000000000000000 ) ) ;
#13534=VECTOR ( 'NONE', #6284, 1000.000000000000000 ) ;
#13538=EDGE_LOOP ( 'NONE', ( #11760, #11566, #3197, #5048 ) ) ;
#13542=VERTEX_POINT ( 'NONE', #7431 ) ;
#13543=AXIS2_PLACEMENT_3D ( 'NONE', #103, #9312, #7771 ) ;
#13544=CARTESIAN_POINT ( 'NONE',  ( 77.31114765718493231, -12.23146955673620795, 132.4711112102474146 ) ) ;
#13546=ORIENTED_EDGE ( 'NONE', *, *, #884, .T. ) ;
#13547=LINE ( 'NONE', #18167, #18595 ) ;
#13550=AXIS2_PLACEMENT_3D ( 'NONE', #11179, #8314, #8418 ) ;
#13555=ORIENTED_EDGE ( 'NONE', *, *, #18353, .F. ) ;
#13556=CARTESIAN_POINT ( 'NONE',  ( -25.47058595421603044, -74.01264520835144367, 248.9926560891072143 ) ) ;
#13558=VECTOR ( 'NONE', #13567, 1000.000000000000000 ) ;
#13559=ORIENTED_EDGE ( 'NONE', *, *, #4483, .T. ) ;
#13561=ORIENTED_EDGE ( 'NONE', *, *, #2609, .F. ) ;
#13562=ORIENTED_EDGE ( 'NONE', *, *, #19533, .F. ) ;
#13563=CYLINDRICAL_SURFACE ( 'NONE', #7791, 60.74260934110282051 ) ;
#13565=CARTESIAN_POINT ( 'NONE',  ( 0.000000000000000000, 0.000000000000000000, 283.5832628385307999 ) ) ;
#13567=DIRECTION ( 'NONE',  ( 0.000000000000000000, 0.000000000000000000, 1.000000000000000000 ) ) ;
#13568=CARTESIAN_POINT ( 'NONE',  ( -57.55901709132179178, -11.54977938102067547, 132.4711112102474146 ) ) ;
#13570=ORIENTED_EDGE ( 'NONE', *, *, #12777, .F. ) ;
#13571=DIRECTION ( 'NONE',  ( 0.000000000000000000, 0.000000000000000000, 1.000000000000000000 ) ) ;
#13572=DIRECTION ( 'NONE',  ( -0.3088643371590125697, 0.9511061040868803440, 0.000000000000000000 ) ) ;
#13578=CARTESIAN_POINT ( 'NONE',  ( 28.06584155524102187, -53.86996498385662591, 293.5832628385307999 ) ) ;
#13579=FACE_OUTER_BOUND ( 'NONE', #9148, .T. ) ;
#13581=CARTESIAN_POINT ( 'NONE',  ( -41.48948842197086151, 47.29944656917798795, 132.4711112102474146 ) ) ;
#13582=FACE_OUTER_BOUND ( 'NONE', #15778, .T. ) ;
#13583=ORIENTED_EDGE ( 'NONE', *, *, #18132, .F. ) ;
#13585=VERTEX_POINT ( 'NONE', #4061 ) ;
#13586=FACE_OUTER_BOUND ( 'NONE', #12434, .T. ) ;
#13587=VECTOR ( 'NONE', #477, 1000.000000000000000 ) ;
#13589=ADVANCED_FACE ( 'NONE', ( #8765 ), #18387, .F. ) ;
#13590=VERTEX_POINT ( 'NONE', #19809 ) ;
#13591=EDGE_CURVE ( 'NONE', #6775, #4330, #10489, .T. ) ;
#13593=CARTESIAN_POINT ( 'NONE',  ( -37.78198917157317993, 47.56244194535179304, 293.5832628385307999 ) ) ;
#13594=ORIENTED_EDGE ( 'NONE', *, *, #11115, .T. ) ;
#13597=AXIS2_PLACEMENT_3D ( 'NONE', #14624, #12401, #1095 ) ;
#13598=EDGE_CURVE ( 'NONE', #9705, #4730, #10392, .T. ) ;
#13600=FACE_OUTER_BOUND ( 'NONE', #13872, .T. ) ;
#13605=DIRECTION ( 'NONE',  ( -0.000000000000000000, 0.000000000000000000, 1.000000000000000000 ) ) ;
#13608=AXIS2_PLACEMENT_3D ( 'NONE', #1849, #8490, #6764 ) ;
#13609=DIRECTION ( 'NONE',  ( -0.000000000000000000, -0.000000000000000000, 1.000000000000000000 ) ) ;
#13611=ORIENTED_EDGE ( 'NONE', *, *, #19057, .T. ) ;
#13612=ORIENTED_EDGE ( 'NONE', *, *, #2417, .T. ) ;
#13614=EDGE_CURVE ( 'NONE', #5836, #5572, #4365, .T. ) ;
#13618=ORIENTED_EDGE ( 'NONE', *, *, #535, .T. ) ;
#13619=CARTESIAN_POINT ( 'NONE',  ( 59.30716253403183913, -13.12726406102058441, 283.5832628385307999 ) ) ;
#13621=AXIS2_PLACEMENT_3D ( 'NONE', #6546, #9397, #7857 ) ;
#13625=DIRECTION ( 'NONE',  ( 1.000000000000000000, 0.000000000000000000, 0.000000000000000000 ) ) ;
#13627=DIRECTION ( 'NONE',  ( 1.000000000000000000, 0.000000000000000000, 0.000000000000000000 ) ) ;
#13629=EDGE_CURVE ( 'NONE', #19407, #2612, #2534, .T. ) ;
#13635=LINE ( 'NONE', #19320, #2699 ) ;
#13638=ORIENTED_EDGE ( 'NONE', *, *, #3886, .F. ) ;
#13639=EDGE_LOOP ( 'NONE', ( #5117, #364, #6217, #9307 ) ) ;
#13641=EDGE_CURVE ( 'NONE', #3790, #10591, #11198, .T. ) ;
#13644=VERTEX_POINT ( 'NONE', #4163 ) ;
#13645=ADVANCED_FACE ( 'NONE', ( #16652 ), #7533, .F. ) ;
#13647=DIRECTION ( 'NONE',  ( 1.000000000000000000, 0.000000000000000000, 0.000000000000000000 ) ) ;
#13651=VECTOR ( 'NONE', #15500, 1000.000000000000114 ) ;
#13652=ORIENTED_EDGE ( 'NONE', *, *, #13759, .T. ) ;
#13656=FACE_OUTER_BOUND ( 'NONE', #18290, .T. ) ;
#13658=CARTESIAN_POINT ( 'NONE',  ( -53.86996498385653354, -28.06584155524119950, 283.5832628385307999 ) ) ;
#13661=ORIENTED_EDGE ( 'NONE', *, *, #20144, .T. ) ;
#13663=VECTOR ( 'NONE', #13879, 1000.000000000000227 ) ;
#13665=AXIS2_PLACEMENT_3D ( 'NONE', #11688, #5461, #17845 ) ;
#13668=CARTESIAN_POINT ( 'NONE',  ( 0.000000000000000000, 0.000000000000000000, 283.5832628385307999 ) ) ;
#13670=ORIENTED_EDGE ( 'NONE', *, *, #8335, .F. ) ;
#13672=EDGE_CURVE ( 'NONE', #15515, #13875, #2389, .T. ) ;
#13677=CYLINDRICAL_SURFACE ( 'NONE', #9348, 60.74260934110282051 ) ;
#13682=AXIS2_PLACEMENT_3D ( 'NONE', #14700, #689, #11434 ) ;
#13684=VERTEX_POINT ( 'NONE', #4262 ) ;
#13688=ORIENTED_EDGE ( 'NONE', *, *, #2241, .T. ) ;
#13695=VERTEX_POINT ( 'NONE', #15202 ) ;
#13697=AXIS2_PLACEMENT_3D ( 'NONE', #3946, #18070, #12009 ) ;
#13698=EDGE_CURVE ( 'NONE', #18902, #5832, #19913, .T. ) ;
#13699=CARTESIAN_POINT ( 'NONE',  ( 53.87178215532755132, 28.06680738835045119, 293.5832628385307999 ) ) ;
#13700=DIRECTION ( 'NONE',  ( 0.9396926207859126468, -0.3420201433256568890, 0.000000000000000000 ) ) ;
#13703=CYLINDRICAL_SURFACE ( 'NONE', #9959, 60.74260934110282051 ) ;
#13709=CARTESIAN_POINT ( 'NONE',  ( 45.84586732611860782, -36.66871011346395193, 110.7293897666001214 ) ) ;
#13710=CARTESIAN_POINT ( 'NONE',  ( -22.81000261549328911, 58.63718168490508020, 293.5832628385307999 ) ) ;
#13711=AXIS2_PLACEMENT_3D ( 'NONE', #5873, #12087, #10866 ) ;
#13713=ORIENTED_EDGE ( 'NONE', *, *, #13598, .F. ) ;
#13714=CARTESIAN_POINT ( 'NONE',  ( -8.938941455414985526, 60.08127757648384915, 283.5832628385307999 ) ) ;
#13715=CARTESIAN_POINT ( 'NONE',  ( 0.000000000000000000, 0.000000000000000000, 248.9926560891072143 ) ) ;
#13718=ORIENTED_EDGE ( 'NONE', *, *, #9887, .T. ) ;
#13719=ADVANCED_FACE ( 'NONE', ( #15724 ), #11006, .T. ) ;
#13721=FACE_BOUND ( 'NONE', #4063, .T. ) ;
#13722=VERTEX_POINT ( 'NONE', #1505 ) ;
#13723=VECTOR ( 'NONE', #9366, 1000.000000000000114 ) ;
#13727=CARTESIAN_POINT ( 'NONE',  ( 50.93469132750264095, 59.42266395395811429, 132.4711112102474146 ) ) ;
#13728=CARTESIAN_POINT ( 'NONE',  ( 9.564549117045082482, 62.18629025319818737, 248.9926560891072143 ) ) ;
#13729=PLANE ( 'NONE',  #1919 ) ;
#13730=VERTEX_POINT ( 'NONE', #6323 ) ;
#13731=LINE ( 'NONE', #17121, #12077 ) ;
#13735=LINE ( 'NONE', #1469, #16059 ) ;
#13738=ORIENTED_EDGE ( 'NONE', *, *, #11892, .F. ) ;
#13739=ADVANCED_FACE ( 'NONE', ( #8146 ), #18594, .F. ) ;
#13741=VECTOR ( 'NONE', #516, 1000.000000000000000 ) ;
#13744=ADVANCED_FACE ( 'NONE', ( #3147 ), #17473, .F. ) ;
#13745=ORIENTED_EDGE ( 'NONE', *, *, #3460, .T. ) ;
#13746=DIRECTION ( 'NONE',  ( 0.000000000000000000, -1.000000000000000000, 0.000000000000000000 ) ) ;
#13751=AXIS2_PLACEMENT_3D ( 'NONE', #11989, #6189, #4750 ) ;
#13753=CARTESIAN_POINT ( 'NONE',  ( -22.30005961346265408, -56.50329132715937419, 293.5832628385307999 ) ) ;
#13756=CARTESIAN_POINT ( 'NONE',  ( -41.02212542604614498, -44.79787735033404061, 283.5832628385307999 ) ) ;
#13759=EDGE_CURVE ( 'NONE', #1551, #18312, #17264, .T. ) ;
#13761=EDGE_CURVE ( 'NONE', #12874, #8815, #9583, .T. ) ;
#13762=EDGE_CURVE ( 'NONE', #15302, #18854, #15929, .T. ) ;
#13765=CARTESIAN_POINT ( 'NONE',  ( 59.51523122377253117, -12.14914984460739156, 283.5832628385307999 ) ) ;
#13766=EDGE_LOOP ( 'NONE', ( #10177, #14318, #2789, #8111 ) ) ;
#13769=ORIENTED_EDGE ( 'NONE', *, *, #15044, .F. ) ;
#13770=ORIENTED_EDGE ( 'NONE', *, *, #17268, .F. ) ;
#13772=EDGE_CURVE ( 'NONE', #15722, #3219, #4683, .T. ) ;
#13774=EDGE_LOOP ( 'NONE', ( #12121, #179, #8398 ) ) ;
#13778=DIRECTION ( 'NONE',  ( 0.000000000000000000, 0.000000000000000000, 1.000000000000000000 ) ) ;
#13779=EDGE_LOOP ( 'NONE', ( #5652, #3373, #17103 ) ) ;
#13784=CARTESIAN_POINT ( 'NONE',  ( 49.24833719034187851, 60.83768308848395634, 248.9926560891072143 ) ) ;
#13791=CARTESIAN_POINT ( 'NONE',  ( 2.605298826209745400, 5.111158570920780519, 293.5832628385307999 ) ) ;
#13792=EDGE_CURVE ( 'NONE', #2887, #19150, #14081, .T. ) ;
#13793=ORIENTED_EDGE ( 'NONE', *, *, #13214, .T. ) ;
#13795=LINE ( 'NONE', #18310, #8597 ) ;
#13798=ORIENTED_EDGE ( 'NONE', *, *, #5757, .F. ) ;
#13800=ORIENTED_EDGE ( 'NONE', *, *, #17919, .T. ) ;
#13801=CARTESIAN_POINT ( 'NONE',  ( 23.22641211976290876, 56.12662799072082720, 293.5832628385307999 ) ) ;
#13802=CARTESIAN_POINT ( 'NONE',  ( 27.53920554013639688, 73.25972925305639194, 248.9926560891072143 ) ) ;
#13805=AXIS2_PLACEMENT_3D ( 'NONE', #14121, #19049, #3486 ) ;
#13807=LINE ( 'NONE', #2773, #6379 ) ;
#13810=LINE ( 'NONE', #10942, #12880 ) ;
#13811=CARTESIAN_POINT ( 'NONE',  ( 40.27908801169993325, 45.46712722958823605, 283.5832628385307999 ) ) ;
#13813=DIRECTION ( 'NONE',  ( 0.000000000000000000, 0.000000000000000000, -1.000000000000000000 ) ) ;
#13815=ORIENTED_EDGE ( 'NONE', *, *, #11636, .T. ) ;
#13819=ORIENTED_EDGE ( 'NONE', *, *, #14946, .F. ) ;
#13820=ORIENTED_EDGE ( 'NONE', *, *, #14924, .T. ) ;
#13823=FACE_BOUND ( 'NONE', #11110, .T. ) ;
#13824=CIRCLE ( 'NONE', #14160, 62.91752772691707207 ) ;
#13825=ORIENTED_EDGE ( 'NONE', *, *, #10124, .F. ) ;
#13828=CARTESIAN_POINT ( 'NONE',  ( -54.89456854707563593, -30.74413178637172805, 132.4711112102474146 ) ) ;
#13832=DIRECTION ( 'NONE',  ( 0.4693298356057564180, -0.8830229359480272766, 0.000000000000000000 ) ) ;
#13834=CARTESIAN_POINT ( 'NONE',  ( 0.000000000000000000, 0.000000000000000000, 132.4711112102474146 ) ) ;
#13839=DIRECTION ( 'NONE',  ( 0.9848077530122103518, -0.1736481776669172583, 0.000000000000000000 ) ) ;
#13840=DIRECTION ( 'NONE',  ( 0.2080686897406943681, 0.9781142164131909622, 0.000000000000000000 ) ) ;
#13842=EDGE_CURVE ( 'NONE', #14032, #3122, #170, .T. ) ;
#13846=ORIENTED_EDGE ( 'NONE', *, *, #1677, .F. ) ;
#13847=ORIENTED_EDGE ( 'NONE', *, *, #11725, .F. ) ;
#13848=EDGE_CURVE ( 'NONE', #13023, #18959, #6116, .T. ) ;
#13851=EDGE_CURVE ( 'NONE', #6772, #11398, #9278, .T. ) ;
#13852=LINE ( 'NONE', #17040, #17791 ) ;
#13856=CARTESIAN_POINT ( 'NONE',  ( -76.83212392882501263, -14.94814811854935854, 132.4711112102474146 ) ) ;
#13860=DIRECTION ( 'NONE',  ( 1.000000000000000000, 0.000000000000000000, -0.000000000000000000 ) ) ;
#13863=CARTESIAN_POINT ( 'NONE',  ( 41.06890862491472660, 47.66508197439486594, 293.5832628385307999 ) ) ;
#13868=EDGE_LOOP ( 'NONE', ( #13388, #7581, #10514 ) ) ;
#13870=DIRECTION ( 'NONE',  ( 0.3420201433256757073, -0.9396926207859057634, 0.000000000000000000 ) ) ;
#13872=EDGE_LOOP ( 'NONE', ( #50, #7915, #2467, #12419 ) ) ;
#13873=DIRECTION ( 'NONE',  ( 1.000000000000000000, 0.000000000000000000, 0.000000000000000000 ) ) ;
#13875=VERTEX_POINT ( 'NONE', #3648 ) ;
#13876=EDGE_CURVE ( 'NONE', #8342, #4330, #19399, .T. ) ;
#13877=VECTOR ( 'NONE', #11926, 1000.000000000000114 ) ;
#13878=EDGE_CURVE ( 'NONE', #7889, #17522, #8240, .T. ) ;
#13879=DIRECTION ( 'NONE',  ( -0.3088643371590125697, 0.9511061040868803440, 0.000000000000000000 ) ) ;
#13880=DIRECTION ( 'NONE',  ( 1.000000000000000000, 0.000000000000000000, 0.000000000000000000 ) ) ;
#13881=DIRECTION ( 'NONE',  ( -0.000000000000000000, -0.000000000000000000, 1.000000000000000000 ) ) ;
#13882=ORIENTED_EDGE ( 'NONE', *, *, #5140, .F. ) ;
#13888=CARTESIAN_POINT ( 'NONE',  ( -40.27908801169994746, -45.46712722958822184, 283.5832628385307999 ) ) ;
#13890=ADVANCED_FACE ( 'NONE', ( #8546 ), #9878, .F. ) ;
#13894=VERTEX_POINT ( 'NONE', #5091 ) ;
#13896=CARTESIAN_POINT ( 'NONE',  ( 19.23677882349201695, -57.61823435390814296, 293.5832628385307999 ) ) ;
#13898=VERTEX_POINT ( 'NONE', #12846 ) ;
#13899=PLANE ( 'NONE',  #3225 ) ;
#13901=ORIENTED_EDGE ( 'NONE', *, *, #14997, .F. ) ;
#13903=EDGE_CURVE ( 'NONE', #7664, #4838, #9984, .T. ) ;
#13904=DIRECTION ( 'NONE',  ( 0.000000000000000000, 0.000000000000000000, -1.000000000000000000 ) ) ;
#13905=CARTESIAN_POINT ( 'NONE',  ( 0.000000000000000000, 0.000000000000000000, 283.5832628385307999 ) ) ;
#13906=VERTEX_POINT ( 'NONE', #13133 ) ;
#13907=AXIS2_PLACEMENT_3D ( 'NONE', #17174, #19921, #13985 ) ;
#13908=CARTESIAN_POINT ( 'NONE',  ( 0.000000000000000000, 0.000000000000000000, 132.4711112102474146 ) ) ;
#13909=DIRECTION ( 'NONE',  ( -0.9848077530122080203, -0.1736481776669306920, 0.000000000000000000 ) ) ;
#13910=EDGE_CURVE ( 'NONE', #18605, #15066, #17769, .T. ) ;
#13913=VERTEX_POINT ( 'NONE', #2317 ) ;
#13916=PLANE ( 'NONE',  #2373 ) ;
#13919=ORIENTED_EDGE ( 'NONE', *, *, #7764, .T. ) ;
#13920=VECTOR ( 'NONE', #14492, 1000.000000000000000 ) ;
#13925=ORIENTED_EDGE ( 'NONE', *, *, #18489, .F. ) ;
#13931=PLANE ( 'NONE',  #8908 ) ;
#13932=DIRECTION ( 'NONE',  ( -0.000000000000000000, -0.000000000000000000, 1.000000000000000000 ) ) ;
#13935=VECTOR ( 'NONE', #11571, 1000.000000000000227 ) ;
#13938=CARTESIAN_POINT ( 'NONE',  ( 53.87178215532755132, 28.06680738835045119, 293.5832628385307999 ) ) ;
#13940=CARTESIAN_POINT ( 'NONE',  ( 0.000000000000000000, 0.000000000000000000, 283.5832628385307999 ) ) ;
#13942=DIRECTION ( 'NONE',  ( -0.6692498792541777819, -0.7430374143461878633, 0.000000000000000000 ) ) ;
#13946=DIRECTION ( 'NONE',  ( -0.000000000000000000, -0.000000000000000000, 1.000000000000000000 ) ) ;
#13947=ORIENTED_EDGE ( 'NONE', *, *, #16884, .F. ) ;
#13948=EDGE_LOOP ( 'NONE', ( #13360, #4868, #1077, #12152 ) ) ;
#13949=SHAPE_REPRESENTATION ( 'MOTOR', ( #18639 ), #8174 ) ;
#13950=AXIS2_PLACEMENT_3D ( 'NONE', #1204, #12352, #4591 ) ;
#13951=ORIENTED_EDGE ( 'NONE', *, *, #19533, .T. ) ;
#13953=ADVANCED_FACE ( 'NONE', ( #3838 ), #14782, .F. ) ;
#13956=ORIENTED_EDGE ( 'NONE', *, *, #8135, .T. ) ;
#13959=ORIENTED_EDGE ( 'NONE', *, *, #19282, .F. ) ;
#13961=CARTESIAN_POINT ( 'NONE',  ( 39.37628763770421614, 49.07263256785966377, 248.9926560891072143 ) ) ;
#13962=CARTESIAN_POINT ( 'NONE',  ( -49.67518383744793908, 60.47951622432802310, 132.4711112102474146 ) ) ;
#13965=VECTOR ( 'NONE', #12855, 1000.000000000000114 ) ;
#13966=VECTOR ( 'NONE', #12324, 1000.000000000000000 ) ;
#13973=VERTEX_POINT ( 'NONE', #20093 ) ;
#13975=DIRECTION ( 'NONE',  ( -0.5000000000000039968, 0.8660254037844363761, 0.000000000000000000 ) ) ;
#13976=VERTEX_POINT ( 'NONE', #19788 ) ;
#13977=CARTESIAN_POINT ( 'NONE',  ( -55.43188410062182925, -19.30071112029661151, 132.4711112102474146 ) ) ;
#13978=CONICAL_SURFACE ( 'NONE', #6484, 79.75827554147308263, 0.5305858521701756203 ) ;
#13980=DIRECTION ( 'NONE',  ( -0.000000000000000000, -0.000000000000000000, 1.000000000000000000 ) ) ;
#13985=DIRECTION ( 'NONE',  ( 1.000000000000000000, 0.000000000000000000, 0.000000000000000000 ) ) ;
#13986=CARTESIAN_POINT ( 'NONE',  ( 62.90240729679780429, 1.379293853802413983, 132.4711112102474146 ) ) ;
#13987=EDGE_LOOP ( 'NONE', ( #4248, #3974, #11633 ) ) ;
#13988=LINE ( 'NONE', #18400, #7402 ) ;
#13989=DIRECTION ( 'NONE',  ( -0.000000000000000000, -0.000000000000000000, 1.000000000000000000 ) ) ;
#13990=LINE ( 'NONE', #6238, #17158 ) ;
#13993=DIRECTION ( 'NONE',  ( -0.000000000000000000, -0.000000000000000000, 1.000000000000000000 ) ) ;
#13995=LINE ( 'NONE', #9298, #4932 ) ;
#13997=VECTOR ( 'NONE', #6041, 1000.000000000000000 ) ;
#13999=VERTEX_POINT ( 'NONE', #16533 ) ;
#14002=DIRECTION ( 'NONE',  ( 0.3420201433256662704, 0.9396926207859092051, 0.000000000000000000 ) ) ;
#14005=DIRECTION ( 'NONE',  ( 1.000000000000000000, 0.000000000000000000, 0.000000000000000000 ) ) ;
#14008=EDGE_CURVE ( 'NONE', #15468, #3495, #7510, .T. ) ;
#14010=ORIENTED_EDGE ( 'NONE', *, *, #14431, .T. ) ;
#14012=DIRECTION ( 'NONE',  ( 0.6427876096865300370, 0.7660444431189858960, 0.000000000000000000 ) ) ;
#14013=VECTOR ( 'NONE', #159, 1000.000000000000000 ) ;
#14014=AXIS2_PLACEMENT_3D ( 'NONE', #997, #13463, #17380 ) ;
#14018=ORIENTED_EDGE ( 'NONE', *, *, #13330, .F. ) ;
#14019=DIRECTION ( 'NONE',  ( -0.000000000000000000, -0.000000000000000000, 1.000000000000000000 ) ) ;
#14020=CARTESIAN_POINT ( 'NONE',  ( -13.12769224524071277, -59.30917539369501412, 293.5832628385307999 ) ) ;
#14027=CARTESIAN_POINT ( 'NONE',  ( -14.94814811854910452, 76.83212392882505526, 112.0427633081291816 ) ) ;
#14028=FACE_OUTER_BOUND ( 'NONE', #12922, .T. ) ;
#14030=AXIS2_PLACEMENT_3D ( 'NONE', #2275, #629, #16086 ) ;
#14032=VERTEX_POINT ( 'NONE', #3528 ) ;
#14033=ORIENTED_EDGE ( 'NONE', *, *, #8974, .F. ) ;
#14040=APPLICATION_CONTEXT ( 'automotive_design' ) ;
#14041=CARTESIAN_POINT ( 'NONE',  ( 28.94983032429829350, -53.40245231972188833, 293.5832628385307999 ) ) ;
#14042=DIRECTION ( 'NONE',  ( -0.000000000000000000, -0.000000000000000000, 1.000000000000000000 ) ) ;
#14043=LINE ( 'NONE', #11172, #13534 ) ;
#14045=CARTESIAN_POINT ( 'NONE',  ( 62.18629025319813763, -9.564549117045302751, 248.9926560891072143 ) ) ;
#14046=FACE_OUTER_BOUND ( 'NONE', #15979, .T. ) ;
#14050=EDGE_CURVE ( 'NONE', #5404, #3300, #16011, .T. ) ;
#14051=CARTESIAN_POINT ( 'NONE',  ( -27.53920554013687649, -73.25972925305620720, 132.4711112102474146 ) ) ;
#14054=ORIENTED_EDGE ( 'NONE', *, *, #9526, .F. ) ;
#14057=VECTOR ( 'NONE', #17616, 1000.000000000000227 ) ;
#14059=ORIENTED_EDGE ( 'NONE', *, *, #9357, .F. ) ;
#14062=ORIENTED_EDGE ( 'NONE', *, *, #3994, .F. ) ;
#14065=LINE ( 'NONE', #10988, #3539 ) ;
#14067=VERTEX_POINT ( 'NONE', #11399 ) ;
#14068=DIRECTION ( 'NONE',  ( -0.000000000000000000, -0.000000000000000000, 1.000000000000000000 ) ) ;
#14069=CARTESIAN_POINT ( 'NONE',  ( 37.78325588002174840, -47.56406379474564972, 293.5832628385307999 ) ) ;
#14071=LINE ( 'NONE', #7621, #1669 ) ;
#14073=PLANE ( 'NONE',  #14306 ) ;
#14074=EDGE_LOOP ( 'NONE', ( #12049, #9427, #9392, #16523 ) ) ;
#14076=CARTESIAN_POINT ( 'NONE',  ( 59.51724408343574879, -12.14957802882732452, 293.5832628385307999 ) ) ;
#14078=ORIENTED_EDGE ( 'NONE', *, *, #17417, .T. ) ;
#14080=EDGE_LOOP ( 'NONE', ( #3557, #9402, #7064, #14582 ) ) ;
#14081=LINE ( 'NONE', #1705, #6326 ) ;
#14083=ORIENTED_EDGE ( 'NONE', *, *, #11158, .F. ) ;
#14084=LINE ( 'NONE', #172, #15907 ) ;
#14085=AXIS2_PLACEMENT_3D ( 'NONE', #7008, #955, #1050 ) ;
#14086=FACE_OUTER_BOUND ( 'NONE', #2016, .T. ) ;
#14090=ORIENTED_EDGE ( 'NONE', *, *, #12992, .F. ) ;
#14091=CARTESIAN_POINT ( 'NONE',  ( 0.000000000000000000, 0.000000000000000000, 293.5832628385307999 ) ) ;
#14097=CARTESIAN_POINT ( 'NONE',  ( -28.94886449118903826, 53.40063514825088475, 283.5832628385307999 ) ) ;
#14099=DIRECTION ( 'NONE',  ( -0.000000000000000000, -0.000000000000000000, 1.000000000000000000 ) ) ;
#14100=EDGE_LOOP ( 'NONE', ( #9412, #1325, #6601, #3234 ) ) ;
#14102=EDGE_CURVE ( 'NONE', #15888, #15836, #10065, .T. ) ;
#14104=ORIENTED_EDGE ( 'NONE', *, *, #8393, .F. ) ;
#14106=CARTESIAN_POINT ( 'NONE',  ( -38.35506425062487779, -44.43084819159262366, 248.9926560891072143 ) ) ;
#14107=ORIENTED_EDGE ( 'NONE', *, *, #16443, .F. ) ;
#14110=EDGE_CURVE ( 'NONE', #4841, #16766, #17653, .T. ) ;
#14111=DIRECTION ( 'NONE',  ( 1.000000000000000000, 0.000000000000000000, 0.000000000000000000 ) ) ;
#14113=EDGE_CURVE ( 'NONE', #13644, #18605, #6995, .T. ) ;
#14115=FACE_OUTER_BOUND ( 'NONE', #17176, .T. ) ;
#14116=EDGE_CURVE ( 'NONE', #20199, #48, #8323, .T. ) ;
#14118=DIRECTION ( 'NONE',  ( 0.8479630283625716469, -0.5300553768524345344, 0.000000000000000000 ) ) ;
#14119=CARTESIAN_POINT ( 'NONE',  ( 55.43188410062170135, 19.30071112029698455, 111.4180192758973362 ) ) ;
#14120=ORIENTED_EDGE ( 'NONE', *, *, #15819, .T. ) ;
#14121=CARTESIAN_POINT ( 'NONE',  ( 0.000000000000000000, 0.000000000000000000, 293.5832628385307999 ) ) ;
#14122=CYLINDRICAL_SURFACE ( 'NONE', #10039, 62.91752772691707207 ) ;
#14124=VERTEX_POINT ( 'NONE', #16411 ) ;
#14125=EDGE_CURVE ( 'NONE', #12122, #1787, #6803, .T. ) ;
#14126=CARTESIAN_POINT ( 'NONE',  ( 31.77187437101505196, 51.77076963420834232, 283.5832628385307999 ) ) ;
#14130=EDGE_LOOP ( 'NONE', ( #14324, #16509, #16633 ) ) ;
#14132=CIRCLE ( 'NONE', #6624, 62.91752772691707207 ) ;
#14134=EDGE_LOOP ( 'NONE', ( #6745, #2386, #4111 ) ) ;
#14135=DIRECTION ( 'NONE',  ( -0.000000000000000000, -0.000000000000000000, 1.000000000000000000 ) ) ;
#14136=CARTESIAN_POINT ( 'NONE',  ( -13.12769224524071277, -59.30917539369501412, 293.5832628385307999 ) ) ;
#14139=CIRCLE ( 'NONE', #10526, 62.91752772691707207 ) ;
#14143=EDGE_CURVE ( 'NONE', #19280, #12693, #14171, .T. ) ;
#14147=CARTESIAN_POINT ( 'NONE',  ( -37.93579148621510200, -68.46530598706782200, 248.9926560891072143 ) ) ;
#14148=PLANE ( 'NONE',  #15196 ) ;
#14150=VECTOR ( 'NONE', #18227, 1000.000000000000114 ) ;
#14152=PLANE ( 'NONE',  #374 ) ;
#14153=DIRECTION ( 'NONE',  ( -0.3420201433256568335, -0.9396926207859127578, 0.000000000000000000 ) ) ;
#14155=ORIENTED_EDGE ( 'NONE', *, *, #97, .T. ) ;
#14156=EDGE_CURVE ( 'NONE', #2515, #14853, #18753, .T. ) ;
#14160=AXIS2_PLACEMENT_3D ( 'NONE', #16986, #17196, #2971 ) ;
#14163=VERTEX_POINT ( 'NONE', #13619 ) ;
#14169=DIRECTION ( 'NONE',  ( -0.000000000000000000, -0.000000000000000000, 1.000000000000000000 ) ) ;
#14170=FACE_OUTER_BOUND ( 'NONE', #2411, .T. ) ;
#14171=CIRCLE ( 'NONE', #122, 60.74260934110282051 ) ;
#14173=CARTESIAN_POINT ( 'NONE',  ( 0.000000000000000000, 0.000000000000000000, 293.5832628385307999 ) ) ;
#14177=DIRECTION ( 'NONE',  ( 0.03505990758545895342, 0.9993852124581886764, 0.000000000000000000 ) ) ;
#14184=ORIENTED_EDGE ( 'NONE', *, *, #16048, .T. ) ;
#14186=VERTEX_POINT ( 'NONE', #9017 ) ;
#14188=CARTESIAN_POINT ( 'NONE',  ( 30.53958573130908505, -50.13752642112839197, 132.4711112102474146 ) ) ;
#14189=AXIS2_PLACEMENT_3D ( 'NONE', #9858, #16110, #11687 ) ;
#14191=DIRECTION ( 'NONE',  ( 0.000000000000000000, 0.000000000000000000, 1.000000000000000000 ) ) ;
#14192=PLANE ( 'NONE',  #8598 ) ;
#14198=DIRECTION ( 'NONE',  ( -1.000000000000000000, -3.491481338843133355E-15, -0.000000000000000000 ) ) ;
#14199=ORIENTED_EDGE ( 'NONE', *, *, #11850, .F. ) ;
#14201=DIRECTION ( 'NONE',  ( -0.000000000000000000, -0.000000000000000000, 1.000000000000000000 ) ) ;
#14206=ORIENTED_EDGE ( 'NONE', *, *, #18645, .F. ) ;
#14207=DIRECTION ( 'NONE',  ( -0.9902903945359630145, -0.1390141521205912334, 0.000000000000000000 ) ) ;
#14214=DIRECTION ( 'NONE',  ( 1.000000000000000000, 0.000000000000000000, 0.000000000000000000 ) ) ;
#14215=LINE ( 'NONE', #198, #9926 ) ;
#14217=( NAMED_UNIT ( * ) SI_UNIT ( $, .STERADIAN. ) SOLID_ANGLE_UNIT ( ) );
#14218=CARTESIAN_POINT ( 'NONE',  ( 0.000000000000000000, 0.000000000000000000, 283.5832628385307999 ) ) ;
#14219=EDGE_CURVE ( 'NONE', #5361, #1451, #2489, .T. ) ;
#14224=CARTESIAN_POINT ( 'NONE',  ( 0.000000000000000000, 0.000000000000000000, 132.4711112102474146 ) ) ;
#14226=DIRECTION ( 'NONE',  ( 0.000000000000000000, 0.000000000000000000, 1.000000000000000000 ) ) ;
#14227=DIRECTION ( 'NONE',  ( 1.000000000000000000, 0.000000000000000000, 0.000000000000000000 ) ) ;
#14232=LINE ( 'NONE', #12994, #9755 ) ;
#14234=EDGE_CURVE ( 'NONE', #48, #18696, #8719, .T. ) ;
#14235=ORIENTED_EDGE ( 'NONE', *, *, #11397, .T. ) ;
#14238=EDGE_CURVE ( 'NONE', #4139, #12303, #5967, .T. ) ;
#14241=ORIENTED_EDGE ( 'NONE', *, *, #19969, .T. ) ;
#14244=ORIENTED_EDGE ( 'NONE', *, *, #786, .T. ) ;
#14245=DIRECTION ( 'NONE',  ( 0.6427876096865300370, 0.7660444431189858960, 0.000000000000000000 ) ) ;
#14250=CARTESIAN_POINT ( 'NONE',  ( 59.30917539369505675, -13.12769224524051559, 293.5832628385307999 ) ) ;
#14253=LINE ( 'NONE', #11579, #3416 ) ;
#14255=CARTESIAN_POINT ( 'NONE',  ( -57.92514141135453087, -18.28503710798565507, 283.5832628385307999 ) ) ;
#14259=EDGE_CURVE ( 'NONE', #11013, #12611, #12079, .T. ) ;
#14263=ORIENTED_EDGE ( 'NONE', *, *, #6874, .F. ) ;
#14264=VECTOR ( 'NONE', #12140, 1000.000000000000114 ) ;
#14265=VERTEX_POINT ( 'NONE', #18760 ) ;
#14270=EDGE_CURVE ( 'NONE', #17256, #6775, #4741, .T. ) ;
#14271=LINE ( 'NONE', #1689, #17133 ) ;
#14272=LINE ( 'NONE', #253, #14316 ) ;
#14274=ORIENTED_EDGE ( 'NONE', *, *, #19474, .T. ) ;
#14275=CYLINDRICAL_SURFACE ( 'NONE', #6513, 62.91752772691707207 ) ;
#14276=LINE ( 'NONE', #3331, #19992 ) ;
#14277=DIRECTION ( 'NONE',  ( -0.7881095627315599650, -0.6155349844899714595, 0.000000000000000000 ) ) ;
#14278=FACE_OUTER_BOUND ( 'NONE', #6840, .T. ) ;
#14280=VECTOR ( 'NONE', #6001, 1000.000000000000000 ) ;
#14281=EDGE_LOOP ( 'NONE', ( #9734, #9783, #366 ) ) ;
#14282=EDGE_CURVE ( 'NONE', #15923, #7403, #18545, .T. ) ;
#14285=DIRECTION ( 'NONE',  ( -0.000000000000000000, -0.000000000000000000, 1.000000000000000000 ) ) ;
#14286=EDGE_CURVE ( 'NONE', #3178, #18381, #15473, .T. ) ;
#14287=ORIENTED_EDGE ( 'NONE', *, *, #16525, .T. ) ;
#14288=VECTOR ( 'NONE', #11744, 1000.000000000000114 ) ;
#14293=DIRECTION ( 'NONE',  ( 0.3747554100459959958, 0.9271237148521535021, 0.000000000000000000 ) ) ;
#14294=ADVANCED_FACE ( 'NONE', ( #12598 ), #7801, .F. ) ;
#14295=ORIENTED_EDGE ( 'NONE', *, *, #13385, .T. ) ;
#14298=FACE_OUTER_BOUND ( 'NONE', #14465, .T. ) ;
#14299=CARTESIAN_POINT ( 'NONE',  ( -44.79787735033389851, 41.02212542604627998, 283.5832628385307999 ) ) ;
#14303=VECTOR ( 'NONE', #4792, 1000.000000000000114 ) ;
#14306=AXIS2_PLACEMENT_3D ( 'NONE', #18692, #2933, #9163 ) ;
#14309=PLANE ( 'NONE',  #3106 ) ;
#14313=ORIENTED_EDGE ( 'NONE', *, *, #6, .T. ) ;
#14314=LINE ( 'NONE', #16257, #13166 ) ;
#14315=ORIENTED_EDGE ( 'NONE', *, *, #13330, .T. ) ;
#14316=VECTOR ( 'NONE', #4971, 1000.000000000000000 ) ;
#14317=EDGE_CURVE ( 'NONE', #15888, #16227, #1767, .T. ) ;
#14318=ORIENTED_EDGE ( 'NONE', *, *, #13128, .T. ) ;
#14319=DIRECTION ( 'NONE',  ( 0.8660254037844345998, 0.5000000000000069944, 0.000000000000000000 ) ) ;
#14320=VECTOR ( 'NONE', #15511, 1000.000000000000000 ) ;
#14321=ORIENTED_EDGE ( 'NONE', *, *, #5614, .F. ) ;
#14323=PLANE ( 'NONE',  #5034 ) ;
#14324=ORIENTED_EDGE ( 'NONE', *, *, #18046, .T. ) ;
#14325=FILL_AREA_STYLE_COLOUR ( '', #2808 ) ;
#14328=VECTOR ( 'NONE', #8769, 1000.000000000000000 ) ;
#14333=ORIENTED_EDGE ( 'NONE', *, *, #13591, .F. ) ;
#14334=DIRECTION ( 'NONE',  ( -0.7660444431189726844, -0.6427876096865456912, 0.000000000000000000 ) ) ;
#14342=EDGE_CURVE ( 'NONE', #3335, #5555, #4529, .T. ) ;
#14343=ORIENTED_EDGE ( 'NONE', *, *, #348, .T. ) ;
#14349=DIRECTION ( 'NONE',  ( 0.5300553768524375320, 0.8479630283625697595, 0.000000000000000000 ) ) ;
#14350=LINE ( 'NONE', #11166, #16245 ) ;
#14352=FACE_OUTER_BOUND ( 'NONE', #10304, .T. ) ;
#14353=CARTESIAN_POINT ( 'NONE',  ( -1.289614712049159007, 5.590028426173815568, 293.5832628385307999 ) ) ;
#14354=CARTESIAN_POINT ( 'NONE',  ( -76.92888220842476699, 14.39940464655786201, 248.9926560891072143 ) ) ;
#14358=CYLINDRICAL_SURFACE ( 'NONE', #18767, 62.91752772691707207 ) ;
#14361=CYLINDRICAL_SURFACE ( 'NONE', #9843, 60.74260934110282051 ) ;
#14364=AXIS2_PLACEMENT_3D ( 'NONE', #12759, #16241, #19212 ) ;
#14365=VERTEX_POINT ( 'NONE', #4953 ) ;
#14366=DIRECTION ( 'NONE',  ( 0.000000000000000000, 0.000000000000000000, 1.000000000000000000 ) ) ;
#14367=EDGE_CURVE ( 'NONE', #998, #9378, #8298, .T. ) ;
#14370=ORIENTED_EDGE ( 'NONE', *, *, #15155, .F. ) ;
#14371=CIRCLE ( 'NONE', #319, 62.91752772691707207 ) ;
#14376=CARTESIAN_POINT ( 'NONE',  ( -1.379293853801755176, 62.90240729679781850, 132.4711112102474146 ) ) ;
#14377=EDGE_CURVE ( 'NONE', #2297, #10955, #10860, .T. ) ;
#14379=CARTESIAN_POINT ( 'NONE',  ( -0.4239815141812765531, 0.2650276884262135479, 283.5832628385307999 ) ) ;
#14380=DIRECTION ( 'NONE',  ( -0.000000000000000000, -0.000000000000000000, 1.000000000000000000 ) ) ;
#14388=VERTEX_POINT ( 'NONE', #3102 ) ;
#14389=EDGE_CURVE ( 'NONE', #15683, #13913, #9334, .T. ) ;
#14392=ORIENTED_EDGE ( 'NONE', *, *, #8347, .F. ) ;
#14394=DIRECTION ( 'NONE',  ( -0.6427876096865328126, -0.7660444431189835646, 0.000000000000000000 ) ) ;
#14397=ORIENTED_EDGE ( 'NONE', *, *, #13406, .T. ) ;
#14401=CARTESIAN_POINT ( 'NONE',  ( 1.379293853801755176, -78.26059000578311498, 132.4711112102474146 ) ) ;
#14402=ADVANCED_FACE ( 'NONE', ( #17332 ), #9736, .F. ) ;
#14403=ORIENTED_EDGE ( 'NONE', *, *, #14857, .T. ) ;
#14405=CARTESIAN_POINT ( 'NONE',  ( 0.000000000000000000, 0.000000000000000000, 283.5832628385307999 ) ) ;
#14406=PLANE ( 'NONE',  #16372 ) ;
#14407=DIRECTION ( 'NONE',  ( 0.000000000000000000, 0.000000000000000000, 1.000000000000000000 ) ) ;
#14410=CARTESIAN_POINT ( 'NONE',  ( 2.629250726500717672, 60.68567895461850981, 283.5832628385307999 ) ) ;
#14413=EDGE_CURVE ( 'NONE', #6318, #16710, #5710, .T. ) ;
#14414=CARTESIAN_POINT ( 'NONE',  ( 0.000000000000000000, 0.000000000000000000, 283.5832628385307999 ) ) ;
#14420=ORIENTED_EDGE ( 'NONE', *, *, #5875, .F. ) ;
#14422=DIRECTION ( 'NONE',  ( 0.1390141521205946196, -0.9902903945359624593, 0.000000000000000000 ) ) ;
#14423=ORIENTED_EDGE ( 'NONE', *, *, #12083, .T. ) ;
#14424=EDGE_CURVE ( 'NONE', #11394, #6348, #19071, .T. ) ;
#14425=CARTESIAN_POINT ( 'NONE',  ( -5.111158570922238020, 2.605298826210300511, 293.5832628385307999 ) ) ;
#14427=CARTESIAN_POINT ( 'NONE',  ( -31.77296517111735596, -51.77251465595229263, 293.5832628385307999 ) ) ;
#14428=VECTOR ( 'NONE', #19868, 1000.000000000000000 ) ;
#14429=CARTESIAN_POINT ( 'NONE',  ( 0.000000000000000000, 0.000000000000000000, 132.4711112102474146 ) ) ;
#14430=VECTOR ( 'NONE', #14943, 1000.000000000000114 ) ;
#14431=EDGE_CURVE ( 'NONE', #219, #16961, #6879, .T. ) ;
#14432=CARTESIAN_POINT ( 'NONE',  ( 18.77710619359078947, 55.62246070845787216, 132.4711112102474146 ) ) ;
#14433=CARTESIAN_POINT ( 'NONE',  ( -58.83691981461618781, 22.28973221005139749, 132.4711112102474146 ) ) ;
#14434=DIRECTION ( 'NONE',  ( 0.6427876096865456912, -0.7660444431189726844, 0.000000000000000000 ) ) ;
#14435=DIRECTION ( 'NONE',  ( -0.000000000000000000, -0.000000000000000000, 1.000000000000000000 ) ) ;
#14436=CARTESIAN_POINT ( 'NONE',  ( 60.72279549541555355, -1.629937663769388090, 293.5832628385307999 ) ) ;
#14438=VERTEX_POINT ( 'NONE', #14353 ) ;
#14439=DIRECTION ( 'NONE',  ( 1.000000000000000000, 0.000000000000000000, 0.000000000000000000 ) ) ;
#14441=ORIENTED_EDGE ( 'NONE', *, *, #2363, .F. ) ;
#14443=ORIENTED_EDGE ( 'NONE', *, *, #12233, .F. ) ;
#14446=LINE ( 'NONE', #17530, #5224 ) ;
#14456=FACE_OUTER_BOUND ( 'NONE', #12378, .T. ) ;
#14461=VECTOR ( 'NONE', #11181, 1000.000000000000000 ) ;
#14464=ORIENTED_EDGE ( 'NONE', *, *, #1083, .T. ) ;
#14465=EDGE_LOOP ( 'NONE', ( #11836, #1757, #16388, #10152 ) ) ;
#14467=DIRECTION ( 'NONE',  ( 0.9396926207859046531, 0.3420201433256790380, 0.000000000000000000 ) ) ;
#14469=DIRECTION ( 'NONE',  ( -0.000000000000000000, -0.000000000000000000, 1.000000000000000000 ) ) ;
#14470=CIRCLE ( 'NONE', #19686, 17.50000000000001066 ) ;
#14472=EDGE_CURVE ( 'NONE', #2129, #18497, #11274, .T. ) ;
#14473=DIRECTION ( 'NONE',  ( -0.000000000000000000, -0.000000000000000000, 1.000000000000000000 ) ) ;
#14474=LINE ( 'NONE', #17661, #1706 ) ;
#14475=DIRECTION ( 'NONE',  ( 0.1390141521205912056, -0.9902903945359629034, 0.000000000000000000 ) ) ;
#14476=AXIS2_PLACEMENT_3D ( 'NONE', #12438, #9680, #11109 ) ;
#14479=VERTEX_POINT ( 'NONE', #728 ) ;
#14480=EDGE_CURVE ( 'NONE', #10368, #675, #5056, .T. ) ;
#14481=FACE_OUTER_BOUND ( 'NONE', #14134, .T. ) ;
#14487=EDGE_CURVE ( 'NONE', #9275, #5133, #14508, .T. ) ;
#14488=ORIENTED_EDGE ( 'NONE', *, *, #639, .F. ) ;
#14490=DIRECTION ( 'NONE',  ( -0.1390141521205912334, 0.9902903945359629034, 0.000000000000000000 ) ) ;
#14492=DIRECTION ( 'NONE',  ( -0.000000000000000000, -0.000000000000000000, 1.000000000000000000 ) ) ;
#14495=CARTESIAN_POINT ( 'NONE',  ( -3.453261854572980738, -4.581103194069957141, 293.5832628385307999 ) ) ;
#14498=ORIENTED_EDGE ( 'NONE', *, *, #4589, .F. ) ;
#14500=LINE ( 'NONE', #6634, #19574 ) ;
#14502=ORIENTED_EDGE ( 'NONE', *, *, #15234, .T. ) ;
#14503=LINE ( 'NONE', #11222, #859 ) ;
#14505=CARTESIAN_POINT ( 'NONE',  ( -11.73417718768092044, -61.81362617575096152, 293.5832628385307999 ) ) ;
#14506=CARTESIAN_POINT ( 'NONE',  ( 59.51523122377252406, -12.14914984460739156, 293.5832628385307999 ) ) ;
#14508=CIRCLE ( 'NONE', #11568, 60.74260934110282051 ) ;
#14511=VERTEX_POINT ( 'NONE', #9944 ) ;
#14513=VECTOR ( 'NONE', #868, 1000.000000000000000 ) ;
#14514=EDGE_LOOP ( 'NONE', ( #17673, #10851, #6963, #1832 ) ) ;
#14516=ORIENTED_EDGE ( 'NONE', *, *, #16393, .T. ) ;
#14521=DIRECTION ( 'NONE',  ( 0.000000000000000000, 0.000000000000000000, 1.000000000000000000 ) ) ;
#14522=VECTOR ( 'NONE', #11742, 1000.000000000000000 ) ;
#14525=LINE ( 'NONE', #17016, #369 ) ;
#14526=EDGE_CURVE ( 'NONE', #13023, #15125, #7309, .T. ) ;
#14527=CARTESIAN_POINT ( 'NONE',  ( 0.000000000000000000, 0.000000000000000000, 248.9926560891072143 ) ) ;
#14528=CARTESIAN_POINT ( 'NONE',  ( -60.22029172860437285, -7.948651060879224239, 283.5832628385307999 ) ) ;
#14529=FACE_OUTER_BOUND ( 'NONE', #4285, .T. ) ;
#14532=FACE_OUTER_BOUND ( 'NONE', #4831, .T. ) ;
#14533=AXIS2_PLACEMENT_3D ( 'NONE', #1977, #10861, #7898 ) ;
#14534=CARTESIAN_POINT ( 'NONE',  ( 45.46712722958809394, -40.27908801170008246, 283.5832628385307999 ) ) ;
#14536=CARTESIAN_POINT ( 'NONE',  ( -32.16802499836779106, -54.07248341783242296, 293.5832628385307999 ) ) ;
#14538=EDGE_CURVE ( 'NONE', #12174, #12822, #16194, .T. ) ;
#14541=ADVANCED_FACE ( 'NONE', ( #15994 ), #14358, .T. ) ;
#14542=EDGE_LOOP ( 'NONE', ( #14441, #7329, #15772, #14712 ) ) ;
#14544=EDGE_LOOP ( 'NONE', ( #653, #18207, #16602, #8943 ) ) ;
#14545=ADVANCED_FACE ( 'NONE', ( #13103 ), #6690, .F. ) ;
#14546=CARTESIAN_POINT ( 'NONE',  ( -28.06281046684226155, 73.06915264522029929, 248.9926560891072143 ) ) ;
#14548=ORIENTED_EDGE ( 'NONE', *, *, #12105, .T. ) ;
#14549=EDGE_CURVE ( 'NONE', #5714, #16297, #14253, .T. ) ;
#14550=AXIS2_PLACEMENT_3D ( 'NONE', #14218, #6354, #12573 ) ;
#14552=CARTESIAN_POINT ( 'NONE',  ( 0.000000000000000000, 0.000000000000000000, 283.5832628385307999 ) ) ;
#14556=FACE_OUTER_BOUND ( 'NONE', #6126, .T. ) ;
#14558=CARTESIAN_POINT ( 'NONE',  ( -48.17797692984162694, -36.99387960884178739, 283.5832628385307999 ) ) ;
#14561=CARTESIAN_POINT ( 'NONE',  ( -27.53920554013687649, -73.25972925305620720, 248.9926560891072143 ) ) ;
#14562=DIRECTION ( 'NONE',  ( 0.000000000000000000, 0.000000000000000000, -1.000000000000000000 ) ) ;
#14565=CARTESIAN_POINT ( 'NONE',  ( -30.25670013172253192, -55.16472960512360402, 132.4711112102474146 ) ) ;
#14566=VERTEX_POINT ( 'NONE', #12710 ) ;
#14568=VERTEX_POINT ( 'NONE', #1983 ) ;
#14569=CARTESIAN_POINT ( 'NONE',  ( 60.47951622432751151, 49.67518383744852883, 132.4711112102474146 ) ) ;
#14570=AXIS2_PLACEMENT_3D ( 'NONE', #13449, #10167, #14768 ) ;
#14572=DIRECTION ( 'NONE',  ( 0.6155349844899715706, -0.7881095627315598540, 0.000000000000000000 ) ) ;
#14573=CARTESIAN_POINT ( 'NONE',  ( 27.53920554013639688, 73.25972925305639194, 248.9926560891072143 ) ) ;
#14578=CARTESIAN_POINT ( 'NONE',  ( -2.629322876227788264, -60.68773558783006905, 293.5832628385307999 ) ) ;
#14579=CARTESIAN_POINT ( 'NONE',  ( 58.69016442926520938, 1.379293853802370018, 132.4711112102474146 ) ) ;
#14582=ORIENTED_EDGE ( 'NONE', *, *, #3980, .F. ) ;
#14583=CIRCLE ( 'NONE', #12602, 62.91752772691707207 ) ;
#14584=ORIENTED_EDGE ( 'NONE', *, *, #4270, .F. ) ;
#14585=ORIENTED_EDGE ( 'NONE', *, *, #15036, .F. ) ;
#14586=VERTEX_POINT ( 'NONE', #8209 ) ;
#14587=ORIENTED_EDGE ( 'NONE', *, *, #17892, .T. ) ;
#14592=CARTESIAN_POINT ( 'NONE',  ( -56.12662799072088404, 23.22641211976270625, 293.5832628385307999 ) ) ;
#14593=DIRECTION ( 'NONE',  ( 0.8660254037844328234, 0.5000000000000101030, 0.000000000000000000 ) ) ;
#14594=EDGE_LOOP ( 'NONE', ( #6722, #4557, #9045, #18060 ) ) ;
#14595=CARTESIAN_POINT ( 'NONE',  ( 54.86954475316255042, -20.84572577951183092, 248.9926560891072143 ) ) ;
#14601=LINE ( 'NONE', #11622, #11637 ) ;
#14602=DIRECTION ( 'NONE',  ( 1.000000000000000000, 0.000000000000000000, 0.000000000000000000 ) ) ;
#14604=ADVANCED_FACE ( 'NONE', ( #5159 ), #1775, .F. ) ;
#14610=ORIENTED_EDGE ( 'NONE', *, *, #5611, .T. ) ;
#14612=VERTEX_POINT ( 'NONE', #17439 ) ;
#14613=ORIENTED_EDGE ( 'NONE', *, *, #12717, .F. ) ;
#14616=ORIENTED_EDGE ( 'NONE', *, *, #2510, .T. ) ;
#14617=LINE ( 'NONE', #12779, #1588 ) ;
#14624=CARTESIAN_POINT ( 'NONE',  ( 0.000000000000000000, 0.000000000000000000, 293.5832628385307999 ) ) ;
#14625=CARTESIAN_POINT ( 'NONE',  ( 0.000000000000000000, 0.000000000000000000, 283.5832628385307999 ) ) ;
#14626=CARTESIAN_POINT ( 'NONE',  ( -10.11498556985118746, 62.09913334491134407, 293.5832628385307999 ) ) ;
#14627=ADVANCED_FACE ( 'NONE', ( #3903 ), #8899, .F. ) ;
#14628=CARTESIAN_POINT ( 'NONE',  ( 8.939227532413712041, -60.08331549348429235, 293.5832628385307999 ) ) ;
#14631=CYLINDRICAL_SURFACE ( 'NONE', #6881, 62.91752772691707207 ) ;
#14634=ORIENTED_EDGE ( 'NONE', *, *, #15234, .F. ) ;
#14636=CARTESIAN_POINT ( 'NONE',  ( 62.18629025319814474, -9.564549117045300974, 132.4711112102474146 ) ) ;
#14637=CARTESIAN_POINT ( 'NONE',  ( -5.693982670708919613, 0.7000608949449669272, 283.5832628385307999 ) ) ;
#14641=EDGE_CURVE ( 'NONE', #1866, #7218, #19749, .T. ) ;
#14643=FACE_OUTER_BOUND ( 'NONE', #1701, .T. ) ;
#14644=DIRECTION ( 'NONE',  ( -0.3420201433256694901, 0.9396926207859082059, 0.000000000000000000 ) ) ;
#14645=ORIENTED_EDGE ( 'NONE', *, *, #10704, .F. ) ;
#14646=CARTESIAN_POINT ( 'NONE',  ( -47.29944656917786006, -41.48948842197101783, 248.9926560891072143 ) ) ;
#14647=CARTESIAN_POINT ( 'NONE',  ( -25.99419088092141550, 73.82206860051556419, 248.9926560891072143 ) ) ;
#14650=VECTOR ( 'NONE', #1586, 1000.000000000000114 ) ;
#14652=EDGE_CURVE ( 'NONE', #17581, #11236, #6978, .T. ) ;
#14655=EDGE_CURVE ( 'NONE', #17978, #8052, #930, .T. ) ;
#14656=DIRECTION ( 'NONE',  ( 1.000000000000000000, 0.000000000000000000, 0.000000000000000000 ) ) ;
#14658=DIRECTION ( 'NONE',  ( -0.8830229359480271656, -0.4693298356057563625, 0.000000000000000000 ) ) ;
#14663=AXIS2_PLACEMENT_3D ( 'NONE', #10932, #9511, #15548 ) ;
#14665=CIRCLE ( 'NONE', #4878, 62.91752772691707207 ) ;
#14668=ORIENTED_EDGE ( 'NONE', *, *, #8998, .F. ) ;
#14669=DIRECTION ( 'NONE',  ( 1.000000000000000000, 0.000000000000000000, 0.000000000000000000 ) ) ;
#14672=ADVANCED_FACE ( 'NONE', ( #17934 ), #13294, .F. ) ;
#14674=VECTOR ( 'NONE', #13057, 999.9999999999998863 ) ;
#14682=CARTESIAN_POINT ( 'NONE',  ( 0.000000000000000000, 0.000000000000000000, 248.9926560891072143 ) ) ;
#14686=ORIENTED_EDGE ( 'NONE', *, *, #16637, .F. ) ;
#14687=AXIS2_PLACEMENT_3D ( 'NONE', #5340, #6875, #820 ) ;
#14688=CIRCLE ( 'NONE', #5871, 65.74260934110282051 ) ;
#14690=ORIENTED_EDGE ( 'NONE', *, *, #19854, .F. ) ;
#14691=PLANE ( 'NONE',  #6967 ) ;
#14692=PLANE ( 'NONE',  #6698 ) ;
#14693=DIRECTION ( 'NONE',  ( 0.000000000000000000, 0.000000000000000000, -1.000000000000000000 ) ) ;
#14694=ORIENTED_EDGE ( 'NONE', *, *, #5733, .F. ) ;
#14695=CARTESIAN_POINT ( 'NONE',  ( -8.938941455414980197, 60.08127757648381362, 283.5832628385307999 ) ) ;
#14698=DIRECTION ( 'NONE',  ( -0.000000000000000000, -0.000000000000000000, 1.000000000000000000 ) ) ;
#14699=FACE_OUTER_BOUND ( 'NONE', #19914, .T. ) ;
#14700=CARTESIAN_POINT ( 'NONE',  ( 0.000000000000000000, 0.000000000000000000, 248.9926560891072143 ) ) ;
#14701=CARTESIAN_POINT ( 'NONE',  ( -38.78191089773041256, 44.07268132743711675, 132.4711112102474146 ) ) ;
#14710=DIRECTION ( 'NONE',  ( 1.000000000000000000, 0.000000000000000000, 0.000000000000000000 ) ) ;
#14711=ORIENTED_EDGE ( 'NONE', *, *, #4227, .T. ) ;
#14712=ORIENTED_EDGE ( 'NONE', *, *, #9209, .T. ) ;
#14718=EDGE_LOOP ( 'NONE', ( #19984, #13418, #15209 ) ) ;
#14719=DIRECTION ( 'NONE',  ( -0.000000000000000000, -0.000000000000000000, 1.000000000000000000 ) ) ;
#14720=DIRECTION ( 'NONE',  ( -0.000000000000000000, -0.000000000000000000, 1.000000000000000000 ) ) ;
#14722=LINE ( 'NONE', #14528, #13741 ) ;
#14723=FACE_OUTER_BOUND ( 'NONE', #624, .T. ) ;
#14724=AXIS2_PLACEMENT_3D ( 'NONE', #11333, #17589, #2033 ) ;
#14727=CARTESIAN_POINT ( 'NONE',  ( -60.08127757648377099, -8.938941455415186255, 293.5832628385307999 ) ) ;
#14729=AXIS2_PLACEMENT_3D ( 'NONE', #15509, #4773, #17252 ) ;
#14731=ORIENTED_EDGE ( 'NONE', *, *, #18119, .F. ) ;
#14733=DIRECTION ( 'NONE',  ( 1.000000000000000000, 0.000000000000000000, 0.000000000000000000 ) ) ;
#14734=ORIENTED_EDGE ( 'NONE', *, *, #1997, .F. ) ;
#14735=EDGE_LOOP ( 'NONE', ( #8236, #2850, #5139, #10108 ) ) ;
#14738=ADVANCED_FACE ( 'NONE', ( #7079 ), #19847, .T. ) ;
#14741=ADVANCED_FACE ( 'NONE', ( #5543 ), #1026, .F. ) ;
#14743=LINE ( 'NONE', #1020, #9371 ) ;
#14744=ORIENTED_EDGE ( 'NONE', *, *, #5915, .T. ) ;
#14752=DIRECTION ( 'NONE',  ( 0.9848077530122080203, 0.1736481776669307198, 0.000000000000000000 ) ) ;
#14755=VERTEX_POINT ( 'NONE', #13197 ) ;
#14758=EDGE_CURVE ( 'NONE', #3694, #5829, #18029, .T. ) ;
#14760=ADVANCED_FACE ( 'NONE', ( #14939 ), #13498, .F. ) ;
#14763=DIRECTION ( 'NONE',  ( -0.000000000000000000, -0.000000000000000000, 1.000000000000000000 ) ) ;
#14767=DIRECTION ( 'NONE',  ( -0.7881095627315599650, -0.6155349844899714595, 0.000000000000000000 ) ) ;
#14768=DIRECTION ( 'NONE',  ( 1.000000000000000000, 0.000000000000000000, 0.000000000000000000 ) ) ;
#14771=VECTOR ( 'NONE', #11487, 1000.000000000000000 ) ;
#14774=LINE ( 'NONE', #10359, #17572 ) ;
#14775=VERTEX_POINT ( 'NONE', #7775 ) ;
#14777=VECTOR ( 'NONE', #16790, 1000.000000000000227 ) ;
#14779=ORIENTED_EDGE ( 'NONE', *, *, #1724, .T. ) ;
#14781=ORIENTED_EDGE ( 'NONE', *, *, #13876, .T. ) ;
#14782=PLANE ( 'NONE',  #13490 ) ;
#14788=DIRECTION ( 'NONE',  ( -0.4999999999999889533, -0.8660254037844450359, 0.000000000000000000 ) ) ;
#14789=DIRECTION ( 'NONE',  ( 0.5000000000000101030, -0.8660254037844328234, 0.000000000000000000 ) ) ;
#14790=ORIENTED_EDGE ( 'NONE', *, *, #17857, .T. ) ;
#14792=VECTOR ( 'NONE', #10296, 1000.000000000000227 ) ;
#14793=LINE ( 'NONE', #16240, #14877 ) ;
#14794=FACE_OUTER_BOUND ( 'NONE', #5016, .T. ) ;
#14795=VERTEX_POINT ( 'NONE', #18736 ) ;
#14796=LINE ( 'NONE', #8655, #940 ) ;
#14797=CARTESIAN_POINT ( 'NONE',  ( -39.80940113485986842, 48.72193424476489554, 293.5832628385307999 ) ) ;
#14799=CARTESIAN_POINT ( 'NONE',  ( 0.000000000000000000, 0.000000000000000000, 283.5832628385307999 ) ) ;
#14800=VECTOR ( 'NONE', #6343, 1000.000000000000000 ) ;
#14801=VECTOR ( 'NONE', #4740, 1000.000000000000114 ) ;
#14802=CARTESIAN_POINT ( 'NONE',  ( -54.07248341783231638, 32.16802499836798290, 293.5832628385307999 ) ) ;
#14803=CARTESIAN_POINT ( 'NONE',  ( -39.37628763770455009, -49.07263256785938665, 293.5832628385307999 ) ) ;
#14804=CARTESIAN_POINT ( 'NONE',  ( 68.18670162478805707, 38.41834839689404646, 110.9660488491356887 ) ) ;
#14806=CARTESIAN_POINT ( 'NONE',  ( 47.29944656917757584, 41.48948842197132336, 293.5832628385307999 ) ) ;
#14807=VERTEX_POINT ( 'NONE', #12061 ) ;
#14810=FACE_OUTER_BOUND ( 'NONE', #558, .T. ) ;
#14815=VECTOR ( 'NONE', #13157, 1000.000000000000000 ) ;
#14816=FACE_OUTER_BOUND ( 'NONE', #11058, .T. ) ;
#14817=CARTESIAN_POINT ( 'NONE',  ( 60.08331549348424971, 8.939227532413909216, 283.5832628385307999 ) ) ;
#14818=VERTEX_POINT ( 'NONE', #2777 ) ;
#14819=LINE ( 'NONE', #11830, #17858 ) ;
#14820=LINE ( 'NONE', #17805, #7140 ) ;
#14821=VECTOR ( 'NONE', #3819, 999.9999999999998863 ) ;
#14822=CARTESIAN_POINT ( 'NONE',  ( 25.99419088092191643, -73.82206860051539365, 111.4180192758973362 ) ) ;
#14824=LINE ( 'NONE', #712, #19372 ) ;
#14825=AXIS2_PLACEMENT_3D ( 'NONE', #17704, #19712, #17996 ) ;
#14827=CARTESIAN_POINT ( 'NONE',  ( 58.69016442926523069, -0.8220851292429179891, 132.4711112102474146 ) ) ;
#14834=AXIS2_PLACEMENT_3D ( 'NONE', #12704, #13932, #18658 ) ;
#14841=ORIENTED_EDGE ( 'NONE', *, *, #2526, .F. ) ;
#14843=DIRECTION ( 'NONE',  ( 1.000000000000000000, 0.000000000000000000, 0.000000000000000000 ) ) ;
#14844=ADVANCED_FACE ( 'NONE', ( #18325 ), #6261, .F. ) ;
#14845=CARTESIAN_POINT ( 'NONE',  ( -25.99419088092141550, 73.82206860051556419, 132.4711112102474146 ) ) ;
#14848=CARTESIAN_POINT ( 'NONE',  ( 0.000000000000000000, 0.000000000000000000, 283.5832628385307999 ) ) ;
#14850=EDGE_CURVE ( 'NONE', #3096, #6110, #13810, .T. ) ;
#14851=DIRECTION ( 'NONE',  ( -0.9848077530122104628, 0.1736481776669172861, 0.000000000000000000 ) ) ;
#14853=VERTEX_POINT ( 'NONE', #1442 ) ;
#14855=CIRCLE ( 'NONE', #14550, 60.74260934110282051 ) ;
#14856=EDGE_LOOP ( 'NONE', ( #6248, #11488, #1835 ) ) ;
#14857=EDGE_CURVE ( 'NONE', #13590, #10563, #20056, .T. ) ;
#14859=ORIENTED_EDGE ( 'NONE', *, *, #14424, .F. ) ;
#14861=CARTESIAN_POINT ( 'NONE',  ( 0.000000000000000000, 0.000000000000000000, 283.5832628385307999 ) ) ;
#14862=PLANE ( 'NONE',  #14189 ) ;
#14863=PLANE ( 'NONE',  #14952 ) ;
#14865=DIRECTION ( 'NONE',  ( 0.9781142164131917394, -0.2080686897406911207, 0.000000000000000000 ) ) ;
#14867=ADVANCED_FACE ( 'NONE', ( #18636 ), #17409, .T. ) ;
#14868=CARTESIAN_POINT ( 'NONE',  ( -5.281164089014724006, -2.240720816136035243, 293.5832628385307999 ) ) ;
#14873=ADVANCED_FACE ( 'NONE', ( #15968 ), #6461, .F. ) ;
#14877=VECTOR ( 'NONE', #8454, 1000.000000000000227 ) ;
#14880=ORIENTED_EDGE ( 'NONE', *, *, #5665, .T. ) ;
#14882=CARTESIAN_POINT ( 'NONE',  ( -68.46530598706770832, 37.93579148621532937, 132.4711112102474146 ) ) ;
#14883=LINE ( 'NONE', #17870, #7976 ) ;
#14884=CARTESIAN_POINT ( 'NONE',  ( -0.7000608949449798057, -5.693982670708954252, 283.5832628385307999 ) ) ;
#14885=ORIENTED_EDGE ( 'NONE', *, *, #15915, .F. ) ;
#14886=CARTESIAN_POINT ( 'NONE',  ( 53.40245231972179596, 28.94983032429848535, 283.5832628385307999 ) ) ;
#14888=ORIENTED_EDGE ( 'NONE', *, *, #7386, .T. ) ;
#14889=PLANE ( 'NONE',  #18252 ) ;
#14890=LINE ( 'NONE', #14797, #16558 ) ;
#14893=EDGE_CURVE ( 'NONE', #1634, #1213, #3484, .T. ) ;
#14894=CARTESIAN_POINT ( 'NONE',  ( 44.79940644582654841, -41.02350267428983699, 283.5832628385307999 ) ) ;
#14896=ADVANCED_FACE ( 'NONE', ( #14529 ), #12683, .T. ) ;
#14900=VERTEX_POINT ( 'NONE', #14433 ) ;
#14903=ORIENTED_EDGE ( 'NONE', *, *, #9526, .T. ) ;
#14907=ORIENTED_EDGE ( 'NONE', *, *, #15249, .F. ) ;
#14909=VECTOR ( 'NONE', #6427, 1000.000000000000227 ) ;
#14914=AXIS2_PLACEMENT_3D ( 'NONE', #2263, #18101, #3976 ) ;
#14916=DIRECTION ( 'NONE',  ( 0.5300553768524375320, 0.8479630283625697595, 0.000000000000000000 ) ) ;
#14917=EDGE_CURVE ( 'NONE', #19299, #6975, #8952, .T. ) ;
#14920=VERTEX_POINT ( 'NONE', #15763 ) ;
#14923=DIRECTION ( 'NONE',  ( 0.9848077530122085754, -0.1736481776669273336, 0.000000000000000000 ) ) ;
#14924=EDGE_CURVE ( 'NONE', #1866, #12611, #6692, .T. ) ;
#14927=CARTESIAN_POINT ( 'NONE',  ( 22.81000261549367991, -58.63718168490493099, 248.9926560891072143 ) ) ;
#14929=ORIENTED_EDGE ( 'NONE', *, *, #8885, .T. ) ;
#14932=CARTESIAN_POINT ( 'NONE',  ( -31.77296517111735596, -51.77251465595229263, 293.5832628385307999 ) ) ;
#14937=DIRECTION ( 'NONE',  ( -0.7881095627315599650, -0.6155349844899714595, 0.000000000000000000 ) ) ;
#14938=DIRECTION ( 'NONE',  ( 0.9848077530122073542, 0.1736481776669340227, -0.000000000000000000 ) ) ;
#14939=FACE_OUTER_BOUND ( 'NONE', #1703, .T. ) ;
#14941=DIRECTION ( 'NONE',  ( -0.3088643371590125697, 0.9511061040868803440, 0.000000000000000000 ) ) ;
#14943=DIRECTION ( 'NONE',  ( -0.7430374143461878633, 0.6692498792541777819, 0.000000000000000000 ) ) ;
#14944=LINE ( 'NONE', #13401, #16428 ) ;
#14945=LINE ( 'NONE', #19752, #15782 ) ;
#14946=EDGE_CURVE ( 'NONE', #4516, #195, #1744, .T. ) ;
#14947=VERTEX_POINT ( 'NONE', #9620 ) ;
#14948=DIRECTION ( 'NONE',  ( -0.000000000000000000, -0.000000000000000000, 1.000000000000000000 ) ) ;
#14951=ORIENTED_EDGE ( 'NONE', *, *, #1508, .T. ) ;
#14952=AXIS2_PLACEMENT_3D ( 'NONE', #13028, #14572, #16213 ) ;
#14953=VERTEX_POINT ( 'NONE', #16174 ) ;
#14961=LINE ( 'NONE', #16416, #7707 ) ;
#14962=DIRECTION ( 'NONE',  ( -0.03505990758545895342, -0.9993852124581886764, 0.000000000000000000 ) ) ;
#14968=DIRECTION ( 'NONE',  ( 0.6155349844899687950, -0.7881095627315619634, 0.000000000000000000 ) ) ;
#14970=CARTESIAN_POINT ( 'NONE',  ( -47.56244194535165803, -37.78198917157333625, 293.5832628385307999 ) ) ;
#14977=EDGE_LOOP ( 'NONE', ( #4602, #15034, #9825, #5407 ) ) ;
#14981=EDGE_CURVE ( 'NONE', #16297, #1477, #19244, .T. ) ;
#14982=AXIS2_PLACEMENT_3D ( 'NONE', #9595, #286, #15538 ) ;
#14984=EDGE_CURVE ( 'NONE', #3256, #8052, #2160, .T. ) ;
#14988=ORIENTED_EDGE ( 'NONE', *, *, #19884, .T. ) ;
#14991=ORIENTED_EDGE ( 'NONE', *, *, #2423, .T. ) ;
#14993=DIRECTION ( 'NONE',  ( -0.000000000000000000, -0.000000000000000000, 1.000000000000000000 ) ) ;
#14996=EDGE_CURVE ( 'NONE', #18905, #15888, #12577, .T. ) ;
#14997=EDGE_CURVE ( 'NONE', #6696, #3720, #12225, .T. ) ;
#14998=DIRECTION ( 'NONE',  ( 0.6427876096865481337, -0.7660444431189707970, 0.000000000000000000 ) ) ;
#14999=PLANE ( 'NONE',  #8697 ) ;
#15006=DIRECTION ( 'NONE',  ( -0.9848077530122085754, 0.1736481776669273336, 0.000000000000000000 ) ) ;
#15008=VERTEX_POINT ( 'NONE', #13079 ) ;
#15012=LINE ( 'NONE', #892, #16934 ) ;
#15013=EDGE_CURVE ( 'NONE', #12045, #11852, #13272, .T. ) ;
#15015=CARTESIAN_POINT ( 'NONE',  ( 8.938941455415006843, -60.08127757648380651, 293.5832628385307999 ) ) ;
#15016=PLANE ( 'NONE',  #14014 ) ;
#15020=CARTESIAN_POINT ( 'NONE',  ( -59.42266395395758138, 50.93469132750324491, 132.4711112102474146 ) ) ;
#15024=EDGE_CURVE ( 'NONE', #13684, #10955, #11555, .T. ) ;
#15025=LINE ( 'NONE', #4485, #9707 ) ;
#15027=CARTESIAN_POINT ( 'NONE',  ( 0.000000000000000000, 0.000000000000000000, 132.4711112102474146 ) ) ;
#15034=ORIENTED_EDGE ( 'NONE', *, *, #15385, .T. ) ;
#15036=EDGE_CURVE ( 'NONE', #19147, #4654, #806, .T. ) ;
#15037=ADVANCED_FACE ( 'NONE', ( #4176 ), #10408, .F. ) ;
#15039=CARTESIAN_POINT ( 'NONE',  ( -22.30005961346265408, -56.50329132715937419, 293.5832628385307999 ) ) ;
#15040=PLANE ( 'NONE',  #17226 ) ;
#15043=LINE ( 'NONE', #10524, #8319 ) ;
#15044=EDGE_CURVE ( 'NONE', #16743, #14586, #10308, .T. ) ;
#15049=DIRECTION ( 'NONE',  ( -0.8660254037844415942, 0.4999999999999950040, 0.000000000000000000 ) ) ;
#15052=ORIENTED_EDGE ( 'NONE', *, *, #13698, .T. ) ;
#15053=CARTESIAN_POINT ( 'NONE',  ( 7.948937137877743808, -60.22232964560488000, 293.5832628385307999 ) ) ;
#15055=ORIENTED_EDGE ( 'NONE', *, *, #5060, .T. ) ;
#15056=AXIS2_PLACEMENT_3D ( 'NONE', #3662, #5206, #13150 ) ;
#15059=LINE ( 'NONE', #7195, #2491 ) ;
#15060=ORIENTED_EDGE ( 'NONE', *, *, #10367, .F. ) ;
#15063=CARTESIAN_POINT ( 'NONE',  ( -73.25972925305609351, 27.53920554013712874, 111.4180192758973931 ) ) ;
#15065=CARTESIAN_POINT ( 'NONE',  ( 0.000000000000000000, 0.000000000000000000, 248.9926560891072143 ) ) ;
#15066=VERTEX_POINT ( 'NONE', #6953 ) ;
#15073=ORIENTED_EDGE ( 'NONE', *, *, #4220, .F. ) ;
#15077=ORIENTED_EDGE ( 'NONE', *, *, #16524, .T. ) ;
#15078=ORIENTED_EDGE ( 'NONE', *, *, #17799, .F. ) ;
#15080=CARTESIAN_POINT ( 'NONE',  ( -47.56244194535165803, -37.78198917157335046, 283.5832628385307999 ) ) ;
#15082=ORIENTED_EDGE ( 'NONE', *, *, #5611, .F. ) ;
#15083=AXIS2_PLACEMENT_3D ( 'NONE', #7619, #9050, #15297 ) ;
#15084=LINE ( 'NONE', #8025, #6088 ) ;
#15087=FACE_OUTER_BOUND ( 'NONE', #13779, .T. ) ;
#15089=CARTESIAN_POINT ( 'NONE',  ( -21.36933070621726571, 54.67896814532662830, 132.4711112102474146 ) ) ;
#15092=EDGE_CURVE ( 'NONE', #7122, #4330, #10214, .T. ) ;
#15094=FACE_OUTER_BOUND ( 'NONE', #2891, .T. ) ;
#15095=VERTEX_POINT ( 'NONE', #8487 ) ;
#15096=ADVANCED_FACE ( 'NONE', ( #14723 ), #13174, .F. ) ;
#15099=VECTOR ( 'NONE', #7981, 1000.000000000000227 ) ;
#15101=ORIENTED_EDGE ( 'NONE', *, *, #17750, .F. ) ;
#15102=CARTESIAN_POINT ( 'NONE',  ( 0.000000000000000000, 0.000000000000000000, 293.5832628385307999 ) ) ;
#15104=ORIENTED_EDGE ( 'NONE', *, *, #4911, .F. ) ;
#15107=DIRECTION ( 'NONE',  ( 1.000000000000000000, 0.000000000000000000, 0.000000000000000000 ) ) ;
#15109=FACE_OUTER_BOUND ( 'NONE', #17682, .T. ) ;
#15116=VECTOR ( 'NONE', #2797, 1000.000000000000114 ) ;
#15117=DIRECTION ( 'NONE',  ( 0.03505990758545895342, 0.9993852124581886764, 0.000000000000000000 ) ) ;
#15118=VERTEX_POINT ( 'NONE', #10125 ) ;
#15119=ADVANCED_FACE ( 'NONE', ( #8682 ), #18195, .F. ) ;
#15120=LINE ( 'NONE', #1103, #13295 ) ;
#15125=VERTEX_POINT ( 'NONE', #6131 ) ;
#15131=LINE ( 'NONE', #12364, #7139 ) ;
#15134=CARTESIAN_POINT ( 'NONE',  ( -55.16472960512350454, 30.25670013172272377, 132.4711112102474146 ) ) ;
#15136=LINE ( 'NONE', #12159, #16459 ) ;
#15139=FACE_OUTER_BOUND ( 'NONE', #14542, .T. ) ;
#15145=ADVANCED_FACE ( 'NONE', ( #1202 ), #9295, .F. ) ;
#15146=LINE ( 'NONE', #2781, #15909 ) ;
#15148=DIRECTION ( 'NONE',  ( 1.000000000000000000, 0.000000000000000000, 0.000000000000000000 ) ) ;
#15150=ORIENTED_EDGE ( 'NONE', *, *, #17778, .F. ) ;
#15152=LINE ( 'NONE', #4208, #2710 ) ;
#15154=VECTOR ( 'NONE', #6687, 1000.000000000000227 ) ;
#15155=EDGE_CURVE ( 'NONE', #18587, #16844, #16496, .T. ) ;
#15157=AXIS2_PLACEMENT_3D ( 'NONE', #252, #12420, #17455 ) ;
#15161=ORIENTED_EDGE ( 'NONE', *, *, #763, .T. ) ;
#15163=DIRECTION ( 'NONE',  ( -0.6692498792541753394, -0.7430374143461900838, 0.000000000000000000 ) ) ;
#15164=CARTESIAN_POINT ( 'NONE',  ( 79.75827554147308263, 9.767571684737763671E-15, 269.6944534026102360 ) ) ;
#15167=CARTESIAN_POINT ( 'NONE',  ( 32.64570716507540737, -53.78543575132139409, 248.9926560891072143 ) ) ;
#15168=VERTEX_POINT ( 'NONE', #18301 ) ;
#15172=DIRECTION ( 'NONE',  ( 0.000000000000000000, 0.000000000000000000, -1.000000000000000000 ) ) ;
#15177=EDGE_CURVE ( 'NONE', #15284, #7659, #20033, .T. ) ;
#15179=ORIENTED_EDGE ( 'NONE', *, *, #2364, .F. ) ;
#15181=VERTEX_POINT ( 'NONE', #1521 ) ;
#15185=CARTESIAN_POINT ( 'NONE',  ( -28.06584155524099700, 53.86996498385662591, 293.5832628385307999 ) ) ;
#15187=AXIS2_PLACEMENT_3D ( 'NONE', #3678, #13264, #11549 ) ;
#15188=CARTESIAN_POINT ( 'NONE',  ( -32.16802499836779106, -54.07248341783242296, 248.9926560891072143 ) ) ;
#15189=DIRECTION ( 'NONE',  ( 0.000000000000000000, 0.000000000000000000, 1.000000000000000000 ) ) ;
#15191=CYLINDRICAL_SURFACE ( 'NONE', #1595, 60.74260934110282051 ) ;
#15192=CARTESIAN_POINT ( 'NONE',  ( 0.000000000000000000, 0.000000000000000000, 283.5832628385307999 ) ) ;
#15195=CARTESIAN_POINT ( 'NONE',  ( -58.69016442926522359, 0.8220851292433277724, 248.9926560891072143 ) ) ;
#15196=AXIS2_PLACEMENT_3D ( 'NONE', #5158, #12604, #18867 ) ;
#15197=ORIENTED_EDGE ( 'NONE', *, *, #7504, .F. ) ;
#15198=EDGE_CURVE ( 'NONE', #19395, #10591, #1421, .T. ) ;
#15202=CARTESIAN_POINT ( 'NONE',  ( 38.41834839689379777, -68.18670162478818497, 248.9926560891072143 ) ) ;
#15203=ORIENTED_EDGE ( 'NONE', *, *, #9530, .T. ) ;
#15205=CARTESIAN_POINT ( 'NONE',  ( 28.06281046684275182, -73.06915264522010034, 248.9926560891072143 ) ) ;
#15206=EDGE_CURVE ( 'NONE', #18899, #16800, #20090, .T. ) ;
#15209=ORIENTED_EDGE ( 'NONE', *, *, #4273, .F. ) ;
#15211=LINE ( 'NONE', #5513, #18807 ) ;
#15212=CIRCLE ( 'NONE', #542, 60.74260934110282051 ) ;
#15215=DIRECTION ( 'NONE',  ( -0.000000000000000000, -0.000000000000000000, 1.000000000000000000 ) ) ;
#15217=LINE ( 'NONE', #12248, #12567 ) ;
#15219=LINE ( 'NONE', #10411, #880 ) ;
#15222=VERTEX_POINT ( 'NONE', #8976 ) ;
#15223=EDGE_CURVE ( 'NONE', #18597, #12045, #15217, .T. ) ;
#15225=CARTESIAN_POINT ( 'NONE',  ( -60.72073886220397299, 1.629865514042312613, 283.5832628385307999 ) ) ;
#15228=ORIENTED_EDGE ( 'NONE', *, *, #17094, .F. ) ;
#15230=AXIS2_PLACEMENT_3D ( 'NONE', #9382, #15727, #12544 ) ;
#15232=FACE_OUTER_BOUND ( 'NONE', #1665, .T. ) ;
#15233=AXIS2_PLACEMENT_3D ( 'NONE', #16839, #4567, #2731 ) ;
#15234=EDGE_CURVE ( 'NONE', #19683, #9722, #13990, .T. ) ;
#15240=AXIS2_PLACEMENT_3D ( 'NONE', #15192, #16835, #17148 ) ;
#15242=CYLINDRICAL_SURFACE ( 'NONE', #10817, 60.74260934110282051 ) ;
#15244=CYLINDRICAL_SURFACE ( 'NONE', #16895, 79.75827554147308263 ) ;
#15246=DIRECTION ( 'NONE',  ( -0.000000000000000000, -0.000000000000000000, 1.000000000000000000 ) ) ;
#15248=VECTOR ( 'NONE', #18008, 1000.000000000000000 ) ;
#15249=EDGE_CURVE ( 'NONE', #20227, #12671, #17182, .T. ) ;
#15251=CARTESIAN_POINT ( 'NONE',  ( -19.30071112029641967, 55.43188410062188609, 111.4180192758973931 ) ) ;
#15254=ORIENTED_EDGE ( 'NONE', *, *, #10595, .T. ) ;
#15260=DIRECTION ( 'NONE',  ( -0.9511061040868794558, -0.3088643371590157338, 0.000000000000000000 ) ) ;
#15268=CARTESIAN_POINT ( 'NONE',  ( -51.24071425735602503, 32.61983739937743820, 293.5832628385307999 ) ) ;
#15269=ORIENTED_EDGE ( 'NONE', *, *, #2640, .F. ) ;
#15270=CARTESIAN_POINT ( 'NONE',  ( 0.000000000000000000, 0.000000000000000000, 283.5832628385307999 ) ) ;
#15277=EDGE_CURVE ( 'NONE', #16849, #9808, #2854, .T. ) ;
#15279=CIRCLE ( 'NONE', #4181, 62.91752772691707207 ) ;
#15280=CIRCLE ( 'NONE', #12322, 62.91752772691707207 ) ;
#15281=VERTEX_POINT ( 'NONE', #4484 ) ;
#15284=VERTEX_POINT ( 'NONE', #20131 ) ;
#15285=EDGE_CURVE ( 'NONE', #4813, #10391, #1931, .T. ) ;
#15287=LINE ( 'NONE', #9565, #15830 ) ;
#15288=DIRECTION ( 'NONE',  ( -0.000000000000000000, -0.000000000000000000, 1.000000000000000000 ) ) ;
#15289=ORIENTED_EDGE ( 'NONE', *, *, #13842, .F. ) ;
#15296=AXIS2_PLACEMENT_3D ( 'NONE', #2267, #19635, #5527 ) ;
#15297=DIRECTION ( 'NONE',  ( -0.9848077530122073542, -0.1736481776669340227, 0.000000000000000000 ) ) ;
#15299=PLANE ( 'NONE',  #18322 ) ;
#15300=LINE ( 'NONE', #1292, #4849 ) ;
#15301=CARTESIAN_POINT ( 'NONE',  ( -49.67518383744793908, 60.47951622432801599, 110.7293897666001214 ) ) ;
#15302=VERTEX_POINT ( 'NONE', #9796 ) ;
#15306=ORIENTED_EDGE ( 'NONE', *, *, #2102, .F. ) ;
#15308=VERTEX_POINT ( 'NONE', #17488 ) ;
#15311=ORIENTED_EDGE ( 'NONE', *, *, #685, .F. ) ;
#15312=ORIENTED_EDGE ( 'NONE', *, *, #7039, .F. ) ;
#15316=DIRECTION ( 'NONE',  ( -0.000000000000000000, -0.000000000000000000, 1.000000000000000000 ) ) ;
#15319=ORIENTED_EDGE ( 'NONE', *, *, #6884, .T. ) ;
#15322=VECTOR ( 'NONE', #2076, 1000.000000000000114 ) ;
#15323=CIRCLE ( 'NONE', #4211, 62.91752772691707207 ) ;
#15324=CARTESIAN_POINT ( 'NONE',  ( 61.70726652483817531, 12.28122767885865407, 293.5832628385307999 ) ) ;
#15328=ORIENTED_EDGE ( 'NONE', *, *, #3182, .T. ) ;
#15330=CARTESIAN_POINT ( 'NONE',  ( 40.28046525994349736, 45.46865632508086463, 283.5832628385307999 ) ) ;
#15331=EDGE_LOOP ( 'NONE', ( #16083, #5090, #19455, #3430 ) ) ;
#15334=ORIENTED_EDGE ( 'NONE', *, *, #18863, .F. ) ;
#15337=CARTESIAN_POINT ( 'NONE',  ( 0.000000000000000000, 0.000000000000000000, 283.5832628385307999 ) ) ;
#15338=FACE_OUTER_BOUND ( 'NONE', #4947, .T. ) ;
#15344=DIRECTION ( 'NONE',  ( 0.4693298356057564180, -0.8830229359480272766, 0.000000000000000000 ) ) ;
#15350=VECTOR ( 'NONE', #12811, 1000.000000000000227 ) ;
#15353=ADVANCED_FACE ( 'NONE', ( #3360 ), #12863, .F. ) ;
#15356=ADVANCED_FACE ( 'NONE', ( #1825 ), #11024, .F. ) ;
#15357=VERTEX_POINT ( 'NONE', #15945 ) ;
#15358=ADVANCED_FACE ( 'NONE', ( #3461 ), #18923, .F. ) ;
#15363=FACE_BOUND ( 'NONE', #16898, .T. ) ;
#15365=VECTOR ( 'NONE', #10213, 1000.000000000000227 ) ;
#15366=CARTESIAN_POINT ( 'NONE',  ( -51.51682027493045979, 28.15057869795642986, 110.9660488491356887 ) ) ;
#15371=LINE ( 'NONE', #5867, #6497 ) ;
#15375=CARTESIAN_POINT ( 'NONE',  ( 48.72193424476451895, 39.80940113486035159, 248.9926560891072143 ) ) ;
#15380=ORIENTED_EDGE ( 'NONE', *, *, #6919, .T. ) ;
#15382=CARTESIAN_POINT ( 'NONE',  ( -41.48948842197086151, 47.29944656917798795, 293.5832628385307999 ) ) ;
#15383=ADVANCED_FACE ( 'NONE', ( #6440 ), #14309, .F. ) ;
#15385=EDGE_CURVE ( 'NONE', #18152, #6652, #1804, .T. ) ;
#15386=ORIENTED_EDGE ( 'NONE', *, *, #20115, .T. ) ;
#15391=VECTOR ( 'NONE', #18343, 1000.000000000000227 ) ;
#15392=EDGE_CURVE ( 'NONE', #18157, #10298, #2443, .T. ) ;
#15393=DIRECTION ( 'NONE',  ( -0.000000000000000000, -0.000000000000000000, 1.000000000000000000 ) ) ;
#15398=CARTESIAN_POINT ( 'NONE',  ( 40.28046525994349736, 45.46865632508086463, 293.5832628385307999 ) ) ;
#15399=ORIENTED_EDGE ( 'NONE', *, *, #15480, .T. ) ;
#15401=DIRECTION ( 'NONE',  ( -0.3420201433256568890, -0.9396926207859126468, -0.000000000000000000 ) ) ;
#15402=DIRECTION ( 'NONE',  ( -0.000000000000000000, -0.000000000000000000, 1.000000000000000000 ) ) ;
#15404=DIRECTION ( 'NONE',  ( -0.6692498792541753394, -0.7430374143461900838, 0.000000000000000000 ) ) ;
#15406=CARTESIAN_POINT ( 'NONE',  ( -62.90240729679781850, -1.379293853801974779, 248.9926560891072143 ) ) ;
#15407=DIRECTION ( 'NONE',  ( -0.000000000000000000, -0.000000000000000000, 1.000000000000000000 ) ) ;
#15408=EDGE_CURVE ( 'NONE', #15066, #18605, #12241, .T. ) ;
#15410=ORIENTED_EDGE ( 'NONE', *, *, #2142, .T. ) ;
#15414=VERTEX_POINT ( 'NONE', #14506 ) ;
#15415=CARTESIAN_POINT ( 'NONE',  ( -0.8220851292435327196, -58.69016442926522359, 112.7772637782949943 ) ) ;
#15417=VECTOR ( 'NONE', #15916, 1000.000000000000000 ) ;
#15419=DIRECTION ( 'NONE',  ( -0.9396926207859046531, -0.3420201433256790380, 0.000000000000000000 ) ) ;
#15420=CARTESIAN_POINT ( 'NONE',  ( 28.06281046684275182, -73.06915264522012876, 132.4711112102474146 ) ) ;
#15421=DIRECTION ( 'NONE',  ( -0.000000000000000000, -0.000000000000000000, 1.000000000000000000 ) ) ;
#15424=DIRECTION ( 'NONE',  ( 0.03505990758545895342, 0.9993852124581886764, 0.000000000000000000 ) ) ;
#15425=CARTESIAN_POINT ( 'NONE',  ( 73.82206860051530839, 25.99419088092216867, 132.4711112102474146 ) ) ;
#15428=LINE ( 'NONE', #9185, #1608 ) ;
#15429=DIRECTION ( 'NONE',  ( 0.000000000000000000, 0.000000000000000000, -1.000000000000000000 ) ) ;
#15432=LINE ( 'NONE', #1422, #19522 ) ;
#15435=ORIENTED_EDGE ( 'NONE', *, *, #10609, .F. ) ;
#15441=ORIENTED_EDGE ( 'NONE', *, *, #15533, .F. ) ;
#15443=ORIENTED_EDGE ( 'NONE', *, *, #17624, .F. ) ;
#15444=CARTESIAN_POINT ( 'NONE',  ( 9.564549117045078930, 62.18629025319817316, 132.4711112102474146 ) ) ;
#15445=PLANE ( 'NONE',  #5659 ) ;
#15446=CIRCLE ( 'NONE', #15795, 62.91752772691707207 ) ;
#15447=ORIENTED_EDGE ( 'NONE', *, *, #14286, .F. ) ;
#15448=AXIS2_PLACEMENT_3D ( 'NONE', #5482, #19403, #11705 ) ;
#15451=AXIS2_PLACEMENT_3D ( 'NONE', #7237, #9171, #18181 ) ;
#15456=DIRECTION ( 'NONE',  ( 1.000000000000000000, 0.000000000000000000, 0.000000000000000000 ) ) ;
#15458=ORIENTED_EDGE ( 'NONE', *, *, #2391, .F. ) ;
#15460=DIRECTION ( 'NONE',  ( 0.3420201433256694901, -0.9396926207859082059, 0.000000000000000000 ) ) ;
#15463=EDGE_LOOP ( 'NONE', ( #7201, #9481, #5241, #17066 ) ) ;
#15464=EDGE_CURVE ( 'NONE', #17279, #1274, #289, .T. ) ;
#15468=VERTEX_POINT ( 'NONE', #17590 ) ;
#15470=FACE_BOUND ( 'NONE', #3168, .T. ) ;
#15472=DIRECTION ( 'NONE',  ( -0.6155349844899689060, 0.7881095627315620744, 0.000000000000000000 ) ) ;
#15473=LINE ( 'NONE', #6283, #15484 ) ;
#15474=LINE ( 'NONE', #18138, #5837 ) ;
#15479=DIRECTION ( 'NONE',  ( 0.8830229359480271656, 0.4693298356057563625, 0.000000000000000000 ) ) ;
#15480=EDGE_CURVE ( 'NONE', #19763, #12174, #5571, .T. ) ;
#15484=VECTOR ( 'NONE', #6180, 1000.000000000000114 ) ;
#15485=LINE ( 'NONE', #3010, #11147 ) ;
#15489=DIRECTION ( 'NONE',  ( -1.000000000000000000, 0.000000000000000000, 0.000000000000000000 ) ) ;
#15490=AXIS2_PLACEMENT_3D ( 'NONE', #18704, #19108, #1618 ) ;
#15491=EDGE_CURVE ( 'NONE', #15722, #14388, #10933, .T. ) ;
#15492=ORIENTED_EDGE ( 'NONE', *, *, #18527, .T. ) ;
#15493=ORIENTED_EDGE ( 'NONE', *, *, #15392, .F. ) ;
#15494=ORIENTED_EDGE ( 'NONE', *, *, #430, .T. ) ;
#15499=VECTOR ( 'NONE', #1996, 1000.000000000000000 ) ;
#15500=DIRECTION ( 'NONE',  ( -0.9902903945359624593, -0.1390141521205945918, 0.000000000000000000 ) ) ;
#15504=CYLINDRICAL_SURFACE ( 'NONE', #4909, 62.91752772691707207 ) ;
#15505=VERTEX_POINT ( 'NONE', #16621 ) ;
#15507=PLANE ( 'NONE',  #2843 ) ;
#15509=CARTESIAN_POINT ( 'NONE',  ( 0.000000000000000000, 0.000000000000000000, 132.4711112102474146 ) ) ;
#15510=LINE ( 'NONE', #1496, #5579 ) ;
#15511=DIRECTION ( 'NONE',  ( -0.6427876096865430267, 0.7660444431189749048, 0.000000000000000000 ) ) ;
#15512=VECTOR ( 'NONE', #8732, 1000.000000000000114 ) ;
#15515=VERTEX_POINT ( 'NONE', #13426 ) ;
#15518=EDGE_LOOP ( 'NONE', ( #13846, #17012, #15720, #1405 ) ) ;
#15520=CARTESIAN_POINT ( 'NONE',  ( 60.68773558783009747, -2.629322876227576433, 293.5832628385307999 ) ) ;
#15522=DIRECTION ( 'NONE',  ( -0.000000000000000000, -0.000000000000000000, 1.000000000000000000 ) ) ;
#15523=VECTOR ( 'NONE', #10207, 1000.000000000000000 ) ;
#15524=LINE ( 'NONE', #15729, #12696 ) ;
#15527=VERTEX_POINT ( 'NONE', #14970 ) ;
#15530=EDGE_CURVE ( 'NONE', #16066, #12093, #8931, .T. ) ;
#15532=CARTESIAN_POINT ( 'NONE',  ( -60.72073886220397299, 1.629865514042312613, 283.5832628385307999 ) ) ;
#15533=EDGE_CURVE ( 'NONE', #19640, #10955, #587, .T. ) ;
#15538=DIRECTION ( 'NONE',  ( 0.5000000000000069944, -0.8660254037844345998, 0.000000000000000000 ) ) ;
#15539=DIRECTION ( 'NONE',  ( 1.000000000000000000, 0.000000000000000000, 0.000000000000000000 ) ) ;
#15547=VERTEX_POINT ( 'NONE', #9954 ) ;
#15548=DIRECTION ( 'NONE',  ( -0.3747554100459959403, -0.9271237148521535021, 0.000000000000000000 ) ) ;
#15551=DIRECTION ( 'NONE',  ( 0.7660444431189726844, 0.6427876096865456912, 0.000000000000000000 ) ) ;
#15553=ADVANCED_FACE ( 'NONE', ( #11484 ), #3713, .T. ) ;
#15556=AXIS2_PLACEMENT_3D ( 'NONE', #17090, #3, #10939 ) ;
#15557=EDGE_CURVE ( 'NONE', #15547, #12093, #646, .T. ) ;
#15562=DIRECTION ( 'NONE',  ( -0.9396926207859092051, 0.3420201433256662704, 0.000000000000000000 ) ) ;
#15563=CARTESIAN_POINT ( 'NONE',  ( -25.99419088092141550, 73.82206860051556419, 111.4180192758973931 ) ) ;
#15572=ORIENTED_EDGE ( 'NONE', *, *, #2102, .T. ) ;
#15574=EDGE_LOOP ( 'NONE', ( #4113, #17027, #16431, #6940 ) ) ;
#15575=DIRECTION ( 'NONE',  ( -0.000000000000000000, -0.000000000000000000, 1.000000000000000000 ) ) ;
#15577=ORIENTED_EDGE ( 'NONE', *, *, #19767, .T. ) ;
#15581=VECTOR ( 'NONE', #2563, 1000.000000000000000 ) ;
#15586=CYLINDRICAL_SURFACE ( 'NONE', #1309, 60.74260934110282051 ) ;
#15587=DIRECTION ( 'NONE',  ( 0.8830229359480271656, 0.4693298356057563625, 0.000000000000000000 ) ) ;
#15589=FACE_OUTER_BOUND ( 'NONE', #13428, .T. ) ;
#15590=DIRECTION ( 'NONE',  ( -0.000000000000000000, -0.000000000000000000, 1.000000000000000000 ) ) ;
#15593=ORIENTED_EDGE ( 'NONE', *, *, #19400, .T. ) ;
#15596=ORIENTED_EDGE ( 'NONE', *, *, #9444, .T. ) ;
#15597=ORIENTED_EDGE ( 'NONE', *, *, #2523, .F. ) ;
#15598=AXIS2_PLACEMENT_3D ( 'NONE', #9137, #1156, #17233 ) ;
#15600=LINE ( 'NONE', #7916, #11887 ) ;
#15601=CARTESIAN_POINT ( 'NONE',  ( -44.43084819159250287, 38.35506425062501989, 132.4711112102474146 ) ) ;
#15602=ORIENTED_EDGE ( 'NONE', *, *, #12282, .F. ) ;
#15603=DIRECTION ( 'NONE',  ( -0.9902903945359624593, -0.1390141521205945918, 0.000000000000000000 ) ) ;
#15604=DIRECTION ( 'NONE',  ( 1.000000000000000000, 0.000000000000000000, 0.000000000000000000 ) ) ;
#15606=LINE ( 'NONE', #6100, #8450 ) ;
#15608=LINE ( 'NONE', #1493, #14280 ) ;
#15614=VECTOR ( 'NONE', #4306, 1000.000000000000114 ) ;
#15615=CARTESIAN_POINT ( 'NONE',  ( -45.48770046196285932, -37.09555676056982065, 110.7293897666001214 ) ) ;
#15617=ORIENTED_EDGE ( 'NONE', *, *, #6787, .F. ) ;
#15618=ORIENTED_EDGE ( 'NONE', *, *, #12081, .T. ) ;
#15619=ADVANCED_FACE ( 'NONE', ( #551 ), #16001, .T. ) ;
#15620=ORIENTED_EDGE ( 'NONE', *, *, #15013, .T. ) ;
#15622=ORIENTED_EDGE ( 'NONE', *, *, #376, .T. ) ;
#15625=ORIENTED_EDGE ( 'NONE', *, *, #4532, .T. ) ;
#15633=EDGE_LOOP ( 'NONE', ( #11159, #7408, #12329, #3675 ) ) ;
#15634=CYLINDRICAL_SURFACE ( 'NONE', #3795, 62.91752772691707207 ) ;
#15635=CARTESIAN_POINT ( 'NONE',  ( 53.40245231972179596, 28.94983032429848535, 293.5832628385307999 ) ) ;
#15637=ORIENTED_EDGE ( 'NONE', *, *, #9530, .F. ) ;
#15640=CARTESIAN_POINT ( 'NONE',  ( 0.000000000000000000, 0.000000000000000000, 283.5832628385307999 ) ) ;
#15641=DIRECTION ( 'NONE',  ( 1.000000000000000000, 0.000000000000000000, 0.000000000000000000 ) ) ;
#15642=AXIS2_PLACEMENT_3D ( 'NONE', #18394, #7435, #4167 ) ;
#15643=LINE ( 'NONE', #14097, #2527 ) ;
#15647=AXIS2_PLACEMENT_3D ( 'NONE', #14527, #14720, #13269 ) ;
#15652=EDGE_CURVE ( 'NONE', #9808, #20114, #8336, .T. ) ;
#15654=ORIENTED_EDGE ( 'NONE', *, *, #10120, .T. ) ;
#15660=ORIENTED_EDGE ( 'NONE', *, *, #2895, .T. ) ;
#15662=LINE ( 'NONE', #10831, #13207 ) ;
#15663=VECTOR ( 'NONE', #2226, 1000.000000000000000 ) ;
#15668=LINE ( 'NONE', #6263, #2369 ) ;
#15669=FACE_OUTER_BOUND ( 'NONE', #9214, .T. ) ;
#15672=EDGE_LOOP ( 'NONE', ( #10198, #15060, #2916, #13310 ) ) ;
#15673=LINE ( 'NONE', #11054, #18910 ) ;
#15678=VECTOR ( 'NONE', #8797, 1000.000000000000000 ) ;
#15679=AXIS2_PLACEMENT_3D ( 'NONE', #3130, #7716, #4449 ) ;
#15683=VERTEX_POINT ( 'NONE', #4002 ) ;
#15684=EDGE_CURVE ( 'NONE', #8543, #2811, #14139, .T. ) ;
#15689=DIRECTION ( 'NONE',  ( 0.000000000000000000, 0.000000000000000000, -1.000000000000000000 ) ) ;
#15694=LINE ( 'NONE', #6589, #15350 ) ;
#15696=DIRECTION ( 'NONE',  ( -0.000000000000000000, -0.000000000000000000, 1.000000000000000000 ) ) ;
#15697=CARTESIAN_POINT ( 'NONE',  ( 27.53920554013639688, 73.25972925305639194, 111.4180192758974499 ) ) ;
#15699=ORIENTED_EDGE ( 'NONE', *, *, #1658, .T. ) ;
#15701=DIRECTION ( 'NONE',  ( -0.000000000000000000, -0.000000000000000000, 1.000000000000000000 ) ) ;
#15704=AXIS2_PLACEMENT_3D ( 'NONE', #18839, #9521, #14118 ) ;
#15708=CARTESIAN_POINT ( 'NONE',  ( 68.18670162478805707, 38.41834839689404646, 132.4711112102474146 ) ) ;
#15709=CARTESIAN_POINT ( 'NONE',  ( 40.32479851956816930, -67.08601213326551260, 248.9926560891072143 ) ) ;
#15710=LINE ( 'NONE', #9047, #18281 ) ;
#15711=LINE ( 'NONE', #8128, #296 ) ;
#15712=PLANE ( 'NONE',  #11503 ) ;
#15713=DIRECTION ( 'NONE',  ( 0.000000000000000000, 0.000000000000000000, -1.000000000000000000 ) ) ;
#15715=CARTESIAN_POINT ( 'NONE',  ( 0.000000000000000000, 0.000000000000000000, 132.4711112102474146 ) ) ;
#15718=LINE ( 'NONE', #5848, #6093 ) ;
#15719=ORIENTED_EDGE ( 'NONE', *, *, #5735, .T. ) ;
#15720=ORIENTED_EDGE ( 'NONE', *, *, #5068, .T. ) ;
#15722=VERTEX_POINT ( 'NONE', #5646 ) ;
#15723=EDGE_CURVE ( 'NONE', #9758, #15949, #17938, .T. ) ;
#15724=FACE_OUTER_BOUND ( 'NONE', #13345, .T. ) ;
#15725=AXIS2_PLACEMENT_3D ( 'NONE', #16944, #6104, #7828 ) ;
#15726=ORIENTED_EDGE ( 'NONE', *, *, #7717, .F. ) ;
#15727=DIRECTION ( 'NONE',  ( -0.9396926207859127578, 0.3420201433256568335, 0.000000000000000000 ) ) ;
#15728=CARTESIAN_POINT ( 'NONE',  ( 59.42266395395792955, -50.93469132750283279, 110.7293897666001214 ) ) ;
#15729=CARTESIAN_POINT ( 'NONE',  ( 2.605298826210328045, 5.111158570922230915, 293.5832628385307999 ) ) ;
#15735=EDGE_CURVE ( 'NONE', #3219, #19783, #16427, .T. ) ;
#15737=LINE ( 'NONE', #13888, #9437 ) ;
#15738=ADVANCED_FACE ( 'NONE', ( #8613 ), #18223, .T. ) ;
#15739=EDGE_CURVE ( 'NONE', #3073, #15683, #1132, .T. ) ;
#15740=DIRECTION ( 'NONE',  ( -0.5000000000000039968, 0.8660254037844363761, 0.000000000000000000 ) ) ;
#15742=DIRECTION ( 'NONE',  ( -0.9781142164131917394, 0.2080686897406911207, 0.000000000000000000 ) ) ;
#15746=LINE ( 'NONE', #6549, #2395 ) ;
#15748=ORIENTED_EDGE ( 'NONE', *, *, #16795, .T. ) ;
#15751=ORIENTED_EDGE ( 'NONE', *, *, #157, .F. ) ;
#15752=DIRECTION ( 'NONE',  ( 0.000000000000000000, 1.000000000000000000, -0.000000000000000000 ) ) ;
#15754=VERTEX_POINT ( 'NONE', #11964 ) ;
#15755=( NAMED_UNIT ( * ) PLANE_ANGLE_UNIT ( ) SI_UNIT ( $, .RADIAN. ) );
#15757=EDGE_CURVE ( 'NONE', #10035, #18230, #14945, .T. ) ;
#15759=AXIS2_PLACEMENT_3D ( 'NONE', #3133, #2826, #4669 ) ;
#15760=EDGE_CURVE ( 'NONE', #5114, #4761, #7277, .T. ) ;
#15763=CARTESIAN_POINT ( 'NONE',  ( 60.22029172860436574, 7.948651060879242003, 293.5832628385307999 ) ) ;
#15764=ORIENTED_EDGE ( 'NONE', *, *, #5928, .F. ) ;
#15765=DIRECTION ( 'NONE',  ( 1.000000000000000000, 0.000000000000000000, 0.000000000000000000 ) ) ;
#15766=CARTESIAN_POINT ( 'NONE',  ( 0.000000000000000000, 0.000000000000000000, 132.4711112102474146 ) ) ;
#15767=LINE ( 'NONE', #15973, #16354 ) ;
#15770=DIRECTION ( 'NONE',  ( 1.000000000000000000, 0.000000000000000000, 0.000000000000000000 ) ) ;
#15772=ORIENTED_EDGE ( 'NONE', *, *, #12233, .T. ) ;
#15777=VECTOR ( 'NONE', #342, 1000.000000000000000 ) ;
#15778=EDGE_LOOP ( 'NONE', ( #7126, #3370, #8392 ) ) ;
#15780=DIRECTION ( 'NONE',  ( -0.9271237148521547233, 0.3747554100459928872, 0.000000000000000000 ) ) ;
#15782=VECTOR ( 'NONE', #832, 1000.000000000000000 ) ;
#15784=DIRECTION ( 'NONE',  ( 0.6427876096865405842, -0.7660444431189771253, 0.000000000000000000 ) ) ;
#15787=EDGE_CURVE ( 'NONE', #19280, #13684, #2784, .T. ) ;
#15789=EDGE_CURVE ( 'NONE', #9422, #17872, #10334, .T. ) ;
#15794=CARTESIAN_POINT ( 'NONE',  ( 0.000000000000000000, 0.000000000000000000, 132.4711112102474146 ) ) ;
#15795=AXIS2_PLACEMENT_3D ( 'NONE', #13715, #5957, #4413 ) ;
#15796=AXIS2_PLACEMENT_3D ( 'NONE', #4635, #10859, #6380 ) ;
#15797=DIRECTION ( 'NONE',  ( -0.000000000000000000, -0.000000000000000000, 1.000000000000000000 ) ) ;
#15798=CARTESIAN_POINT ( 'NONE',  ( -3.911853314815649796, 4.196299268919085890, 283.5832628385307999 ) ) ;
#15800=VERTEX_POINT ( 'NONE', #19466 ) ;
#15801=CARTESIAN_POINT ( 'NONE',  ( 0.000000000000000000, 0.000000000000000000, 283.5832628385307999 ) ) ;
#15803=VECTOR ( 'NONE', #2943, 1000.000000000000000 ) ;
#15804=ORIENTED_EDGE ( 'NONE', *, *, #10505, .T. ) ;
#15805=ORIENTED_EDGE ( 'NONE', *, *, #5735, .F. ) ;
#15806=AXIS2_PLACEMENT_3D ( 'NONE', #1831, #15950, #6446 ) ;
#15807=EDGE_LOOP ( 'NONE', ( #20091, #19492, #17762, #12263 ) ) ;
#15809=CARTESIAN_POINT ( 'NONE',  ( 58.03804081968166173, -8.833100819207778898, 112.0427633081292385 ) ) ;
#15811=DIRECTION ( 'NONE',  ( 0.8660254037844432595, -0.4999999999999919509, 0.000000000000000000 ) ) ;
#15812=ORIENTED_EDGE ( 'NONE', *, *, #11469, .F. ) ;
#15813=DIRECTION ( 'NONE',  ( 0.000000000000000000, 0.000000000000000000, 1.000000000000000000 ) ) ;
#15815=LINE ( 'NONE', #12629, #19260 ) ;
#15819=EDGE_CURVE ( 'NONE', #20066, #19327, #10151, .T. ) ;
#15824=ORIENTED_EDGE ( 'NONE', *, *, #12864, .T. ) ;
#15826=ORIENTED_EDGE ( 'NONE', *, *, #4535, .F. ) ;
#15827=VECTOR ( 'NONE', #17831, 1000.000000000000000 ) ;
#15830=VECTOR ( 'NONE', #17556, 1000.000000000000000 ) ;
#15831=ORIENTED_EDGE ( 'NONE', *, *, #8359, .F. ) ;
#15834=CARTESIAN_POINT ( 'NONE',  ( 28.06680738835026290, -53.87178215532764369, 293.5832628385307999 ) ) ;
#15835=PLANE ( 'NONE',  #1886 ) ;
#15836=VERTEX_POINT ( 'NONE', #17207 ) ;
#15840=LINE ( 'NONE', #384, #8390 ) ;
#15841=PLANE ( 'NONE',  #3244 ) ;
#15842=AXIS2_PLACEMENT_3D ( 'NONE', #5845, #11764, #7272 ) ;
#15843=CARTESIAN_POINT ( 'NONE',  ( 55.16472960512370349, -30.25670013172234007, 293.5832628385307999 ) ) ;
#15845=DIRECTION ( 'NONE',  ( -0.9511061040868794558, -0.3088643371590157338, 0.000000000000000000 ) ) ;
#15847=DIRECTION ( 'NONE',  ( 1.000000000000000000, 0.000000000000000000, 0.000000000000000000 ) ) ;
#15849=ORIENTED_EDGE ( 'NONE', *, *, #17560, .F. ) ;
#15850=CARTESIAN_POINT ( 'NONE',  ( 58.83691981461633702, -22.28973221005102090, 248.9926560891072143 ) ) ;
#15854=DIRECTION ( 'NONE',  ( 0.000000000000000000, 0.000000000000000000, -1.000000000000000000 ) ) ;
#15857=ORIENTED_EDGE ( 'NONE', *, *, #3793, .T. ) ;
#15859=DIRECTION ( 'NONE',  ( 0.000000000000000000, 0.000000000000000000, 1.000000000000000000 ) ) ;
#15861=SURFACE_STYLE_FILL_AREA ( #9813 ) ;
#15862=FACE_OUTER_BOUND ( 'NONE', #17947, .T. ) ;
#15865=AXIS2_PLACEMENT_3D ( 'NONE', #17802, #16269, #2249 ) ;
#15867=CARTESIAN_POINT ( 'NONE',  ( -59.58067424803613221, 20.21777810286735289, 248.9926560891072143 ) ) ;
#15870=CARTESIAN_POINT ( 'NONE',  ( -30.74413178637153976, 54.89456854707572830, 248.9926560891072143 ) ) ;
#15879=VECTOR ( 'NONE', #2225, 1000.000000000000227 ) ;
#15882=EDGE_CURVE ( 'NONE', #5311, #15357, #3489, .T. ) ;
#15884=ORIENTED_EDGE ( 'NONE', *, *, #18673, .F. ) ;
#15885=EDGE_CURVE ( 'NONE', #17837, #3073, #522, .T. ) ;
#15888=VERTEX_POINT ( 'NONE', #8190 ) ;
#15893=DIRECTION ( 'NONE',  ( 0.8660254037844415942, -0.4999999999999950040, 0.000000000000000000 ) ) ;
#15896=FACE_OUTER_BOUND ( 'NONE', #6198, .T. ) ;
#15897=DIRECTION ( 'NONE',  ( 0.000000000000000000, 0.000000000000000000, 1.000000000000000000 ) ) ;
#15899=VERTEX_POINT ( 'NONE', #13085 ) ;
#15901=ORIENTED_EDGE ( 'NONE', *, *, #6814, .T. ) ;
#15902=ADVANCED_FACE ( 'NONE', ( #2065 ), #19250, .F. ) ;
#15907=VECTOR ( 'NONE', #6325, 1000.000000000000000 ) ;
#15908=ORIENTED_EDGE ( 'NONE', *, *, #750, .T. ) ;
#15909=VECTOR ( 'NONE', #18640, 1000.000000000000000 ) ;
#15910=LINE ( 'NONE', #18682, #791 ) ;
#15911=DIRECTION ( 'NONE',  ( 0.000000000000000000, 0.000000000000000000, -1.000000000000000000 ) ) ;
#15913=CARTESIAN_POINT ( 'NONE',  ( -14.94814811854910275, 76.83212392882506947, 132.4711112102474146 ) ) ;
#15914=LINE ( 'NONE', #17459, #5521 ) ;
#15915=EDGE_CURVE ( 'NONE', #13875, #4038, #209, .T. ) ;
#15916=DIRECTION ( 'NONE',  ( -0.000000000000000000, -0.000000000000000000, 1.000000000000000000 ) ) ;
#15917=LINE ( 'NONE', #6810, #10117 ) ;
#15920=EDGE_LOOP ( 'NONE', ( #14033, #12113, #694, #19374 ) ) ;
#15923=VERTEX_POINT ( 'NONE', #6466 ) ;
#15929=LINE ( 'NONE', #15520, #10877 ) ;
#15931=DIRECTION ( 'NONE',  ( -0.000000000000000000, -0.000000000000000000, 1.000000000000000000 ) ) ;
#15938=CARTESIAN_POINT ( 'NONE',  ( 31.77187437101505196, 51.77076963420834232, 293.5832628385307999 ) ) ;
#15939=ORIENTED_EDGE ( 'NONE', *, *, #17969, .T. ) ;
#15941=VECTOR ( 'NONE', #12935, 1000.000000000000000 ) ;
#15942=LINE ( 'NONE', #8157, #10653 ) ;
#15945=CARTESIAN_POINT ( 'NONE',  ( 45.46712722958809394, -40.27908801170008246, 283.5832628385307999 ) ) ;
#15946=PLANE ( 'NONE',  #4833 ) ;
#15949=VERTEX_POINT ( 'NONE', #2265 ) ;
#15950=DIRECTION ( 'NONE',  ( -0.6427876096865456912, 0.7660444431189726844, 0.000000000000000000 ) ) ;
#15951=EDGE_LOOP ( 'NONE', ( #9281, #3426, #3442, #6140 ) ) ;
#15952=VECTOR ( 'NONE', #17143, 1000.000000000000227 ) ;
#15955=VECTOR ( 'NONE', #7230, 1000.000000000000000 ) ;
#15956=ORIENTED_EDGE ( 'NONE', *, *, #1883, .F. ) ;
#15957=FACE_OUTER_BOUND ( 'NONE', #13355, .T. ) ;
#15958=DIRECTION ( 'NONE',  ( -0.000000000000000000, -0.000000000000000000, 1.000000000000000000 ) ) ;
#15959=VERTEX_POINT ( 'NONE', #715 ) ;
#15961=DIRECTION ( 'NONE',  ( -0.000000000000000000, -0.000000000000000000, 1.000000000000000000 ) ) ;
#15962=DIRECTION ( 'NONE',  ( 0.000000000000000000, 0.000000000000000000, -1.000000000000000000 ) ) ;
#15963=DIRECTION ( 'NONE',  ( -0.000000000000000000, -0.000000000000000000, 1.000000000000000000 ) ) ;
#15965=VECTOR ( 'NONE', #2800, 1000.000000000000000 ) ;
#15966=CIRCLE ( 'NONE', #15647, 62.91752772691707207 ) ;
#15967=FACE_OUTER_BOUND ( 'NONE', #9535, .T. ) ;
#15968=FACE_OUTER_BOUND ( 'NONE', #13032, .T. ) ;
#15971=CARTESIAN_POINT ( 'NONE',  ( -59.42266395395758138, 50.93469132750324491, 110.7293897666001214 ) ) ;
#15972=DIRECTION ( 'NONE',  ( -0.000000000000000000, -0.000000000000000000, 1.000000000000000000 ) ) ;
#15973=CARTESIAN_POINT ( 'NONE',  ( -3.123743752084084058, 4.811834253409051243, 293.5832628385307999 ) ) ;
#15975=VERTEX_POINT ( 'NONE', #2658 ) ;
#15979=EDGE_LOOP ( 'NONE', ( #6089, #16006, #2224, #19084 ) ) ;
#15982=CIRCLE ( 'NONE', #7156, 62.91752772691707207 ) ;
#15985=ADVANCED_FACE ( 'NONE', ( #7062 ), #812, .F. ) ;
#15987=CARTESIAN_POINT ( 'NONE',  ( -5.590028426173815568, -1.289614712049183209, 293.5832628385307999 ) ) ;
#15989=CARTESIAN_POINT ( 'NONE',  ( -44.07268132743698175, -38.78191089773056177, 110.7293897666001214 ) ) ;
#15992=VECTOR ( 'NONE', #17937, 1000.000000000000000 ) ;
#15994=FACE_OUTER_BOUND ( 'NONE', #15951, .T. ) ;
#15998=LINE ( 'NONE', #18976, #10171 ) ;
#16000=AXIS2_PLACEMENT_3D ( 'NONE', #18755, #14135, #7796 ) ;
#16001=PLANE ( 'NONE',  #16510 ) ;
#16004=EDGE_CURVE ( 'NONE', #14853, #11236, #5525, .T. ) ;
#16006=ORIENTED_EDGE ( 'NONE', *, *, #2607, .T. ) ;
#16007=ORIENTED_EDGE ( 'NONE', *, *, #11670, .F. ) ;
#16011=LINE ( 'NONE', #13025, #16131 ) ;
#16013=LINE ( 'NONE', #17952, #2754 ) ;
#16023=CARTESIAN_POINT ( 'NONE',  ( 48.17797692984161984, 36.99387960884179449, 293.5832628385307999 ) ) ;
#16024=ADVANCED_FACE ( 'NONE', ( #13579 ), #16477, .F. ) ;
#16026=VECTOR ( 'NONE', #5447, 1000.000000000000000 ) ;
#16028=LINE ( 'NONE', #2010, #9681 ) ;
#16030=ORIENTED_EDGE ( 'NONE', *, *, #10607, .F. ) ;
#16032=ORIENTED_EDGE ( 'NONE', *, *, #9238, .F. ) ;
#16033=ADVANCED_FACE ( 'NONE', ( #4078 ), #8686, .F. ) ;
#16037=PLANE ( 'NONE',  #7634 ) ;
#16038=DIRECTION ( 'NONE',  ( -0.9848077530122062440, -0.1736481776669404620, 0.000000000000000000 ) ) ;
#16040=CIRCLE ( 'NONE', #3625, 62.91752772691707207 ) ;
#16041=DIRECTION ( 'NONE',  ( 0.000000000000000000, 0.000000000000000000, -1.000000000000000000 ) ) ;
#16042=CARTESIAN_POINT ( 'NONE',  ( -57.65577537092151772, 11.00103590902930328, 248.9926560891072143 ) ) ;
#16043=VERTEX_POINT ( 'NONE', #18103 ) ;
#16044=FACE_OUTER_BOUND ( 'NONE', #8670, .T. ) ;
#16045=CARTESIAN_POINT ( 'NONE',  ( 0.000000000000000000, 0.000000000000000000, 0.000000000000000000 ) ) ;
#16046=ADVANCED_FACE ( 'NONE', ( #12044 ), #19632, .F. ) ;
#16048=EDGE_CURVE ( 'NONE', #2266, #18696, #7925, .T. ) ;
#16051=CARTESIAN_POINT ( 'NONE',  ( -67.08601213326568313, -40.32479851956793482, 110.9660488491356887 ) ) ;
#16054=VERTEX_POINT ( 'NONE', #6035 ) ;
#16055=VECTOR ( 'NONE', #9597, 1000.000000000000000 ) ;
#16056=FACE_OUTER_BOUND ( 'NONE', #10320, .T. ) ;
#16057=EDGE_CURVE ( 'NONE', #9227, #17450, #9399, .T. ) ;
#16059=VECTOR ( 'NONE', #15172, 1000.000000000000000 ) ;
#16060=ORIENTED_EDGE ( 'NONE', *, *, #8886, .F. ) ;
#16061=FACE_OUTER_BOUND ( 'NONE', #15463, .T. ) ;
#16062=ORIENTED_EDGE ( 'NONE', *, *, #15277, .F. ) ;
#16065=FACE_OUTER_BOUND ( 'NONE', #7358, .T. ) ;
#16066=VERTEX_POINT ( 'NONE', #17185 ) ;
#16067=PRESENTATION_STYLE_ASSIGNMENT (( #12782 ) ) ;
#16068=LINE ( 'NONE', #14817, #6053 ) ;
#16069=CARTESIAN_POINT ( 'NONE',  ( 41.02350267428969488, 44.79940644582669051, 293.5832628385307999 ) ) ;
#16073=ORIENTED_EDGE ( 'NONE', *, *, #13903, .T. ) ;
#16077=DIRECTION ( 'NONE',  ( 0.000000000000000000, 0.000000000000000000, -1.000000000000000000 ) ) ;
#16079=CARTESIAN_POINT ( 'NONE',  ( -30.05702882063063086, -50.41613078340792242, 248.9926560891072143 ) ) ;
#16081=EDGE_LOOP ( 'NONE', ( #11895, #5477, #9876, #19153 ) ) ;
#16083=ORIENTED_EDGE ( 'NONE', *, *, #5759, .T. ) ;
#16086=DIRECTION ( 'NONE',  ( 0.3088643371590125142, -0.9511061040868803440, 0.000000000000000000 ) ) ;
#16088=VERTEX_POINT ( 'NONE', #13791 ) ;
#16089=VECTOR ( 'NONE', #5161, 1000.000000000000114 ) ;
#16095=DIRECTION ( 'NONE',  ( 0.4999999999999919509, 0.8660254037844432595, 0.000000000000000000 ) ) ;
#16096=DIRECTION ( 'NONE',  ( -0.4974449862757516216, 6.091944101944981818E-17, 0.8674955248467378643 ) ) ;
#16097=DIRECTION ( 'NONE',  ( -0.000000000000000000, -0.000000000000000000, 1.000000000000000000 ) ) ;
#16101=EDGE_LOOP ( 'NONE', ( #19453, #14241, #9729, #2544 ) ) ;
#16108=ORIENTED_EDGE ( 'NONE', *, *, #16534, .T. ) ;
#16110=DIRECTION ( 'NONE',  ( 0.000000000000000000, 0.000000000000000000, 1.000000000000000000 ) ) ;
#16111=CIRCLE ( 'NONE', #7282, 62.91752772691707207 ) ;
#16112=DIRECTION ( 'NONE',  ( 0.9848077530122097967, -0.1736481776669207000, 0.000000000000000000 ) ) ;
#16114=DIRECTION ( 'NONE',  ( 0.000000000000000000, 0.000000000000000000, 1.000000000000000000 ) ) ;
#16116=CARTESIAN_POINT ( 'NONE',  ( -9.564549117045515914, -62.18629025319810211, 293.5832628385307999 ) ) ;
#16117=PLANE ( 'NONE',  #17642 ) ;
#16119=CARTESIAN_POINT ( 'NONE',  ( 14.39940464655707331, 76.92888220842492331, 248.9926560891072143 ) ) ;
#16121=EDGE_CURVE ( 'NONE', #6626, #15899, #1318, .T. ) ;
#16127=CARTESIAN_POINT ( 'NONE',  ( -0.8220851292435327196, -78.26059000578311498, 112.7772637782949943 ) ) ;
#16128=EDGE_CURVE ( 'NONE', #13973, #6346, #9561, .T. ) ;
#16131=VECTOR ( 'NONE', #2299, 1000.000000000000000 ) ;
#16133=DIRECTION ( 'NONE',  ( 0.7660444431189771253, 0.6427876096865404731, 0.000000000000000000 ) ) ;
#16134=DIRECTION ( 'NONE',  ( -0.000000000000000000, -0.000000000000000000, 1.000000000000000000 ) ) ;
#16142=DIRECTION ( 'NONE',  ( -0.000000000000000000, -0.000000000000000000, 1.000000000000000000 ) ) ;
#16149=LINE ( 'NONE', #16347, #1719 ) ;
#16154=VECTOR ( 'NONE', #3653, 1000.000000000000227 ) ;
#16156=ORIENTED_EDGE ( 'NONE', *, *, #8781, .F. ) ;
#16160=EDGE_CURVE ( 'NONE', #11536, #8815, #1935, .T. ) ;
#16162=ADVANCED_FACE ( 'NONE', ( #292 ), #6547, .T. ) ;
#16163=EDGE_CURVE ( 'NONE', #274, #18902, #2192, .T. ) ;
#16164=LINE ( 'NONE', #3676, #4194 ) ;
#16169=DIRECTION ( 'NONE',  ( 0.6692498792541753394, 0.7430374143461900838, 0.000000000000000000 ) ) ;
#16170=CIRCLE ( 'NONE', #2119, 60.74260934110282051 ) ;
#16173=CARTESIAN_POINT ( 'NONE',  ( -12.14957802882752524, -59.51724408343569905, 283.5832628385307999 ) ) ;
#16174=CARTESIAN_POINT ( 'NONE',  ( 2.240720816136073434, -5.281164089014820817, 283.5832628385307999 ) ) ;
#16176=LINE ( 'NONE', #8388, #11113 ) ;
#16178=DIRECTION ( 'NONE',  ( -0.8830229359480271656, -0.4693298356057563625, 0.000000000000000000 ) ) ;
#16179=ORIENTED_EDGE ( 'NONE', *, *, #6776, .T. ) ;
#16184=VERTEX_POINT ( 'NONE', #4055 ) ;
#16186=EDGE_LOOP ( 'NONE', ( #4214, #14274, #2894, #19027 ) ) ;
#16191=EDGE_LOOP ( 'NONE', ( #13713, #217, #19831, #2938 ) ) ;
#16194=LINE ( 'NONE', #14558, #7631 ) ;
#16196=EDGE_LOOP ( 'NONE', ( #13448, #17926, #11660, #15228 ) ) ;
#16199=PLANE ( 'NONE',  #6908 ) ;
#16201=LINE ( 'NONE', #6983, #9190 ) ;
#16202=CARTESIAN_POINT ( 'NONE',  ( 51.77076963420847733, -31.77187437101486367, 283.5832628385307999 ) ) ;
#16207=ORIENTED_EDGE ( 'NONE', *, *, #8872, .T. ) ;
#16208=EDGE_LOOP ( 'NONE', ( #1459, #13257, #17862, #6921 ) ) ;
#16209=EDGE_LOOP ( 'NONE', ( #14668, #18163, #9251, #579 ) ) ;
#16210=DIRECTION ( 'NONE',  ( 0.000000000000000000, 0.000000000000000000, 1.000000000000000000 ) ) ;
#16213=DIRECTION ( 'NONE',  ( 0.7881095627315598540, 0.6155349844899715706, 0.000000000000000000 ) ) ;
#16216=ORIENTED_EDGE ( 'NONE', *, *, #14472, .F. ) ;
#16217=CIRCLE ( 'NONE', #6397, 60.74260934110282051 ) ;
#16218=DIRECTION ( 'NONE',  ( -0.9993852124581887875, 0.03505990758545545621, 0.000000000000000000 ) ) ;
#16220=LINE ( 'NONE', #18146, #3345 ) ;
#16221=CARTESIAN_POINT ( 'NONE',  ( -11.73417718768092044, -61.81362617575097573, 248.9926560891072143 ) ) ;
#16223=DIRECTION ( 'NONE',  ( 0.000000000000000000, 0.000000000000000000, 1.000000000000000000 ) ) ;
#16225=VECTOR ( 'NONE', #18552, 1000.000000000000000 ) ;
#16227=VERTEX_POINT ( 'NONE', #7134 ) ;
#16229=ORIENTED_EDGE ( 'NONE', *, *, #3519, .F. ) ;
#16230=EDGE_LOOP ( 'NONE', ( #17613, #816, #7789, #1974 ) ) ;
#16231=DIRECTION ( 'NONE',  ( -0.7660444431189726844, -0.6427876096865458022, 0.000000000000000000 ) ) ;
#16233=ORIENTED_EDGE ( 'NONE', *, *, #8420, .T. ) ;
#16234=EDGE_CURVE ( 'NONE', #16184, #9484, #11534, .T. ) ;
#16235=CARTESIAN_POINT ( 'NONE',  ( -32.62092819947992695, -51.24245927909985454, 293.5832628385307999 ) ) ;
#16236=ADVANCED_FACE ( 'NONE', ( #15094 ), #11721, .F. ) ;
#16239=EDGE_LOOP ( 'NONE', ( #19512, #4723, #3739, #3404 ) ) ;
#16240=CARTESIAN_POINT ( 'NONE',  ( 51.77251465595239921, -31.77296517111717478, 283.5832628385307999 ) ) ;
#16241=DIRECTION ( 'NONE',  ( 0.1736481776669404620, -0.9848077530122062440, 0.000000000000000000 ) ) ;
#16242=VECTOR ( 'NONE', #3876, 1000.000000000000000 ) ;
#16243=ORIENTED_EDGE ( 'NONE', *, *, #6270, .T. ) ;
#16244=CARTESIAN_POINT ( 'NONE',  ( 54.86954475316255042, -20.84572577951183092, 132.4711112102474146 ) ) ;
#16245=VECTOR ( 'NONE', #12595, 1000.000000000000000 ) ;
#16247=DIRECTION ( 'NONE',  ( 1.000000000000000000, 0.000000000000000000, 0.000000000000000000 ) ) ;
#16248=CARTESIAN_POINT ( 'NONE',  ( 49.67518383744835120, -60.47951622432767493, 110.7293897666001214 ) ) ;
#16249=AXIS2_PLACEMENT_3D ( 'NONE', #4616, #17096, #10433 ) ;
#16250=ADVANCED_FACE ( 'NONE', ( #1076 ), #14999, .F. ) ;
#16254=DIRECTION ( 'NONE',  ( -0.000000000000000000, -0.000000000000000000, 1.000000000000000000 ) ) ;
#16255=ORIENTED_EDGE ( 'NONE', *, *, #16914, .F. ) ;
#16257=CARTESIAN_POINT ( 'NONE',  ( 51.77251465595239921, -31.77296517111717478, 293.5832628385307999 ) ) ;
#16258=ORIENTED_EDGE ( 'NONE', *, *, #9916, .T. ) ;
#16260=DIRECTION ( 'NONE',  ( 1.000000000000000000, 0.000000000000000000, 0.000000000000000000 ) ) ;
#16262=ORIENTED_EDGE ( 'NONE', *, *, #9559, .F. ) ;
#16263=ADVANCED_FACE ( 'NONE', ( #3758 ), #10193, .F. ) ;
#16264=DIRECTION ( 'NONE',  ( 0.000000000000000000, 0.000000000000000000, 1.000000000000000000 ) ) ;
#16265=VECTOR ( 'NONE', #1005, 1000.000000000000000 ) ;
#16267=VECTOR ( 'NONE', #6517, 1000.000000000000114 ) ;
#16268=DIRECTION ( 'NONE',  ( 1.000000000000000000, 0.000000000000000000, 0.000000000000000000 ) ) ;
#16269=DIRECTION ( 'NONE',  ( -0.000000000000000000, -0.000000000000000000, 1.000000000000000000 ) ) ;
#16270=VERTEX_POINT ( 'NONE', #13249 ) ;
#16276=FACE_OUTER_BOUND ( 'NONE', #19943, .T. ) ;
#16277=EDGE_CURVE ( 'NONE', #2315, #10541, #10000, .T. ) ;
#16279=DIRECTION ( 'NONE',  ( 0.8660254037844397068, -0.4999999999999978906, 0.000000000000000000 ) ) ;
#16280=VECTOR ( 'NONE', #17353, 1000.000000000000000 ) ;
#16282=ORIENTED_EDGE ( 'NONE', *, *, #16874, .T. ) ;
#16285=PLANE ( 'NONE',  #19230 ) ;
#16287=ORIENTED_EDGE ( 'NONE', *, *, #1860, .F. ) ;
#16288=ORIENTED_EDGE ( 'NONE', *, *, #18426, .F. ) ;
#16290=ADVANCED_BREP_SHAPE_REPRESENTATION ( '', ( #8201, #18639 ), #8174 ) ;
#16293=CARTESIAN_POINT ( 'NONE',  ( 57.92709869106709419, 18.28567271940532990, 293.5832628385307999 ) ) ;
#16294=EDGE_LOOP ( 'NONE', ( #861, #6567, #1188, #8876 ) ) ;
#16295=CARTESIAN_POINT ( 'NONE',  ( 0.000000000000000000, 0.000000000000000000, 293.5832628385307999 ) ) ;
#16297=VERTEX_POINT ( 'NONE', #19606 ) ;
#16302=LINE ( 'NONE', #8516, #16423 ) ;
#16304=ADVANCED_FACE ( 'NONE', ( #11629 ), #8562, .F. ) ;
#16306=CARTESIAN_POINT ( 'NONE',  ( 1.379293853801755176, -62.90240729679781850, 248.9926560891072143 ) ) ;
#16307=DIRECTION ( 'NONE',  ( 0.6155349844899715706, -0.7881095627315598540, 0.000000000000000000 ) ) ;
#16308=ORIENTED_EDGE ( 'NONE', *, *, #4772, .T. ) ;
#16314=CIRCLE ( 'NONE', #1268, 60.74260934110282051 ) ;
#16315=VERTEX_POINT ( 'NONE', #5800 ) ;
#16318=PLANE ( 'NONE',  #13665 ) ;
#16319=CARTESIAN_POINT ( 'NONE',  ( -67.36461649554505016, 39.84224160888970800, 132.4711112102474146 ) ) ;
#16320=VECTOR ( 'NONE', #5487, 1000.000000000000000 ) ;
#16321=CARTESIAN_POINT ( 'NONE',  ( -60.47951622432784546, -49.67518383744813804, 248.9926560891072143 ) ) ;
#16325=DIRECTION ( 'NONE',  ( -0.8660254037844345998, -0.5000000000000069944, 0.000000000000000000 ) ) ;
#16326=ORIENTED_EDGE ( 'NONE', *, *, #7039, .T. ) ;
#16327=VERTEX_POINT ( 'NONE', #13765 ) ;
#16329=VECTOR ( 'NONE', #10518, 1000.000000000000000 ) ;
#16335=FACE_OUTER_BOUND ( 'NONE', #8937, .T. ) ;
#16336=DIRECTION ( 'NONE',  ( 1.000000000000000000, 0.000000000000000000, 0.000000000000000000 ) ) ;
#16339=LINE ( 'NONE', #16042, #6839 ) ;
#16340=ORIENTED_EDGE ( 'NONE', *, *, #8347, .T. ) ;
#16341=CARTESIAN_POINT ( 'NONE',  ( 12.28122767885846400, -61.70726652483822505, 248.9926560891072143 ) ) ;
#16343=PLANE ( 'NONE',  #4541 ) ;
#16345=LINE ( 'NONE', #18170, #2320 ) ;
#16347=CARTESIAN_POINT ( 'NONE',  ( 0.4239815141812912636, -0.2650276884262227628, 283.5832628385307999 ) ) ;
#16348=CARTESIAN_POINT ( 'NONE',  ( -14.39940464655760799, -76.92888220842480962, 112.0427633081292385 ) ) ;
#16350=EDGE_CURVE ( 'NONE', #19334, #9538, #7426, .T. ) ;
#16351=CARTESIAN_POINT ( 'NONE',  ( -13.12769224524071277, -59.30917539369501412, 283.5832628385307999 ) ) ;
#16354=VECTOR ( 'NONE', #7983, 1000.000000000000000 ) ;
#16355=LINE ( 'NONE', #7045, #9586 ) ;
#16356=ORIENTED_EDGE ( 'NONE', *, *, #9238, .T. ) ;
#16357=ORIENTED_EDGE ( 'NONE', *, *, #7524, .F. ) ;
#16358=ADVANCED_FACE ( 'NONE', ( #9165 ), #6007, .T. ) ;
#16359=VECTOR ( 'NONE', #17049, 1000.000000000000000 ) ;
#16360=DIRECTION ( 'NONE',  ( 0.1736481776669306920, -0.9848077530122080203, 0.000000000000000000 ) ) ;
#16367=ORIENTED_EDGE ( 'NONE', *, *, #11850, .T. ) ;
#16371=DIRECTION ( 'NONE',  ( -0.3420201433256726542, 0.9396926207859069846, 0.000000000000000000 ) ) ;
#16372=AXIS2_PLACEMENT_3D ( 'NONE', #8460, #17385, #386 ) ;
#16375=DIRECTION ( 'NONE',  ( 0.000000000000000000, 0.000000000000000000, -1.000000000000000000 ) ) ;
#16376=CONICAL_SURFACE ( 'NONE', #11791, 17.50000000000001066, 0.7853981633974479459 ) ;
#16377=DIRECTION ( 'NONE',  ( 0.000000000000000000, 0.000000000000000000, -1.000000000000000000 ) ) ;
#16378=ORIENTED_EDGE ( 'NONE', *, *, #15177, .T. ) ;
#16379=EDGE_CURVE ( 'NONE', #11697, #2515, #4356, .T. ) ;
#16381=CARTESIAN_POINT ( 'NONE',  ( -57.61627707419551570, -19.23614321207253042, 293.5832628385307999 ) ) ;
#16383=ORIENTED_EDGE ( 'NONE', *, *, #3968, .T. ) ;
#16388=ORIENTED_EDGE ( 'NONE', *, *, #16121, .T. ) ;
#16389=EDGE_CURVE ( 'NONE', #12180, #55, #4256, .T. ) ;
#16393=EDGE_CURVE ( 'NONE', #20158, #16054, #9272, .T. ) ;
#16395=FACE_OUTER_BOUND ( 'NONE', #9198, .T. ) ;
#16396=CARTESIAN_POINT ( 'NONE',  ( 11.54977938102087620, -57.55901709132175625, 112.0427633081291816 ) ) ;
#16397=LINE ( 'NONE', #18122, #17428 ) ;
#16399=CARTESIAN_POINT ( 'NONE',  ( 59.42266395395792955, -50.93469132750283279, 132.4711112102474146 ) ) ;
#16401=ADVANCED_FACE ( 'NONE', ( #17052 ), #18586, .F. ) ;
#16403=LINE ( 'NONE', #2581, #13450 ) ;
#16404=ORIENTED_EDGE ( 'NONE', *, *, #1615, .T. ) ;
#16406=ORIENTED_EDGE ( 'NONE', *, *, #18932, .F. ) ;
#16407=CARTESIAN_POINT ( 'NONE',  ( -44.79787735033389851, 41.02212542604627998, 293.5832628385307999 ) ) ;
#16408=ORIENTED_EDGE ( 'NONE', *, *, #17980, .T. ) ;
#16409=ADVANCED_FACE ( 'NONE', ( #19803 ), #3039, .F. ) ;
#16411=CARTESIAN_POINT ( 'NONE',  ( -0.8220851292435327196, -78.26059000578311498, 132.4711112102474146 ) ) ;
#16414=LINE ( 'NONE', #3529, #18115 ) ;
#16416=CARTESIAN_POINT ( 'NONE',  ( -74.01264520835137262, 25.47058595421628269, 111.4180192758973931 ) ) ;
#16418=LINE ( 'NONE', #19290, #10409 ) ;
#16421=VECTOR ( 'NONE', #11587, 1000.000000000000227 ) ;
#16423=VECTOR ( 'NONE', #14752, 1000.000000000000000 ) ;
#16425=CARTESIAN_POINT ( 'NONE',  ( -79.75827554147308263, 9.767571684737763671E-15, 132.4711112102474146 ) ) ;
#16426=ORIENTED_EDGE ( 'NONE', *, *, #605, .F. ) ;
#16427=CIRCLE ( 'NONE', #4998, 62.91752772691707207 ) ;
#16428=VECTOR ( 'NONE', #4100, 1000.000000000000114 ) ;
#16431=ORIENTED_EDGE ( 'NONE', *, *, #999, .T. ) ;
#16441=DIRECTION ( 'NONE',  ( -0.000000000000000000, -0.000000000000000000, 1.000000000000000000 ) ) ;
#16442=PLANE ( 'NONE',  #939 ) ;
#16443=EDGE_CURVE ( 'NONE', #11539, #1303, #17159, .T. ) ;
#16445=DIRECTION ( 'NONE',  ( 0.000000000000000000, 0.000000000000000000, 1.000000000000000000 ) ) ;
#16448=CARTESIAN_POINT ( 'NONE',  ( 49.24833719034187851, 60.83768308848395634, 132.4711112102474146 ) ) ;
#16449=VECTOR ( 'NONE', #1322, 1000.000000000000000 ) ;
#16450=VECTOR ( 'NONE', #8548, 1000.000000000000000 ) ;
#16454=CARTESIAN_POINT ( 'NONE',  ( 0.000000000000000000, 0.000000000000000000, 293.5832628385307999 ) ) ;
#16455=ORIENTED_EDGE ( 'NONE', *, *, #9118, .T. ) ;
#16456=VECTOR ( 'NONE', #13975, 999.9999999999998863 ) ;
#16457=ORIENTED_EDGE ( 'NONE', *, *, #11824, .F. ) ;
#16459=VECTOR ( 'NONE', #1116, 1000.000000000000227 ) ;
#16461=LINE ( 'NONE', #18185, #12680 ) ;
#16462=CARTESIAN_POINT ( 'NONE',  ( 0.000000000000000000, 0.000000000000000000, 293.5832628385307999 ) ) ;
#16468=DIRECTION ( 'NONE',  ( 1.000000000000000000, 0.000000000000000000, 0.000000000000000000 ) ) ;
#16472=CARTESIAN_POINT ( 'NONE',  ( 18.28567271940513450, -57.92709869106715814, 293.5832628385307999 ) ) ;
#16474=VECTOR ( 'NONE', #4688, 1000.000000000000000 ) ;
#16477=PLANE ( 'NONE',  #2706 ) ;
#16479=EDGE_CURVE ( 'NONE', #11921, #13055, #9358, .T. ) ;
#16480=DIRECTION ( 'NONE',  ( 1.000000000000000000, 0.000000000000000000, 0.000000000000000000 ) ) ;
#16481=CARTESIAN_POINT ( 'NONE',  ( 0.000000000000000000, 0.000000000000000000, 283.5832628385307999 ) ) ;
#16482=EDGE_LOOP ( 'NONE', ( #18857, #4575, #6785, #15764 ) ) ;
#16493=DIRECTION ( 'NONE',  ( 0.7430374143461878633, -0.6692498792541777819, 0.000000000000000000 ) ) ;
#16494=CARTESIAN_POINT ( 'NONE',  ( 3.453261854573022482, 4.581103194070020201, 293.5832628385307999 ) ) ;
#16496=CIRCLE ( 'NONE', #4407, 79.75827554147308263 ) ;
#16497=CARTESIAN_POINT ( 'NONE',  ( 59.06449708980161972, 51.36153797460926995, 132.4711112102474146 ) ) ;
#16499=DIRECTION ( 'NONE',  ( 0.000000000000000000, 0.000000000000000000, 1.000000000000000000 ) ) ;
#16506=AXIS2_PLACEMENT_3D ( 'NONE', #16856, #2849, #7152 ) ;
#16508=CARTESIAN_POINT ( 'NONE',  ( -0.8220851292435327196, -78.26059000578311498, 248.9926560891072143 ) ) ;
#16509=ORIENTED_EDGE ( 'NONE', *, *, #9627, .F. ) ;
#16510=AXIS2_PLACEMENT_3D ( 'NONE', #10056, #16307, #2290 ) ;
#16512=EDGE_CURVE ( 'NONE', #7714, #2316, #17467, .T. ) ;
#16515=CARTESIAN_POINT ( 'NONE',  ( -60.22029172860436574, -7.948651060879222463, 293.5832628385307999 ) ) ;
#16517=PLANE ( 'NONE',  #9457 ) ;
#16519=DIRECTION ( 'NONE',  ( -0.8660254037844328234, -0.5000000000000101030, -0.000000000000000000 ) ) ;
#16523=ORIENTED_EDGE ( 'NONE', *, *, #5904, .F. ) ;
#16524=EDGE_CURVE ( 'NONE', #15095, #13722, #1906, .T. ) ;
#16525=EDGE_CURVE ( 'NONE', #998, #2414, #16028, .T. ) ;
#16526=ADVANCED_FACE ( 'NONE', ( #14481 ), #9871, .T. ) ;
#16527=ORIENTED_EDGE ( 'NONE', *, *, #8135, .F. ) ;
#16531=EDGE_LOOP ( 'NONE', ( #11489, #10109, #2518 ) ) ;
#16532=VECTOR ( 'NONE', #2848, 1000.000000000000000 ) ;
#16533=CARTESIAN_POINT ( 'NONE',  ( 59.42266395395792955, -50.93469132750283279, 248.9926560891072143 ) ) ;
#16534=EDGE_CURVE ( 'NONE', #15414, #739, #7831, .T. ) ;
#16537=EDGE_LOOP ( 'NONE', ( #10112, #7611, #6400, #15577 ) ) ;
#16538=DIRECTION ( 'NONE',  ( 1.000000000000000000, 0.000000000000000000, 0.000000000000000000 ) ) ;
#16540=ORIENTED_EDGE ( 'NONE', *, *, #18405, .F. ) ;
#16541=CARTESIAN_POINT ( 'NONE',  ( 0.000000000000000000, 0.000000000000000000, 132.4711112102474146 ) ) ;
#16546=VECTOR ( 'NONE', #15522, 1000.000000000000000 ) ;
#16547=EDGE_CURVE ( 'NONE', #274, #14568, #15718, .T. ) ;
#16548=CARTESIAN_POINT ( 'NONE',  ( -59.42266395395758138, 50.93469132750324491, 248.9926560891072143 ) ) ;
#16554=ADVANCED_FACE ( 'NONE', ( #2983 ), #8901, .F. ) ;
#16557=ORIENTED_EDGE ( 'NONE', *, *, #9353, .F. ) ;
#16558=VECTOR ( 'NONE', #19598, 1000.000000000000000 ) ;
#16560=VECTOR ( 'NONE', #4088, 1000.000000000000000 ) ;
#16568=CARTESIAN_POINT ( 'NONE',  ( -0.8220851292435327196, -62.91215678473957240, 293.5832628385307999 ) ) ;
#16570=ORIENTED_EDGE ( 'NONE', *, *, #19389, .T. ) ;
#16572=LINE ( 'NONE', #11839, #19932 ) ;
#16573=DIRECTION ( 'NONE',  ( -1.000000000000000000, -1.047444401652940164E-14, 0.000000000000000000 ) ) ;
#16574=ORIENTED_EDGE ( 'NONE', *, *, #15882, .F. ) ;
#16575=DIRECTION ( 'NONE',  ( 0.6692498792541753394, 0.7430374143461900838, 0.000000000000000000 ) ) ;
#16576=DIRECTION ( 'NONE',  ( 1.000000000000000000, 0.000000000000000000, 0.000000000000000000 ) ) ;
#16580=CIRCLE ( 'NONE', #8071, 62.91752772691707207 ) ;
#16585=DIRECTION ( 'NONE',  ( 0.000000000000000000, 0.000000000000000000, -1.000000000000000000 ) ) ;
#16586=CIRCLE ( 'NONE', #11671, 62.91752772691707207 ) ;
#16587=CARTESIAN_POINT ( 'NONE',  ( 11.00103590902871353, 57.65577537092163851, 132.4711112102474146 ) ) ;
#16588=VECTOR ( 'NONE', #14998, 999.9999999999998863 ) ;
#16590=CARTESIAN_POINT ( 'NONE',  ( -14.94814811854910452, 76.83212392882506947, 248.9926560891072143 ) ) ;
#16591=CARTESIAN_POINT ( 'NONE',  ( -0.2993243175131807821, 5.729042578294318844, 293.5832628385307999 ) ) ;
#16599=ORIENTED_EDGE ( 'NONE', *, *, #15915, .T. ) ;
#16601=CARTESIAN_POINT ( 'NONE',  ( 45.48770046196260353, 37.09555676057011908, 248.9926560891072143 ) ) ;
#16602=ORIENTED_EDGE ( 'NONE', *, *, #8168, .T. ) ;
#16603=EDGE_CURVE ( 'NONE', #4103, #14479, #15146, .T. ) ;
#16607=ADVANCED_FACE ( 'NONE', ( #4408 ), #7370, .F. ) ;
#16610=PLANE ( 'NONE',  #4441 ) ;
#16611=CARTESIAN_POINT ( 'NONE',  ( 57.92709869106709419, 18.28567271940532990, 283.5832628385307999 ) ) ;
#16616=DIRECTION ( 'NONE',  ( 0.7660444431189771253, 0.6427876096865405842, 0.000000000000000000 ) ) ;
#16617=CIRCLE ( 'NONE', #10387, 60.74260934110282051 ) ;
#16620=CIRCLE ( 'NONE', #5194, 60.74260934110282051 ) ;
#16621=CARTESIAN_POINT ( 'NONE',  ( -1.678175111358135130, -5.485913980968154746, 283.5832628385307999 ) ) ;
#16622=EDGE_LOOP ( 'NONE', ( #8828, #7261, #12446, #7153 ) ) ;
#16625=ORIENTED_EDGE ( 'NONE', *, *, #19400, .F. ) ;
#16628=ORIENTED_EDGE ( 'NONE', *, *, #860, .T. ) ;
#16630=VECTOR ( 'NONE', #3559, 1000.000000000000114 ) ;
#16631=LINE ( 'NONE', #5889, #4381 ) ;
#16633=ORIENTED_EDGE ( 'NONE', *, *, #6814, .F. ) ;
#16634=EDGE_CURVE ( 'NONE', #6667, #8663, #6112, .T. ) ;
#16637=EDGE_CURVE ( 'NONE', #7405, #3935, #16690, .T. ) ;
#16638=ORIENTED_EDGE ( 'NONE', *, *, #15684, .F. ) ;
#16640=CARTESIAN_POINT ( 'NONE',  ( -41.02212542604613787, -44.79787735033403351, 283.5832628385307999 ) ) ;
#16642=CARTESIAN_POINT ( 'NONE',  ( -77.21438937758510690, -12.78021302872823384, 248.9926560891072143 ) ) ;
#16646=AXIS2_PLACEMENT_3D ( 'NONE', #15065, #7293, #10165 ) ;
#16648=ADVANCED_FACE ( 'NONE', ( #9003 ), #15244, .T. ) ;
#16649=FACE_OUTER_BOUND ( 'NONE', #13362, .T. ) ;
#16650=ORIENTED_EDGE ( 'NONE', *, *, #1218, .F. ) ;
#16651=ORIENTED_EDGE ( 'NONE', *, *, #13114, .T. ) ;
#16652=FACE_OUTER_BOUND ( 'NONE', #17008, .T. ) ;
#16653=ORIENTED_EDGE ( 'NONE', *, *, #7524, .T. ) ;
#16654=ORIENTED_EDGE ( 'NONE', *, *, #9464, .T. ) ;
#16655=CARTESIAN_POINT ( 'NONE',  ( -53.78543575132152199, -32.64570716507522263, 248.9926560891072143 ) ) ;
#16659=CARTESIAN_POINT ( 'NONE',  ( 14.39940464655707331, 76.92888220842492331, 132.4711112102474146 ) ) ;
#16660=CARTESIAN_POINT ( 'NONE',  ( 38.41834839689379777, -68.18670162478818497, 110.9660488491356887 ) ) ;
#16661=ADVANCED_FACE ( 'NONE', ( #18431 ), #18528, .T. ) ;
#16662=ORIENTED_EDGE ( 'NONE', *, *, #15024, .T. ) ;
#16663=CARTESIAN_POINT ( 'NONE',  ( -9.564549117045519466, -62.18629025319811632, 248.9926560891072143 ) ) ;
#16666=DIRECTION ( 'NONE',  ( -0.000000000000000000, -0.000000000000000000, 1.000000000000000000 ) ) ;
#16667=EDGE_LOOP ( 'NONE', ( #17633, #8244, #15699, #6644 ) ) ;
#16668=CARTESIAN_POINT ( 'NONE',  ( 0.000000000000000000, 0.000000000000000000, 283.5832628385307999 ) ) ;
#16671=VERTEX_POINT ( 'NONE', #16997 ) ;
#16672=AXIS2_PLACEMENT_3D ( 'NONE', #14436, #6670, #9624 ) ;
#16677=AXIS2_PLACEMENT_3D ( 'NONE', #8803, #4612, #5843 ) ;
#16680=ORIENTED_EDGE ( 'NONE', *, *, #16603, .F. ) ;
#16681=DIRECTION ( 'NONE',  ( -0.7660444431189813441, 0.6427876096865353661, 0.000000000000000000 ) ) ;
#16682=CARTESIAN_POINT ( 'NONE',  ( -78.26059000578311498, -1.379293853802028291, 112.7772637782949516 ) ) ;
#16683=ORIENTED_EDGE ( 'NONE', *, *, #10379, .T. ) ;
#16686=VECTOR ( 'NONE', #17091, 1000.000000000000000 ) ;
#16687=EDGE_CURVE ( 'NONE', #16956, #9432, #11001, .T. ) ;
#16688=DIRECTION ( 'NONE',  ( -0.000000000000000000, -0.000000000000000000, 1.000000000000000000 ) ) ;
#16690=LINE ( 'NONE', #3085, #1537 ) ;
#16691=DIRECTION ( 'NONE',  ( -0.000000000000000000, -0.000000000000000000, 1.000000000000000000 ) ) ;
#16693=ORIENTED_EDGE ( 'NONE', *, *, #9616, .T. ) ;
#16694=DIRECTION ( 'NONE',  ( 0.7660444431189749048, 0.6427876096865430267, 0.000000000000000000 ) ) ;
#16695=DIRECTION ( 'NONE',  ( -0.000000000000000000, -0.000000000000000000, 1.000000000000000000 ) ) ;
#16696=ORIENTED_EDGE ( 'NONE', *, *, #16048, .F. ) ;
#16698=ORIENTED_EDGE ( 'NONE', *, *, #480, .F. ) ;
#16705=CARTESIAN_POINT ( 'NONE',  ( 41.48948842197119546, -47.29944656917769663, 132.4711112102474146 ) ) ;
#16706=CARTESIAN_POINT ( 'NONE',  ( -8.833100819207983179, -58.03804081968163331, 112.0427633081292385 ) ) ;
#16709=ADVANCED_FACE ( 'NONE', ( #19144 ), #110, .T. ) ;
#16710=VERTEX_POINT ( 'NONE', #9424 ) ;
#16715=DIRECTION ( 'NONE',  ( 1.000000000000000000, 0.000000000000000000, 0.000000000000000000 ) ) ;
#16716=DIRECTION ( 'NONE',  ( 0.8660254037844363761, 0.5000000000000039968, 0.000000000000000000 ) ) ;
#16717=ORIENTED_EDGE ( 'NONE', *, *, #16350, .F. ) ;
#16720=ADVANCED_FACE ( 'NONE', ( #12476 ), #18740, .F. ) ;
#16724=CARTESIAN_POINT ( 'NONE',  ( -77.21438937758510690, -12.78021302872823384, 248.9926560891072143 ) ) ;
#16726=ORIENTED_EDGE ( 'NONE', *, *, #6092, .T. ) ;
#16729=DIRECTION ( 'NONE',  ( -0.000000000000000000, -0.000000000000000000, 1.000000000000000000 ) ) ;
#16733=DIRECTION ( 'NONE',  ( -0.000000000000000000, -0.000000000000000000, 1.000000000000000000 ) ) ;
#16734=CARTESIAN_POINT ( 'NONE',  ( -2.240720816136038795, 5.281164089014786178, 293.5832628385307999 ) ) ;
#16738=ADVANCED_FACE ( 'NONE', ( #15669 ), #2062, .F. ) ;
#16740=VECTOR ( 'NONE', #495, 1000.000000000000000 ) ;
#16742=ORIENTED_EDGE ( 'NONE', *, *, #2785, .F. ) ;
#16743=VERTEX_POINT ( 'NONE', #7881 ) ;
#16746=ORIENTED_EDGE ( 'NONE', *, *, #8164, .F. ) ;
#16748=DIRECTION ( 'NONE',  ( 1.000000000000000000, 0.000000000000000000, 0.000000000000000000 ) ) ;
#16749=CYLINDRICAL_SURFACE ( 'NONE', #17462, 62.91752772691707207 ) ;
#16752=DIRECTION ( 'NONE',  ( 1.000000000000000000, 0.000000000000000000, 0.000000000000000000 ) ) ;
#16753=DIRECTION ( 'NONE',  ( -0.000000000000000000, -0.000000000000000000, 1.000000000000000000 ) ) ;
#16754=ORIENTED_EDGE ( 'NONE', *, *, #13456, .F. ) ;
#16759=AXIS2_PLACEMENT_3D ( 'NONE', #15366, #7800, #17014 ) ;
#16760=DIRECTION ( 'NONE',  ( -0.000000000000000000, -0.000000000000000000, 1.000000000000000000 ) ) ;
#16763=VECTOR ( 'NONE', #5312, 1000.000000000000000 ) ;
#16764=DIRECTION ( 'NONE',  ( -0.9396926207859105373, 0.3420201433256631063, 0.000000000000000000 ) ) ;
#16766=VERTEX_POINT ( 'NONE', #11255 ) ;
#16767=DIRECTION ( 'NONE',  ( 0.000000000000000000, 0.000000000000000000, -1.000000000000000000 ) ) ;
#16768=DIRECTION ( 'NONE',  ( -0.000000000000000000, -0.000000000000000000, 1.000000000000000000 ) ) ;
#16771=EDGE_CURVE ( 'NONE', #4517, #55, #7407, .T. ) ;
#16772=ORIENTED_EDGE ( 'NONE', *, *, #3621, .F. ) ;
#16773=ADVANCED_FACE ( 'NONE', ( #12687 ), #14122, .T. ) ;
#16776=VECTOR ( 'NONE', #11726, 1000.000000000000227 ) ;
#16778=CARTESIAN_POINT ( 'NONE',  ( -50.93469132750304595, -59.42266395395774481, 248.9926560891072143 ) ) ;
#16780=VERTEX_POINT ( 'NONE', #1959 ) ;
#16781=VECTOR ( 'NONE', #16231, 999.9999999999998863 ) ;
#16784=ADVANCED_FACE ( 'NONE', ( #12888 ), #17314, .T. ) ;
#16786=PLANE ( 'NONE',  #16677 ) ;
#16787=LINE ( 'NONE', #7954, #18334 ) ;
#16789=DIRECTION ( 'NONE',  ( 1.000000000000000000, 0.000000000000000000, 0.000000000000000000 ) ) ;
#16790=DIRECTION ( 'NONE',  ( 0.8660254037844397068, -0.4999999999999978906, 0.000000000000000000 ) ) ;
#16792=EDGE_LOOP ( 'NONE', ( #4138, #14790, #14107 ) ) ;
#16793=CARTESIAN_POINT ( 'NONE',  ( -31.77296517111735596, -51.77251465595229263, 293.5832628385307999 ) ) ;
#16795=EDGE_CURVE ( 'NONE', #4103, #13430, #2200, .T. ) ;
#16800=VERTEX_POINT ( 'NONE', #416 ) ;
#16802=FACE_BOUND ( 'NONE', #19339, .T. ) ;
#16803=ORIENTED_EDGE ( 'NONE', *, *, #5616, .F. ) ;
#16804=LINE ( 'NONE', #6923, #15116 ) ;
#16807=DIRECTION ( 'NONE',  ( -0.1736481776669241417, -0.9848077530122091305, 0.000000000000000000 ) ) ;
#16809=VECTOR ( 'NONE', #6666, 1000.000000000000000 ) ;
#16811=ORIENTED_EDGE ( 'NONE', *, *, #6165, .T. ) ;
#16812=PLANE ( 'NONE',  #11407 ) ;
#16815=LINE ( 'NONE', #2807, #4966 ) ;
#16818=ORIENTED_EDGE ( 'NONE', *, *, #12878, .T. ) ;
#16819=CARTESIAN_POINT ( 'NONE',  ( -55.43188410062182925, -19.30071112029661151, 111.4180192758973931 ) ) ;
#16823=ORIENTED_EDGE ( 'NONE', *, *, #11425, .T. ) ;
#16828=DIRECTION ( 'NONE',  ( 0.000000000000000000, -1.000000000000000000, -0.000000000000000000 ) ) ;
#16832=CARTESIAN_POINT ( 'NONE',  ( 0.000000000000000000, 0.000000000000000000, 132.4711112102474146 ) ) ;
#16834=DIRECTION ( 'NONE',  ( 0.000000000000000000, 0.000000000000000000, 1.000000000000000000 ) ) ;
#16835=DIRECTION ( 'NONE',  ( 0.000000000000000000, 0.000000000000000000, 1.000000000000000000 ) ) ;
#16837=FACE_OUTER_BOUND ( 'NONE', #4571, .T. ) ;
#16838=CARTESIAN_POINT ( 'NONE',  ( 12.14914984460760827, 59.51523122377248853, 293.5832628385307999 ) ) ;
#16839=CARTESIAN_POINT ( 'NONE',  ( 53.40245231972179596, 28.94983032429848535, 293.5832628385307999 ) ) ;
#16840=VECTOR ( 'NONE', #3748, 999.9999999999998863 ) ;
#16842=EDGE_LOOP ( 'NONE', ( #1430, #12143, #9013, #10707 ) ) ;
#16844=VERTEX_POINT ( 'NONE', #9623 ) ;
#16846=EDGE_LOOP ( 'NONE', ( #10774, #14690, #2999 ) ) ;
#16847=ADVANCED_FACE ( 'NONE', ( #207 ), #18517, .T. ) ;
#16849=VERTEX_POINT ( 'NONE', #5427 ) ;
#16850=ORIENTED_EDGE ( 'NONE', *, *, #10904, .F. ) ;
#16851=LINE ( 'NONE', #7637, #13663 ) ;
#16853=CARTESIAN_POINT ( 'NONE',  ( -57.61627707419551570, -19.23614321207253042, 283.5832628385307999 ) ) ;
#16856=CARTESIAN_POINT ( 'NONE',  ( 0.000000000000000000, 0.000000000000000000, 293.5832628385307999 ) ) ;
#16861=CARTESIAN_POINT ( 'NONE',  ( -32.61983739937762294, -51.24071425735592555, 283.5832628385307999 ) ) ;
#16865=DIRECTION ( 'NONE',  ( -0.000000000000000000, -0.000000000000000000, 1.000000000000000000 ) ) ;
#16870=DIRECTION ( 'NONE',  ( -0.9511061040868804550, -0.3088643371590125697, 0.000000000000000000 ) ) ;
#16874=EDGE_CURVE ( 'NONE', #1487, #16315, #233, .T. ) ;
#16877=ORIENTED_EDGE ( 'NONE', *, *, #11408, .F. ) ;
#16879=VECTOR ( 'NONE', #4459, 1000.000000000000000 ) ;
#16881=EDGE_LOOP ( 'NONE', ( #570, #3628, #16653, #3746 ) ) ;
#16884=EDGE_CURVE ( 'NONE', #9325, #11965, #19628, .T. ) ;
#16886=EDGE_CURVE ( 'NONE', #15284, #18381, #10026, .T. ) ;
#16888=DIRECTION ( 'NONE',  ( 1.000000000000000000, 0.000000000000000000, -0.000000000000000000 ) ) ;
#16895=AXIS2_PLACEMENT_3D ( 'NONE', #12275, #12171, #1548 ) ;
#16897=LINE ( 'NONE', #9112, #10538 ) ;
#16898=EDGE_LOOP ( 'NONE', ( #16948, #17855, #11977 ) ) ;
#16903=FACE_BOUND ( 'NONE', #18088, .T. ) ;
#16904=ORIENTED_EDGE ( 'NONE', *, *, #15739, .F. ) ;
#16905=CARTESIAN_POINT ( 'NONE',  ( -12.14914984460759761, -59.51523122377249564, 283.5832628385307999 ) ) ;
#16906=DIRECTION ( 'NONE',  ( -0.000000000000000000, -0.000000000000000000, 1.000000000000000000 ) ) ;
#16908=VECTOR ( 'NONE', #16865, 1000.000000000000000 ) ;
#16910=VECTOR ( 'NONE', #17664, 1000.000000000000000 ) ;
#16912=EDGE_CURVE ( 'NONE', #19503, #7379, #19442, .T. ) ;
#16914=EDGE_CURVE ( 'NONE', #16227, #15975, #6956, .T. ) ;
#16915=ORIENTED_EDGE ( 'NONE', *, *, #12864, .F. ) ;
#16916=CARTESIAN_POINT ( 'NONE',  ( 73.06915264522001507, 28.06281046684300406, 132.4711112102474146 ) ) ;
#16917=DIRECTION ( 'NONE',  ( 1.000000000000000000, 0.000000000000000000, 0.000000000000000000 ) ) ;
#16919=DIRECTION ( 'NONE',  ( -0.7660444431189749048, -0.6427876096865430267, -0.000000000000000000 ) ) ;
#16924=DIRECTION ( 'NONE',  ( -0.000000000000000000, -0.000000000000000000, 1.000000000000000000 ) ) ;
#16926=AXIS2_PLACEMENT_3D ( 'NONE', #17567, #14851, #13302 ) ;
#16927=ORIENTED_EDGE ( 'NONE', *, *, #15735, .F. ) ;
#16928=ORIENTED_EDGE ( 'NONE', *, *, #15530, .F. ) ;
#16931=FACE_OUTER_BOUND ( 'NONE', #3527, .T. ) ;
#16932=CARTESIAN_POINT ( 'NONE',  ( 0.000000000000000000, 0.000000000000000000, 248.9926560891072143 ) ) ;
#16934=VECTOR ( 'NONE', #13259, 1000.000000000000114 ) ;
#16935=DIRECTION ( 'NONE',  ( -0.000000000000000000, -0.000000000000000000, 1.000000000000000000 ) ) ;
#16936=DIRECTION ( 'NONE',  ( -0.7660444431189725734, -0.6427876096865456912, 0.000000000000000000 ) ) ;
#16937=VECTOR ( 'NONE', #5270, 1000.000000000000114 ) ;
#16940=AXIS2_PLACEMENT_3D ( 'NONE', #3786, #10032, #16480 ) ;
#16941=LINE ( 'NONE', #12115, #12633 ) ;
#16943=CYLINDRICAL_SURFACE ( 'NONE', #993, 62.91752772691707207 ) ;
#16944=CARTESIAN_POINT ( 'NONE',  ( -45.84586732611835913, 36.66871011346426457, 110.7293897666001214 ) ) ;
#16945=LINE ( 'NONE', #18173, #16588 ) ;
#16946=CARTESIAN_POINT ( 'NONE',  ( 0.000000000000000000, 0.000000000000000000, 293.5832628385307999 ) ) ;
#16948=ORIENTED_EDGE ( 'NONE', *, *, #457, .F. ) ;
#16950=ORIENTED_EDGE ( 'NONE', *, *, #6295, .F. ) ;
#16952=AXIS2_PLACEMENT_3D ( 'NONE', #13373, #15215, #12036 ) ;
#16954=DIRECTION ( 'NONE',  ( 0.000000000000000000, 0.000000000000000000, -1.000000000000000000 ) ) ;
#16956=VERTEX_POINT ( 'NONE', #14727 ) ;
#16957=LINE ( 'NONE', #2946, #12941 ) ;
#16959=CARTESIAN_POINT ( 'NONE',  ( -32.61983739937760873, -51.24071425735591134, 293.5832628385307999 ) ) ;
#16961=VERTEX_POINT ( 'NONE', #7163 ) ;
#16963=LINE ( 'NONE', #10709, #3245 ) ;
#16966=DIRECTION ( 'NONE',  ( 1.000000000000000000, 0.000000000000000000, 0.000000000000000000 ) ) ;
#16967=VECTOR ( 'NONE', #17010, 1000.000000000000227 ) ;
#16969=ADVANCED_FACE ( 'NONE', ( #16276 ), #5620, .T. ) ;
#16970=CARTESIAN_POINT ( 'NONE',  ( 0.000000000000000000, 0.000000000000000000, 248.9926560891072143 ) ) ;
#16971=DIRECTION ( 'NONE',  ( 1.000000000000000000, 0.000000000000000000, 0.000000000000000000 ) ) ;
#16976=FACE_OUTER_BOUND ( 'NONE', #1014, .T. ) ;
#16977=ORIENTED_EDGE ( 'NONE', *, *, #3856, .F. ) ;
#16979=CARTESIAN_POINT ( 'NONE',  ( 0.000000000000000000, 0.000000000000000000, 293.5832628385307999 ) ) ;
#16981=ORIENTED_EDGE ( 'NONE', *, *, #5577, .T. ) ;
#16982=VECTOR ( 'NONE', #11545, 1000.000000000000114 ) ;
#16983=AXIS2_PLACEMENT_3D ( 'NONE', #6509, #13029, #19089 ) ;
#16984=EDGE_CURVE ( 'NONE', #15949, #10094, #13177, .T. ) ;
#16986=CARTESIAN_POINT ( 'NONE',  ( 0.000000000000000000, 0.000000000000000000, 248.9926560891072143 ) ) ;
#16989=DIRECTION ( 'NONE',  ( 0.000000000000000000, 0.000000000000000000, 1.000000000000000000 ) ) ;
#16992=DIRECTION ( 'NONE',  ( -0.9396926207859115365, 0.3420201433256602197, 0.000000000000000000 ) ) ;
#16993=CARTESIAN_POINT ( 'NONE',  ( 51.24071425735603214, -32.61983739937743110, 283.5832628385307999 ) ) ;
#16994=ORIENTED_EDGE ( 'NONE', *, *, #1880, .T. ) ;
#16997=CARTESIAN_POINT ( 'NONE',  ( -20.74471755083564162, 59.39925916207566559, 132.4711112102474146 ) ) ;
#17003=DIRECTION ( 'NONE',  ( -0.000000000000000000, -0.000000000000000000, 1.000000000000000000 ) ) ;
#17004=ORIENTED_EDGE ( 'NONE', *, *, #10582, .T. ) ;
#17008=EDGE_LOOP ( 'NONE', ( #15751, #13793, #1638, #8423 ) ) ;
#17009=ADVANCED_FACE ( 'NONE', ( #6033 ), #7549, .F. ) ;
#17010=DIRECTION ( 'NONE',  ( -0.8479630283625716469, 0.5300553768524345344, 0.000000000000000000 ) ) ;
#17011=PLANE ( 'NONE',  #6751 ) ;
#17012=ORIENTED_EDGE ( 'NONE', *, *, #5556, .T. ) ;
#17014=DIRECTION ( 'NONE',  ( -0.8660254037844397068, 0.4999999999999978906, 0.000000000000000000 ) ) ;
#17016=CARTESIAN_POINT ( 'NONE',  ( -2.240720816136042348, 5.281164089014786178, 293.5832628385307999 ) ) ;
#17018=CARTESIAN_POINT ( 'NONE',  ( 76.92888220842486646, -14.39940464655733976, 112.0427633081292385 ) ) ;
#17020=CARTESIAN_POINT ( 'NONE',  ( 0.000000000000000000, 0.000000000000000000, 283.5832628385307999 ) ) ;
#17022=ADVANCED_FACE ( 'NONE', ( #19928 ), #7252, .T. ) ;
#17027=ORIENTED_EDGE ( 'NONE', *, *, #13878, .T. ) ;
#17028=VECTOR ( 'NONE', #60, 1000.000000000000000 ) ;
#17030=VECTOR ( 'NONE', #40, 1000.000000000000114 ) ;
#17033=EDGE_CURVE ( 'NONE', #6781, #12002, #15432, .T. ) ;
#17034=VERTEX_POINT ( 'NONE', #8978 ) ;
#17036=VECTOR ( 'NONE', #15897, 1000.000000000000000 ) ;
#17040=CARTESIAN_POINT ( 'NONE',  ( -53.78543575132151489, -32.64570716507521553, 293.5832628385307999 ) ) ;
#17043=DIRECTION ( 'NONE',  ( 0.000000000000000000, 0.000000000000000000, -1.000000000000000000 ) ) ;
#17045=ORIENTED_EDGE ( 'NONE', *, *, #15013, .F. ) ;
#17047=DIRECTION ( 'NONE',  ( -0.7881095627315619634, -0.6155349844899687950, 0.000000000000000000 ) ) ;
#17049=DIRECTION ( 'NONE',  ( 0.000000000000000000, 0.000000000000000000, -1.000000000000000000 ) ) ;
#17052=FACE_OUTER_BOUND ( 'NONE', #17574, .T. ) ;
#17059=VECTOR ( 'NONE', #6691, 999.9999999999998863 ) ;
#17062=EDGE_CURVE ( 'NONE', #3790, #7238, #6133, .T. ) ;
#17066=ORIENTED_EDGE ( 'NONE', *, *, #2526, .T. ) ;
#17069=ORIENTED_EDGE ( 'NONE', *, *, #20144, .F. ) ;
#17072=DIRECTION ( 'NONE',  ( 0.3420201433256757073, -0.9396926207859057634, 0.000000000000000000 ) ) ;
#17077=ORIENTED_EDGE ( 'NONE', *, *, #17417, .F. ) ;
#17080=AXIS2_PLACEMENT_3D ( 'NONE', #5622, #10312, #2552 ) ;
#17081=ORIENTED_EDGE ( 'NONE', *, *, #2609, .T. ) ;
#17082=CARTESIAN_POINT ( 'NONE',  ( 57.61627707419550148, 19.23614321207255529, 283.5832628385307999 ) ) ;
#17083=EDGE_LOOP ( 'NONE', ( #3644, #19836, #4902, #15289 ) ) ;
#17084=EDGE_CURVE ( 'NONE', #6026, #1034, #15025, .T. ) ;
#17086=CARTESIAN_POINT ( 'NONE',  ( 0.000000000000000000, 0.000000000000000000, 293.5832628385307999 ) ) ;
#17087=VECTOR ( 'NONE', #10537, 1000.000000000000000 ) ;
#17090=CARTESIAN_POINT ( 'NONE',  ( 0.000000000000000000, 0.000000000000000000, 283.5832628385307999 ) ) ;
#17091=DIRECTION ( 'NONE',  ( -0.000000000000000000, -0.000000000000000000, 1.000000000000000000 ) ) ;
#17094=EDGE_CURVE ( 'NONE', #1901, #6781, #12146, .T. ) ;
#17096=DIRECTION ( 'NONE',  ( -0.000000000000000000, -0.000000000000000000, 1.000000000000000000 ) ) ;
#17097=CARTESIAN_POINT ( 'NONE',  ( 25.99419088092191643, -73.82206860051539365, 111.4180192758973362 ) ) ;
#17101=CARTESIAN_POINT ( 'NONE',  ( 40.28046525994349736, 45.46865632508086463, 283.5832628385307999 ) ) ;
#17103=ORIENTED_EDGE ( 'NONE', *, *, #19389, .F. ) ;
#17108=ORIENTED_EDGE ( 'NONE', *, *, #16886, .T. ) ;
#17109=EDGE_CURVE ( 'NONE', #12789, #13695, #15219, .T. ) ;
#17112=DIRECTION ( 'NONE',  ( 0.000000000000000000, 0.000000000000000000, -1.000000000000000000 ) ) ;
#17116=DIRECTION ( 'NONE',  ( -0.6155349844899689060, 0.7881095627315620744, 0.000000000000000000 ) ) ;
#17120=DIRECTION ( 'NONE',  ( -0.000000000000000000, -0.000000000000000000, 1.000000000000000000 ) ) ;
#17121=CARTESIAN_POINT ( 'NONE',  ( 11.00103590902871353, 57.65577537092163851, 248.9926560891072143 ) ) ;
#17123=EDGE_CURVE ( 'NONE', #2635, #7392, #15120, .T. ) ;
#17127=LINE ( 'NONE', #14051, #17030 ) ;
#17130=ORIENTED_EDGE ( 'NONE', *, *, #11590, .F. ) ;
#17133=VECTOR ( 'NONE', #4764, 1000.000000000000114 ) ;
#17136=EDGE_CURVE ( 'NONE', #9872, #9804, #5932, .T. ) ;
#17138=ORIENTED_EDGE ( 'NONE', *, *, #15385, .F. ) ;
#17139=VECTOR ( 'NONE', #2473, 1000.000000000000000 ) ;
#17141=CARTESIAN_POINT ( 'NONE',  ( 28.94886449118905247, -53.40063514825087054, 293.5832628385307999 ) ) ;
#17143=DIRECTION ( 'NONE',  ( -0.3088643371590125697, 0.9511061040868803440, 0.000000000000000000 ) ) ;
#17145=CARTESIAN_POINT ( 'NONE',  ( 59.51724408343574879, -12.14957802882732452, 283.5832628385307999 ) ) ;
#17148=DIRECTION ( 'NONE',  ( 1.000000000000000000, 0.000000000000000000, 0.000000000000000000 ) ) ;
#17153=LINE ( 'NONE', #1392, #2216 ) ;
#17154=ADVANCED_FACE ( 'NONE', ( #1826 ), #6239, .F. ) ;
#17156=EDGE_CURVE ( 'NONE', #11965, #20114, #6641, .T. ) ;
#17158=VECTOR ( 'NONE', #4697, 1000.000000000000000 ) ;
#17159=LINE ( 'NONE', #4779, #854 ) ;
#17162=ORIENTED_EDGE ( 'NONE', *, *, #9627, .T. ) ;
#17166=ORIENTED_EDGE ( 'NONE', *, *, #18630, .F. ) ;
#17167=PLANE ( 'NONE',  #8375 ) ;
#17169=CARTESIAN_POINT ( 'NONE',  ( 51.36153797460909232, -59.06449708980179736, 132.4711112102474146 ) ) ;
#17170=CARTESIAN_POINT ( 'NONE',  ( 60.72073886220397299, -1.629865514042299512, 293.5832628385307999 ) ) ;
#17172=LINE ( 'NONE', #280, #14303 ) ;
#17174=CARTESIAN_POINT ( 'NONE',  ( 0.000000000000000000, 0.000000000000000000, 248.9926560891072143 ) ) ;
#17176=EDGE_LOOP ( 'NONE', ( #16574, #11139, #14403, #1530 ) ) ;
#17179=FACE_OUTER_BOUND ( 'NONE', #8775, .T. ) ;
#17181=EDGE_CURVE ( 'NONE', #5705, #5779, #12766, .T. ) ;
#17182=LINE ( 'NONE', #3164, #11592 ) ;
#17184=LINE ( 'NONE', #12455, #8816 ) ;
#17185=CARTESIAN_POINT ( 'NONE',  ( -68.18670162478831287, -38.41834839689355618, 132.4711112102474146 ) ) ;
#17186=EDGE_CURVE ( 'NONE', #675, #244, #11348, .T. ) ;
#17189=ORIENTED_EDGE ( 'NONE', *, *, #9175, .T. ) ;
#17190=APPLICATION_CONTEXT ( 'automotive_design' ) ;
#17195=CARTESIAN_POINT ( 'NONE',  ( 0.000000000000000000, 0.000000000000000000, 248.9926560891072143 ) ) ;
#17196=DIRECTION ( 'NONE',  ( -0.000000000000000000, -0.000000000000000000, 1.000000000000000000 ) ) ;
#17198=CARTESIAN_POINT ( 'NONE',  ( 56.50329132715945235, -22.30005961346246579, 283.5832628385307999 ) ) ;
#17199=PLANE ( 'NONE',  #4785 ) ;
#17201=CARTESIAN_POINT ( 'NONE',  ( 48.17959877923549072, 36.99514631729036296, 293.5832628385307999 ) ) ;
#17204=CARTESIAN_POINT ( 'NONE',  ( -12.28122767885803945, 61.70726652483829611, 132.4711112102474146 ) ) ;
#17207=CARTESIAN_POINT ( 'NONE',  ( -73.82206860051549313, -25.99419088092168195, 132.4711112102474146 ) ) ;
#17211=LINE ( 'NONE', #9111, #15614 ) ;
#17214=ORIENTED_EDGE ( 'NONE', *, *, #18673, .T. ) ;
#17216=ORIENTED_EDGE ( 'NONE', *, *, #19362, .T. ) ;
#17221=ORIENTED_EDGE ( 'NONE', *, *, #6366, .F. ) ;
#17223=CARTESIAN_POINT ( 'NONE',  ( 37.78325588002174840, -47.56406379474564972, 293.5832628385307999 ) ) ;
#17225=AXIS2_PLACEMENT_3D ( 'NONE', #487, #7951, #9692 ) ;
#17226=AXIS2_PLACEMENT_3D ( 'NONE', #11665, #5538, #14644 ) ;
#17232=DIRECTION ( 'NONE',  ( 0.1736481776669306920, -0.9848077530122080203, 0.000000000000000000 ) ) ;
#17233=DIRECTION ( 'NONE',  ( 1.000000000000000000, 0.000000000000000000, 0.000000000000000000 ) ) ;
#17236=EDGE_LOOP ( 'NONE', ( #18414, #5575, #17429, #15884 ) ) ;
#17237=DIRECTION ( 'NONE',  ( 1.000000000000000000, 0.000000000000000000, 0.000000000000000000 ) ) ;
#17238=ORIENTED_EDGE ( 'NONE', *, *, #9300, .T. ) ;
#17240=AXIS2_PLACEMENT_3D ( 'NONE', #9502, #1720, #3462 ) ;
#17241=EDGE_CURVE ( 'NONE', #2612, #17735, #15643, .T. ) ;
#17245=FACE_OUTER_BOUND ( 'NONE', #5860, .T. ) ;
#17249=CARTESIAN_POINT ( 'NONE',  ( 0.000000000000000000, 0.000000000000000000, 283.5832628385307999 ) ) ;
#17251=DIRECTION ( 'NONE',  ( 1.000000000000000000, 0.000000000000000000, -0.000000000000000000 ) ) ;
#17252=DIRECTION ( 'NONE',  ( 1.000000000000000000, 0.000000000000000000, 0.000000000000000000 ) ) ;
#17256=VERTEX_POINT ( 'NONE', #18822 ) ;
#17260=ORIENTED_EDGE ( 'NONE', *, *, #18462, .T. ) ;
#17262=ORIENTED_EDGE ( 'NONE', *, *, #17519, .F. ) ;
#17263=EDGE_LOOP ( 'NONE', ( #10415, #2314, #9048 ) ) ;
#17264=LINE ( 'NONE', #14188, #19691 ) ;
#17268=EDGE_CURVE ( 'NONE', #12685, #5478, #6791, .T. ) ;
#17269=AXIS2_PLACEMENT_3D ( 'NONE', #18683, #12828, #11089 ) ;
#17271=DIRECTION ( 'NONE',  ( 0.8479630283625716469, -0.5300553768524345344, 0.000000000000000000 ) ) ;
#17274=DIRECTION ( 'NONE',  ( 0.000000000000000000, 0.000000000000000000, -1.000000000000000000 ) ) ;
#17278=PLANE ( 'NONE',  #1280 ) ;
#17279=VERTEX_POINT ( 'NONE', #11127 ) ;
#17280=DIRECTION ( 'NONE',  ( 0.3747554100459959958, 0.9271237148521535021, 0.000000000000000000 ) ) ;
#17281=FACE_OUTER_BOUND ( 'NONE', #11753, .T. ) ;
#17282=CARTESIAN_POINT ( 'NONE',  ( 57.92709869106709419, 18.28567271940532990, 283.5832628385307999 ) ) ;
#17284=VECTOR ( 'NONE', #12188, 1000.000000000000000 ) ;
#17291=VECTOR ( 'NONE', #2228, 1000.000000000000000 ) ;
#17292=LINE ( 'NONE', #3367, #1755 ) ;
#17293=EDGE_LOOP ( 'NONE', ( #9716, #5855, #17391, #4418 ) ) ;
#17296=ADVANCED_FACE ( 'NONE', ( #9697 ), #15946, .T. ) ;
#17302=AXIS2_PLACEMENT_3D ( 'NONE', #2984, #13813, #5849 ) ;
#17306=VECTOR ( 'NONE', #6233, 1000.000000000000000 ) ;
#17311=ORIENTED_EDGE ( 'NONE', *, *, #19387, .T. ) ;
#17314=PLANE ( 'NONE',  #4477 ) ;
#17317=ORIENTED_EDGE ( 'NONE', *, *, #14655, .T. ) ;
#17318=CYLINDRICAL_SURFACE ( 'NONE', #6499, 62.91752772691707207 ) ;
#17321=VECTOR ( 'NONE', #18018, 1000.000000000000000 ) ;
#17322=AXIS2_PLACEMENT_3D ( 'NONE', #2925, #19995, #10680 ) ;
#17326=ORIENTED_EDGE ( 'NONE', *, *, #13848, .T. ) ;
#17331=LINE ( 'NONE', #14041, #3044 ) ;
#17332=FACE_OUTER_BOUND ( 'NONE', #1118, .T. ) ;
#17336=CARTESIAN_POINT ( 'NONE',  ( 73.25972925305627825, -27.53920554013664912, 132.4711112102474146 ) ) ;
#17338=DIRECTION ( 'NONE',  ( -0.8660254037844363761, -0.5000000000000039968, 0.000000000000000000 ) ) ;
#17345=AXIS2_PLACEMENT_3D ( 'NONE', #10508, #16764, #4383 ) ;
#17351=EDGE_CURVE ( 'NONE', #3741, #10316, #8560, .T. ) ;
#17352=DIRECTION ( 'NONE',  ( 0.5000000000000101030, -0.8660254037844328234, 0.000000000000000000 ) ) ;
#17353=DIRECTION ( 'NONE',  ( 1.000000000000000000, 0.000000000000000000, 0.000000000000000000 ) ) ;
#17354=CARTESIAN_POINT ( 'NONE',  ( -26.55444175050983091, 16.92388544840482112, 248.9926560891072143 ) ) ;
#17356=CIRCLE ( 'NONE', #8523, 60.74260934110282051 ) ;
#17357=DIRECTION ( 'NONE',  ( 1.000000000000000000, 0.000000000000000000, 0.000000000000000000 ) ) ;
#17360=AXIS2_PLACEMENT_3D ( 'NONE', #5080, #6516, #19193 ) ;
#17361=CARTESIAN_POINT ( 'NONE',  ( 0.000000000000000000, 0.000000000000000000, 283.5832628385307999 ) ) ;
#17364=LINE ( 'NONE', #3439, #14320 ) ;
#17366=ORIENTED_EDGE ( 'NONE', *, *, #13385, .F. ) ;
#17367=EDGE_LOOP ( 'NONE', ( #4943, #7067, #12436, #21 ) ) ;
#17368=ORIENTED_EDGE ( 'NONE', *, *, #1855, .T. ) ;
#17372=DIRECTION ( 'NONE',  ( 1.000000000000000000, 0.000000000000000000, 0.000000000000000000 ) ) ;
#17373=CIRCLE ( 'NONE', #5583, 62.91752772691707207 ) ;
#17378=ORIENTED_EDGE ( 'NONE', *, *, #4273, .T. ) ;
#17380=DIRECTION ( 'NONE',  ( 0.8660254037844380415, 0.5000000000000009992, 0.000000000000000000 ) ) ;
#17381=VERTEX_POINT ( 'NONE', #787 ) ;
#17384=CARTESIAN_POINT ( 'NONE',  ( -59.58067424803613221, 20.21777810286735999, 293.5832628385307999 ) ) ;
#17385=DIRECTION ( 'NONE',  ( 0.000000000000000000, -0.000000000000000000, 1.000000000000000000 ) ) ;
#17391=ORIENTED_EDGE ( 'NONE', *, *, #18225, .F. ) ;
#17393=DIRECTION ( 'NONE',  ( 0.000000000000000000, 0.000000000000000000, 1.000000000000000000 ) ) ;
#17399=CARTESIAN_POINT ( 'NONE',  ( 5.729042578294149202, 0.2993243175132214717, 293.5832628385307999 ) ) ;
#17401=DIRECTION ( 'NONE',  ( 0.6427876096865300370, 0.7660444431189858960, 0.000000000000000000 ) ) ;
#17402=ORIENTED_EDGE ( 'NONE', *, *, #7147, .F. ) ;
#17404=DIRECTION ( 'NONE',  ( 0.9848077530122080203, 0.1736481776669306920, 0.000000000000000000 ) ) ;
#17406=VECTOR ( 'NONE', #6739, 1000.000000000000000 ) ;
#17407=VECTOR ( 'NONE', #4976, 1000.000000000000000 ) ;
#17408=CARTESIAN_POINT ( 'NONE',  ( 4.811834253409037032, 3.123743752084113812, 283.5832628385307999 ) ) ;
#17409=PLANE ( 'NONE',  #6371 ) ;
#17411=PLANE ( 'NONE',  #7918 ) ;
#17412=DIRECTION ( 'NONE',  ( -0.9396926207859058744, -0.3420201433256757628, 0.000000000000000000 ) ) ;
#17417=EDGE_CURVE ( 'NONE', #9731, #9274, #4507, .T. ) ;
#17426=SHAPE_DEFINITION_REPRESENTATION ( #5092, #13949 ) ;
#17427=AXIS2_PLACEMENT_3D ( 'NONE', #13405, #16695, #3913 ) ;
#17428=VECTOR ( 'NONE', #7081, 1000.000000000000000 ) ;
#17429=ORIENTED_EDGE ( 'NONE', *, *, #17504, .T. ) ;
#17436=DIRECTION ( 'NONE',  ( 1.000000000000000000, 0.000000000000000000, 0.000000000000000000 ) ) ;
#17439=CARTESIAN_POINT ( 'NONE',  ( 41.06890862491472660, 47.66508197439486594, 132.4711112102474146 ) ) ;
#17441=AXIS2_PLACEMENT_3D ( 'NONE', #1527, #8883, #1429 ) ;
#17442=VECTOR ( 'NONE', #6723, 1000.000000000000000 ) ;
#17444=CYLINDRICAL_SURFACE ( 'NONE', #19326, 62.91752772691707207 ) ;
#17447=ORIENTED_EDGE ( 'NONE', *, *, #6051, .T. ) ;
#17448=CARTESIAN_POINT ( 'NONE',  ( 0.000000000000000000, 0.000000000000000000, 248.9926560891072143 ) ) ;
#17449=EDGE_CURVE ( 'NONE', #10313, #2962, #16945, .T. ) ;
#17450=VERTEX_POINT ( 'NONE', #15406 ) ;
#17455=DIRECTION ( 'NONE',  ( 1.000000000000000000, 0.000000000000000000, 0.000000000000000000 ) ) ;
#17456=CARTESIAN_POINT ( 'NONE',  ( -48.17797692984161984, -36.99387960884178028, 293.5832628385307999 ) ) ;
#17457=AXIS2_PLACEMENT_3D ( 'NONE', #14552, #6783, #19267 ) ;
#17459=CARTESIAN_POINT ( 'NONE',  ( -51.24071425735602503, 32.61983739937743820, 283.5832628385307999 ) ) ;
#17461=CARTESIAN_POINT ( 'NONE',  ( 60.74260934110282051, 0.000000000000000000, 293.5832628385307999 ) ) ;
#17462=AXIS2_PLACEMENT_3D ( 'NONE', #7436, #10398, #13880 ) ;
#17467=LINE ( 'NONE', #3542, #11645 ) ;
#17472=ORIENTED_EDGE ( 'NONE', *, *, #9863, .T. ) ;
#17473=PLANE ( 'NONE',  #3703 ) ;
#17475=ORIENTED_EDGE ( 'NONE', *, *, #844, .T. ) ;
#17478=DIRECTION ( 'NONE',  ( 0.4693298356057531984, -0.8830229359480288309, 0.000000000000000000 ) ) ;
#17479=LINE ( 'NONE', #18812, #19519 ) ;
#17485=DIRECTION ( 'NONE',  ( 1.000000000000000000, 0.000000000000000000, 0.000000000000000000 ) ) ;
#17488=CARTESIAN_POINT ( 'NONE',  ( 1.678175111358115590, 5.485913980968027737, 283.5832628385307999 ) ) ;
#17493=CARTESIAN_POINT ( 'NONE',  ( 0.000000000000000000, 0.000000000000000000, 293.5832628385307999 ) ) ;
#17495=ORIENTED_EDGE ( 'NONE', *, *, #18046, .F. ) ;
#17497=AXIS2_PLACEMENT_3D ( 'NONE', #13473, #16371, #11933 ) ;
#17498=VERTEX_POINT ( 'NONE', #5799 ) ;
#17500=PLANE ( 'NONE',  #6496 ) ;
#17501=EDGE_CURVE ( 'NONE', #14032, #5816, #4054, .T. ) ;
#17503=ORIENTED_EDGE ( 'NONE', *, *, #5068, .F. ) ;
#17504=EDGE_CURVE ( 'NONE', #3145, #1943, #12018, .T. ) ;
#17507=EDGE_CURVE ( 'NONE', #10402, #4473, #10384, .T. ) ;
#17509=CYLINDRICAL_SURFACE ( 'NONE', #2911, 62.91752772691707207 ) ;
#17514=CARTESIAN_POINT ( 'NONE',  ( 0.000000000000000000, 0.000000000000000000, 283.5832628385307999 ) ) ;
#17518=EDGE_LOOP ( 'NONE', ( #16717, #10786, #3750, #8320 ) ) ;
#17519=EDGE_CURVE ( 'NONE', #5404, #14388, #15300, .T. ) ;
#17520=FACE_OUTER_BOUND ( 'NONE', #18572, .T. ) ;
#17521=LINE ( 'NONE', #11366, #9899 ) ;
#17522=VERTEX_POINT ( 'NONE', #16838 ) ;
#17523=CIRCLE ( 'NONE', #14570, 60.74260934110282051 ) ;
#17528=VECTOR ( 'NONE', #7847, 1000.000000000000000 ) ;
#17529=ORIENTED_EDGE ( 'NONE', *, *, #8017, .T. ) ;
#17530=CARTESIAN_POINT ( 'NONE',  ( 57.94128254008182921, 9.381844291199925578, 132.4711112102474146 ) ) ;
#17531=LINE ( 'NONE', #15987, #7404 ) ;
#17532=ORIENTED_EDGE ( 'NONE', *, *, #19270, .F. ) ;
#17538=VECTOR ( 'NONE', #14719, 1000.000000000000000 ) ;
#17541=CARTESIAN_POINT ( 'NONE',  ( -2.629250726500700353, -60.68567895461850981, 283.5832628385307999 ) ) ;
#17543=CYLINDRICAL_SURFACE ( 'NONE', #18016, 62.91752772691707207 ) ;
#17545=ORIENTED_EDGE ( 'NONE', *, *, #7274, .T. ) ;
#17546=AXIS2_PLACEMENT_3D ( 'NONE', #13709, #6160, #1130 ) ;
#17548=CARTESIAN_POINT ( 'NONE',  ( -56.12662799072088404, 23.22641211976270625, 283.5832628385307999 ) ) ;
#17551=ORIENTED_EDGE ( 'NONE', *, *, #19603, .T. ) ;
#17552=CIRCLE ( 'NONE', #4136, 60.74260934110282051 ) ;
#17553=EDGE_LOOP ( 'NONE', ( #18771, #449, #16650, #15849 ) ) ;
#17554=EDGE_CURVE ( 'NONE', #7714, #6701, #17364, .T. ) ;
#17555=EDGE_CURVE ( 'NONE', #16780, #9274, #20210, .T. ) ;
#17556=DIRECTION ( 'NONE',  ( -0.000000000000000000, -0.000000000000000000, 1.000000000000000000 ) ) ;
#17560=EDGE_CURVE ( 'NONE', #3720, #8668, #18585, .T. ) ;
#17561=CARTESIAN_POINT ( 'NONE',  ( 47.56406379474552182, 37.78325588002191893, 293.5832628385307999 ) ) ;
#17562=DIRECTION ( 'NONE',  ( 0.9271237148521548344, -0.3747554100459928317, 0.000000000000000000 ) ) ;
#17565=FACE_OUTER_BOUND ( 'NONE', #20110, .T. ) ;
#17566=EDGE_LOOP ( 'NONE', ( #14616, #2415, #942 ) ) ;
#17567=CARTESIAN_POINT ( 'NONE',  ( 11.00103590902871353, 57.65577537092163851, 112.0427633081292953 ) ) ;
#17572=VECTOR ( 'NONE', #7009, 1000.000000000000227 ) ;
#17573=ORIENTED_EDGE ( 'NONE', *, *, #168, .F. ) ;
#17574=EDGE_LOOP ( 'NONE', ( #19226, #1053, #18965, #6445 ) ) ;
#17580=LINE ( 'NONE', #14299, #11032 ) ;
#17581=VERTEX_POINT ( 'NONE', #3038 ) ;
#17583=CARTESIAN_POINT ( 'NONE',  ( -22.30005961346265408, -56.50329132715937419, 283.5832628385307999 ) ) ;
#17584=CIRCLE ( 'NONE', #7110, 60.74260934110282051 ) ;
#17588=DIRECTION ( 'NONE',  ( -0.000000000000000000, -0.000000000000000000, 1.000000000000000000 ) ) ;
#17589=DIRECTION ( 'NONE',  ( 0.000000000000000000, 0.000000000000000000, 1.000000000000000000 ) ) ;
#17590=CARTESIAN_POINT ( 'NONE',  ( 0.8220851292435327196, 78.26059000578311498, 132.4711112102474146 ) ) ;
#17593=ORIENTED_EDGE ( 'NONE', *, *, #12193, .T. ) ;
#17594=CARTESIAN_POINT ( 'NONE',  ( 51.36153797460909232, -59.06449708980179025, 110.7293897666001214 ) ) ;
#17598=AXIS2_PLACEMENT_3D ( 'NONE', #16793, #18536, #2787 ) ;
#17603=CARTESIAN_POINT ( 'NONE',  ( 59.51724408343574879, -12.14957802882732452, 293.5832628385307999 ) ) ;
#17604=ADVANCED_FACE ( 'NONE', ( #8034 ), #9372, .F. ) ;
#17605=CARTESIAN_POINT ( 'NONE',  ( 40.27908801169993325, 45.46712722958823605, 283.5832628385307999 ) ) ;
#17606=CARTESIAN_POINT ( 'NONE',  ( 78.26059000578312919, -0.8220851292427129309, 132.4711112102474146 ) ) ;
#17608=CIRCLE ( 'NONE', #8762, 62.91752772691707207 ) ;
#17609=AXIS2_PLACEMENT_3D ( 'NONE', #13467, #8874, #7155 ) ;
#17610=LINE ( 'NONE', #16173, #1993 ) ;
#17611=DIRECTION ( 'NONE',  ( -0.000000000000000000, -0.000000000000000000, 1.000000000000000000 ) ) ;
#17613=ORIENTED_EDGE ( 'NONE', *, *, #6227, .T. ) ;
#17615=DIRECTION ( 'NONE',  ( 1.000000000000000000, 0.000000000000000000, 0.000000000000000000 ) ) ;
#17616=DIRECTION ( 'NONE',  ( -0.4693298356057531429, 0.8830229359480288309, 0.000000000000000000 ) ) ;
#17620=DIRECTION ( 'NONE',  ( -0.000000000000000000, -0.000000000000000000, 1.000000000000000000 ) ) ;
#17624=EDGE_CURVE ( 'NONE', #14438, #17628, #19656, .T. ) ;
#17627=VECTOR ( 'NONE', #878, 1000.000000000000000 ) ;
#17628=VERTEX_POINT ( 'NONE', #17940 ) ;
#17633=ORIENTED_EDGE ( 'NONE', *, *, #17919, .F. ) ;
#17634=CARTESIAN_POINT ( 'NONE',  ( -36.66871011346412246, -45.84586732611848703, 132.4711112102474146 ) ) ;
#17635=DIRECTION ( 'NONE',  ( -0.7660444431189749048, -0.6427876096865430267, 0.000000000000000000 ) ) ;
#17637=ADVANCED_FACE ( 'NONE', ( #6988 ), #10058, .T. ) ;
#17641=DIRECTION ( 'NONE',  ( 0.9396926207859127578, -0.3420201433256568335, 0.000000000000000000 ) ) ;
#17642=AXIS2_PLACEMENT_3D ( 'NONE', #5277, #11410, #5079 ) ;
#17644=AXIS2_PLACEMENT_3D ( 'NONE', #13753, #6207, #54 ) ;
#17645=ORIENTED_EDGE ( 'NONE', *, *, #17084, .F. ) ;
#17646=ADVANCED_FACE ( 'NONE', ( #1031 ), #11310, .F. ) ;
#17653=LINE ( 'NONE', #10160, #3717 ) ;
#17656=CARTESIAN_POINT ( 'NONE',  ( 0.000000000000000000, 0.000000000000000000, 283.5832628385307999 ) ) ;
#17661=CARTESIAN_POINT ( 'NONE',  ( 73.25972925305627825, -27.53920554013664912, 111.4180192758974499 ) ) ;
#17662=CARTESIAN_POINT ( 'NONE',  ( 1.678175111358173099, 5.485913980968232018, 293.5832628385307999 ) ) ;
#17664=DIRECTION ( 'NONE',  ( -0.000000000000000000, -0.000000000000000000, 1.000000000000000000 ) ) ;
#17665=ORIENTED_EDGE ( 'NONE', *, *, #14125, .F. ) ;
#17669=DIRECTION ( 'NONE',  ( 1.000000000000000000, 0.000000000000000000, -0.000000000000000000 ) ) ;
#17670=ORIENTED_EDGE ( 'NONE', *, *, #12070, .F. ) ;
#17672=ORIENTED_EDGE ( 'NONE', *, *, #16512, .T. ) ;
#17673=ORIENTED_EDGE ( 'NONE', *, *, #12912, .T. ) ;
#17674=ORIENTED_EDGE ( 'NONE', *, *, #1523, .F. ) ;
#17677=ORIENTED_EDGE ( 'NONE', *, *, #7361, .T. ) ;
#17680=DIRECTION ( 'NONE',  ( 1.000000000000000000, 0.000000000000000000, 0.000000000000000000 ) ) ;
#17682=EDGE_LOOP ( 'NONE', ( #19020, #18507, #6219, #14083 ) ) ;
#17684=CARTESIAN_POINT ( 'NONE',  ( 59.39925916207545242, 20.74471755083624203, 293.5832628385307999 ) ) ;
#17685=CARTESIAN_POINT ( 'NONE',  ( 5.281164089014835028, 2.240720816136097859, 293.5832628385307999 ) ) ;
#17688=DIRECTION ( 'NONE',  ( 0.000000000000000000, -0.000000000000000000, 1.000000000000000000 ) ) ;
#17689=DIRECTION ( 'NONE',  ( -0.6427876096865405842, 0.7660444431189771253, 0.000000000000000000 ) ) ;
#17690=DIRECTION ( 'NONE',  ( 0.6427876096865481337, -0.7660444431189707970, 0.000000000000000000 ) ) ;
#17692=DIRECTION ( 'NONE',  ( 0.000000000000000000, 0.000000000000000000, -1.000000000000000000 ) ) ;
#17698=ORIENTED_EDGE ( 'NONE', *, *, #16379, .F. ) ;
#17701=CARTESIAN_POINT ( 'NONE',  ( -12.78021302872797449, 77.21438937758516374, 132.4711112102474146 ) ) ;
#17702=VERTEX_POINT ( 'NONE', #2382 ) ;
#17703=PLANE ( 'NONE',  #12351 ) ;
#17704=CARTESIAN_POINT ( 'NONE',  ( -27.53920554013687649, -73.25972925305620720, 111.4180192758973931 ) ) ;
#17706=CARTESIAN_POINT ( 'NONE',  ( 0.000000000000000000, 0.000000000000000000, 132.4711112102474146 ) ) ;
#17709=CARTESIAN_POINT ( 'NONE',  ( 62.91215678473958661, -0.8220851292428736912, 248.9926560891072143 ) ) ;
#17710=DIRECTION ( 'NONE',  ( 0.1736481776669374366, -0.9848077530122066880, 0.000000000000000000 ) ) ;
#17711=CARTESIAN_POINT ( 'NONE',  ( -49.24833719034228352, -60.83768308848360817, 110.7293897666001214 ) ) ;
#17715=CARTESIAN_POINT ( 'NONE',  ( 53.87178215532755132, 28.06680738835045119, 293.5832628385307999 ) ) ;
#17718=CARTESIAN_POINT ( 'NONE',  ( 0.000000000000000000, 0.000000000000000000, 132.4711112102474146 ) ) ;
#17723=ORIENTED_EDGE ( 'NONE', *, *, #2756, .T. ) ;
#17726=AXIS2_PLACEMENT_3D ( 'NONE', #7808, #6389, #1875 ) ;
#17727=LINE ( 'NONE', #3605, #6658 ) ;
#17730=ORIENTED_EDGE ( 'NONE', *, *, #18888, .F. ) ;
#17733=DIRECTION ( 'NONE',  ( 0.000000000000000000, 0.000000000000000000, 1.000000000000000000 ) ) ;
#17735=VERTEX_POINT ( 'NONE', #835 ) ;
#17736=CARTESIAN_POINT ( 'NONE',  ( 12.23146955673593972, 77.31114765718498916, 248.9926560891072143 ) ) ;
#17740=VERTEX_POINT ( 'NONE', #10244 ) ;
#17741=VECTOR ( 'NONE', #7084, 999.9999999999998863 ) ;
#17742=ORIENTED_EDGE ( 'NONE', *, *, #4132, .T. ) ;
#17747=VECTOR ( 'NONE', #2885, 1000.000000000000000 ) ;
#17748=CARTESIAN_POINT ( 'NONE',  ( -60.47951622432784546, -49.67518383744813804, 248.9926560891072143 ) ) ;
#17750=EDGE_CURVE ( 'NONE', #17450, #3588, #15280, .T. ) ;
#17753=CARTESIAN_POINT ( 'NONE',  ( 48.72193424476451185, 39.80940113486035159, 132.4711112102474146 ) ) ;
#17754=CARTESIAN_POINT ( 'NONE',  ( 55.62246070845780110, -18.77710619359098132, 132.4711112102474146 ) ) ;
#17755=DIRECTION ( 'NONE',  ( -0.000000000000000000, -0.000000000000000000, 1.000000000000000000 ) ) ;
#17757=VECTOR ( 'NONE', #20116, 1000.000000000000000 ) ;
#17759=LINE ( 'NONE', #5082, #3526 ) ;
#17760=ORIENTED_EDGE ( 'NONE', *, *, #5846, .T. ) ;
#17762=ORIENTED_EDGE ( 'NONE', *, *, #2613, .T. ) ;
#17763=EDGE_CURVE ( 'NONE', #7735, #2759, #18, .T. ) ;
#17765=VECTOR ( 'NONE', #16768, 1000.000000000000000 ) ;
#17766=ORIENTED_EDGE ( 'NONE', *, *, #4993, .T. ) ;
#17767=ORIENTED_EDGE ( 'NONE', *, *, #3533, .T. ) ;
#17768=ORIENTED_EDGE ( 'NONE', *, *, #10493, .F. ) ;
#17769=CIRCLE ( 'NONE', #7958, 79.75827554147308263 ) ;
#17771=LINE ( 'NONE', #8549, #16154 ) ;
#17774=VERTEX_POINT ( 'NONE', #13714 ) ;
#17775=ADVANCED_FACE ( 'NONE', ( #5956 ), #7475, .F. ) ;
#17776=CARTESIAN_POINT ( 'NONE',  ( 36.99514631729018532, -48.17959877923561862, 293.5832628385307999 ) ) ;
#17778=EDGE_CURVE ( 'NONE', #10931, #12690, #1449, .T. ) ;
#17780=VERTEX_POINT ( 'NONE', #6271 ) ;
#17782=CARTESIAN_POINT ( 'NONE',  ( -30.09424155357359254, 27.05260723904714837, 248.9926560891072143 ) ) ;
#17786=FACE_OUTER_BOUND ( 'NONE', #9026, .T. ) ;
#17788=ORIENTED_EDGE ( 'NONE', *, *, #15036, .T. ) ;
#17791=VECTOR ( 'NONE', #15393, 1000.000000000000000 ) ;
#17794=DIRECTION ( 'NONE',  ( 0.8660254037844363761, 0.5000000000000039968, 0.000000000000000000 ) ) ;
#17796=DIRECTION ( 'NONE',  ( -0.000000000000000000, -0.000000000000000000, 1.000000000000000000 ) ) ;
#17798=ADVANCED_FACE ( 'NONE', ( #18331 ), #12480, .F. ) ;
#17799=EDGE_CURVE ( 'NONE', #10010, #20213, #4621, .T. ) ;
#17800=VECTOR ( 'NONE', #6358, 1000.000000000000000 ) ;
#17802=CARTESIAN_POINT ( 'NONE',  ( 0.000000000000000000, 0.000000000000000000, 293.5832628385307999 ) ) ;
#17804=DIRECTION ( 'NONE',  ( -0.9781142164131917394, 0.2080686897406911207, 0.000000000000000000 ) ) ;
#17805=CARTESIAN_POINT ( 'NONE',  ( 20.74471755083603952, -59.39925916207552348, 293.5832628385307999 ) ) ;
#17807=LINE ( 'NONE', #14822, #2641 ) ;
#17808=DIRECTION ( 'NONE',  ( -0.8830229359480288309, -0.4693298356057531984, 0.000000000000000000 ) ) ;
#17809=ORIENTED_EDGE ( 'NONE', *, *, #7993, .F. ) ;
#17812=CARTESIAN_POINT ( 'NONE',  ( -38.41834839689332171, 68.18670162478844077, 132.4711112102474146 ) ) ;
#17816=DIRECTION ( 'NONE',  ( 1.000000000000000000, 0.000000000000000000, 0.000000000000000000 ) ) ;
#17817=CARTESIAN_POINT ( 'NONE',  ( -5.590028426173819120, -1.289614712049182321, 293.5832628385307999 ) ) ;
#17821=ORIENTED_EDGE ( 'NONE', *, *, #2128, .F. ) ;
#17822=DIRECTION ( 'NONE',  ( -0.9848077530122062440, -0.1736481776669404620, 0.000000000000000000 ) ) ;
#17824=ORIENTED_EDGE ( 'NONE', *, *, #7361, .F. ) ;
#17826=CARTESIAN_POINT ( 'NONE',  ( 18.92519137117231054, 56.02932139001904233, 248.9926560891072143 ) ) ;
#17829=ORIENTED_EDGE ( 'NONE', *, *, #10467, .T. ) ;
#17831=DIRECTION ( 'NONE',  ( -0.5000000000000009992, 0.8660254037844380415, 0.000000000000000000 ) ) ;
#17833=LINE ( 'NONE', #736, #16026 ) ;
#17834=DIRECTION ( 'NONE',  ( -0.000000000000000000, -0.000000000000000000, 1.000000000000000000 ) ) ;
#17837=VERTEX_POINT ( 'NONE', #12067 ) ;
#17838=DIRECTION ( 'NONE',  ( 0.6427876096865405842, -0.7660444431189771253, -0.000000000000000000 ) ) ;
#17839=MECHANICAL_DESIGN_GEOMETRIC_PRESENTATION_REPRESENTATION('',(#10625),#837);
#17845=DIRECTION ( 'NONE',  ( 0.7430374143461878633, -0.6692498792541777819, 0.000000000000000000 ) ) ;
#17847=EDGE_CURVE ( 'NONE', #20212, #9275, #17211, .T. ) ;
#17848=VECTOR ( 'NONE', #4954, 1000.000000000000000 ) ;
#17851=DIRECTION ( 'NONE',  ( -0.9781142164131917394, 0.2080686897406911207, 0.000000000000000000 ) ) ;
#17852=DIRECTION ( 'NONE',  ( 1.000000000000000000, 0.000000000000000000, 0.000000000000000000 ) ) ;
#17855=ORIENTED_EDGE ( 'NONE', *, *, #9875, .T. ) ;
#17857=EDGE_CURVE ( 'NONE', #9195, #1303, #6801, .T. ) ;
#17858=VECTOR ( 'NONE', #19437, 1000.000000000000227 ) ;
#17859=ORIENTED_EDGE ( 'NONE', *, *, #1393, .T. ) ;
#17862=ORIENTED_EDGE ( 'NONE', *, *, #4627, .F. ) ;
#17865=ADVANCED_FACE ( 'NONE', ( #12280 ), #4724, .F. ) ;
#17866=DIRECTION ( 'NONE',  ( 1.000000000000000000, 0.000000000000000000, 0.000000000000000000 ) ) ;
#17869=DIRECTION ( 'NONE',  ( -0.6427876096865404731, 0.7660444431189771253, 0.000000000000000000 ) ) ;
#17870=CARTESIAN_POINT ( 'NONE',  ( 0.4239815141812912636, -0.2650276884262227628, 283.5832628385307999 ) ) ;
#17871=PLANE ( 'NONE',  #19227 ) ;
#17872=VERTEX_POINT ( 'NONE', #10950 ) ;
#17874=DIRECTION ( 'NONE',  ( 0.000000000000000000, 0.000000000000000000, -1.000000000000000000 ) ) ;
#17875=VECTOR ( 'NONE', #10683, 1000.000000000000000 ) ;
#17879=CARTESIAN_POINT ( 'NONE',  ( -78.26059000578311498, 0.8220851292432551638, 132.4711112102474146 ) ) ;
#17881=DIRECTION ( 'NONE',  ( -0.000000000000000000, -0.000000000000000000, 1.000000000000000000 ) ) ;
#17882=VECTOR ( 'NONE', #10310, 1000.000000000000114 ) ;
#17885=DIRECTION ( 'NONE',  ( 0.1736481776669241417, 0.9848077530122091305, 0.000000000000000000 ) ) ;
#17889=ORIENTED_EDGE ( 'NONE', *, *, #12490, .T. ) ;
#17890=EDGE_CURVE ( 'NONE', #13973, #4841, #15673, .T. ) ;
#17891=ORIENTED_EDGE ( 'NONE', *, *, #731, .T. ) ;
#17892=EDGE_CURVE ( 'NONE', #15414, #3831, #11047, .T. ) ;
#17899=CARTESIAN_POINT ( 'NONE',  ( -60.47951622432784546, -49.67518383744813804, 110.7293897666001214 ) ) ;
#17902=EDGE_CURVE ( 'NONE', #399, #9468, #12796, .T. ) ;
#17904=DIRECTION ( 'NONE',  ( -0.8830229359480271656, -0.4693298356057563625, 0.000000000000000000 ) ) ;
#17905=CARTESIAN_POINT ( 'NONE',  ( 10.99904278960855386, 0.5388563210141777970, 248.9926560891072143 ) ) ;
#17907=ORIENTED_EDGE ( 'NONE', *, *, #4681, .T. ) ;
#17908=DIRECTION ( 'NONE',  ( -0.000000000000000000, -0.000000000000000000, 1.000000000000000000 ) ) ;
#17915=CARTESIAN_POINT ( 'NONE',  ( -58.63718168490500204, -22.81000261549350228, 248.9926560891072143 ) ) ;
#17916=CARTESIAN_POINT ( 'NONE',  ( 37.09555676056997697, -45.48770046196272432, 248.9926560891072143 ) ) ;
#17917=EDGE_CURVE ( 'NONE', #5730, #1356, #6469, .T. ) ;
#17918=ORIENTED_EDGE ( 'NONE', *, *, #8998, .T. ) ;
#17919=EDGE_CURVE ( 'NONE', #9982, #13894, #14232, .T. ) ;
#17921=ORIENTED_EDGE ( 'NONE', *, *, #13518, .F. ) ;
#17926=ORIENTED_EDGE ( 'NONE', *, *, #2154, .T. ) ;
#17927=AXIS2_PLACEMENT_3D ( 'NONE', #18626, #197, #14214 ) ;
#17931=CIRCLE ( 'NONE', #16940, 62.91752772691707207 ) ;
#17932=PLANE ( 'NONE',  #5559 ) ;
#17933=FACE_OUTER_BOUND ( 'NONE', #2507, .T. ) ;
#17934=FACE_OUTER_BOUND ( 'NONE', #16196, .T. ) ;
#17935=LINE ( 'NONE', #3904, #10197 ) ;
#17936=CARTESIAN_POINT ( 'NONE',  ( 45.46865632508072963, -40.28046525994365368, 283.5832628385307999 ) ) ;
#17937=DIRECTION ( 'NONE',  ( -0.000000000000000000, -0.000000000000000000, 1.000000000000000000 ) ) ;
#17938=LINE ( 'NONE', #1029, #94 ) ;
#17940=CARTESIAN_POINT ( 'NONE',  ( -8.938941455414985526, 60.08127757648384915, 293.5832628385307999 ) ) ;
#17941=CARTESIAN_POINT ( 'NONE',  ( 57.92514141135453087, 18.28503710798567994, 283.5832628385307999 ) ) ;
#17942=AXIS2_PLACEMENT_3D ( 'NONE', #10806, #13980, #2844 ) ;
#17943=CIRCLE ( 'NONE', #13682, 62.91752772691707207 ) ;
#17945=VECTOR ( 'NONE', #8851, 1000.000000000000114 ) ;
#17946=ORIENTED_EDGE ( 'NONE', *, *, #15223, .F. ) ;
#17947=EDGE_LOOP ( 'NONE', ( #765, #17216, #5565, #14548 ) ) ;
#17952=CARTESIAN_POINT ( 'NONE',  ( -44.07268132743698175, -38.78191089773056177, 132.4711112102474146 ) ) ;
#17953=LINE ( 'NONE', #11401, #19240 ) ;
#17955=FACE_OUTER_BOUND ( 'NONE', #19542, .T. ) ;
#17956=VECTOR ( 'NONE', #9669, 1000.000000000000000 ) ;
#17959=LINE ( 'NONE', #19483, #3975 ) ;
#17960=CYLINDRICAL_SURFACE ( 'NONE', #1007, 60.74260934110282051 ) ;
#17964=ORIENTED_EDGE ( 'NONE', *, *, #8045, .T. ) ;
#17968=EDGE_LOOP ( 'NONE', ( #16754, #12305, #1093, #8637 ) ) ;
#17969=EDGE_CURVE ( 'NONE', #18064, #16227, #11156, .T. ) ;
#17971=ORIENTED_EDGE ( 'NONE', *, *, #15464, .F. ) ;
#17972=DIRECTION ( 'NONE',  ( -0.8479630283625698706, 0.5300553768524376430, 0.000000000000000000 ) ) ;
#17973=DIRECTION ( 'NONE',  ( 3.491481338843133355E-15, -1.000000000000000000, 0.000000000000000000 ) ) ;
#17974=DIRECTION ( 'NONE',  ( 1.000000000000000000, 0.000000000000000000, 0.000000000000000000 ) ) ;
#17976=LINE ( 'NONE', #17776, #16840 ) ;
#17977=CARTESIAN_POINT ( 'NONE',  ( -59.30716253403183202, 13.12726406102060217, 293.5832628385307999 ) ) ;
#17978=VERTEX_POINT ( 'NONE', #18847 ) ;
#17979=CARTESIAN_POINT ( 'NONE',  ( 40.32479851956816930, -67.08601213326551260, 132.4711112102474146 ) ) ;
#17980=EDGE_CURVE ( 'NONE', #934, #1238, #19055, .T. ) ;
#17981=CARTESIAN_POINT ( 'NONE',  ( -22.30005961346265408, -56.50329132715937419, 293.5832628385307999 ) ) ;
#17983=CIRCLE ( 'NONE', #18971, 60.74260934110282051 ) ;
#17986=DIRECTION ( 'NONE',  ( 0.5000000000000101030, -0.8660254037844328234, 0.000000000000000000 ) ) ;
#17987=EDGE_LOOP ( 'NONE', ( #6518, #19030, #7212, #1396 ) ) ;
#17988=DIRECTION ( 'NONE',  ( -0.000000000000000000, -0.000000000000000000, 1.000000000000000000 ) ) ;
#17989=ORIENTED_EDGE ( 'NONE', *, *, #6788, .F. ) ;
#17990=ORIENTED_EDGE ( 'NONE', *, *, #1365, .F. ) ;
#17991=EDGE_CURVE ( 'NONE', #8910, #5730, #8192, .T. ) ;
#17993=ORIENTED_EDGE ( 'NONE', *, *, #11030, .T. ) ;
#17996=DIRECTION ( 'NONE',  ( -0.9396926207859104263, 0.3420201433256630508, 0.000000000000000000 ) ) ;
#17997=DIRECTION ( 'NONE',  ( 0.7660444431189749048, 0.6427876096865430267, 0.000000000000000000 ) ) ;
#18000=ADVANCED_FACE ( 'NONE', ( #17520 ), #17318, .T. ) ;
#18004=EDGE_CURVE ( 'NONE', #3096, #10368, #2067, .T. ) ;
#18008=DIRECTION ( 'NONE',  ( -0.1390141521205912334, 0.9902903945359629034, 0.000000000000000000 ) ) ;
#18013=CARTESIAN_POINT ( 'NONE',  ( 61.81362617575100415, -11.73417718768069840, 248.9926560891072143 ) ) ;
#18016=AXIS2_PLACEMENT_3D ( 'NONE', #550, #7906, #1679 ) ;
#18018=DIRECTION ( 'NONE',  ( 0.3420201433256790380, -0.9396926207859046531, 0.000000000000000000 ) ) ;
#18019=AXIS2_PLACEMENT_3D ( 'NONE', #15063, #1042, #7291 ) ;
#18020=FACE_OUTER_BOUND ( 'NONE', #5013, .T. ) ;
#18023=DIRECTION ( 'NONE',  ( 0.7660444431189771253, 0.6427876096865405842, 0.000000000000000000 ) ) ;
#18026=ADVANCED_FACE ( 'NONE', ( #11365 ), #6864, .T. ) ;
#18029=LINE ( 'NONE', #16494, #17139 ) ;
#18031=DIRECTION ( 'NONE',  ( 0.000000000000000000, 0.000000000000000000, 1.000000000000000000 ) ) ;
#18033=CARTESIAN_POINT ( 'NONE',  ( 78.26059000578310076, 1.379293853802574743, 112.7772637782949516 ) ) ;
#18034=EDGE_LOOP ( 'NONE', ( #6477, #11690, #20171, #9073 ) ) ;
#18036=LINE ( 'NONE', #11969, #14150 ) ;
#18037=ORIENTED_EDGE ( 'NONE', *, *, #19369, .F. ) ;
#18039=VECTOR ( 'NONE', #16616, 999.9999999999998863 ) ;
#18040=ORIENTED_EDGE ( 'NONE', *, *, #13228, .F. ) ;
#18041=LINE ( 'NONE', #16508, #4798 ) ;
#18042=ORIENTED_EDGE ( 'NONE', *, *, #6159, .F. ) ;
#18044=DIRECTION ( 'NONE',  ( 0.8660254037844449249, -0.4999999999999888978, 0.000000000000000000 ) ) ;
#18045=CARTESIAN_POINT ( 'NONE',  ( 60.74260934110282051, 0.000000000000000000, 283.5832628385307999 ) ) ;
#18046=EDGE_CURVE ( 'NONE', #399, #4738, #3868, .T. ) ;
#18047=DIRECTION ( 'NONE',  ( 0.000000000000000000, 0.000000000000000000, 1.000000000000000000 ) ) ;
#18054=CARTESIAN_POINT ( 'NONE',  ( 67.36461649554532016, -39.84224160888924615, 110.9660488491357455 ) ) ;
#18057=ORIENTED_EDGE ( 'NONE', *, *, #1789, .F. ) ;
#18058=AXIS2_PLACEMENT_3D ( 'NONE', #14848, #16499, #5748 ) ;
#18060=ORIENTED_EDGE ( 'NONE', *, *, #8222, .F. ) ;
#18063=CIRCLE ( 'NONE', #15448, 60.74260934110282051 ) ;
#18064=VERTEX_POINT ( 'NONE', #17915 ) ;
#18065=CARTESIAN_POINT ( 'NONE',  ( -57.92514141135452377, -18.28503710798565152, 283.5832628385307999 ) ) ;
#18066=CARTESIAN_POINT ( 'NONE',  ( -13.12726406102078336, -59.30716253403180360, 283.5832628385307999 ) ) ;
#18070=DIRECTION ( 'NONE',  ( 0.000000000000000000, 0.000000000000000000, 1.000000000000000000 ) ) ;
#18072=DIRECTION ( 'NONE',  ( 1.000000000000000000, 0.000000000000000000, 0.000000000000000000 ) ) ;
#18074=CARTESIAN_POINT ( 'NONE',  ( 20.74471755083603597, -59.39925916207552348, 248.9926560891072143 ) ) ;
#18075=LINE ( 'NONE', #8754, #45 ) ;
#18076=VECTOR ( 'NONE', #17988, 1000.000000000000000 ) ;
#18080=ORIENTED_EDGE ( 'NONE', *, *, #19887, .F. ) ;
#18081=CARTESIAN_POINT ( 'NONE',  ( -60.68567895461851691, 2.629250726500500956, 293.5832628385307999 ) ) ;
#18082=ORIENTED_EDGE ( 'NONE', *, *, #4911, .T. ) ;
#18086=CIRCLE ( 'NONE', #2420, 62.91752772691707207 ) ;
#18087=ORIENTED_EDGE ( 'NONE', *, *, #5757, .T. ) ;
#18088=EDGE_LOOP ( 'NONE', ( #17503, #15443, #263 ) ) ;
#18091=CARTESIAN_POINT ( 'NONE',  ( 78.26059000578312919, -0.8220851292427139301, 132.4711112102474146 ) ) ;
#18094=CARTESIAN_POINT ( 'NONE',  ( -1.678175111358159333, -5.485913980968224912, 293.5832628385307999 ) ) ;
#18095=DIRECTION ( 'NONE',  ( -0.000000000000000000, -0.000000000000000000, 1.000000000000000000 ) ) ;
#18096=EDGE_CURVE ( 'NONE', #15899, #18157, #10220, .T. ) ;
#18097=LINE ( 'NONE', #2932, #13723 ) ;
#18099=ORIENTED_EDGE ( 'NONE', *, *, #4270, .T. ) ;
#18101=DIRECTION ( 'NONE',  ( -0.2080686897406911207, -0.9781142164131917394, 0.000000000000000000 ) ) ;
#18103=CARTESIAN_POINT ( 'NONE',  ( -22.81000261549329267, 58.63718168490507310, 248.9926560891072143 ) ) ;
#18106=CARTESIAN_POINT ( 'NONE',  ( 0.000000000000000000, 0.000000000000000000, 283.5832628385307999 ) ) ;
#18107=VERTEX_POINT ( 'NONE', #14636 ) ;
#18108=ORIENTED_EDGE ( 'NONE', *, *, #6, .F. ) ;
#18110=EDGE_CURVE ( 'NONE', #16849, #3604, #17931, .T. ) ;
#18112=ADVANCED_FACE ( 'NONE', ( #2358 ), #16285, .F. ) ;
#18115=VECTOR ( 'NONE', #19378, 1000.000000000000000 ) ;
#18117=LINE ( 'NONE', #1119, #19471 ) ;
#18118=DIRECTION ( 'NONE',  ( 1.000000000000000000, 0.000000000000000000, 0.000000000000000000 ) ) ;
#18119=EDGE_CURVE ( 'NONE', #1551, #10080, #621, .T. ) ;
#18122=CARTESIAN_POINT ( 'NONE',  ( 54.67896814532641514, 21.36933070621782349, 132.4711112102474146 ) ) ;
#18124=LINE ( 'NONE', #13201, #8141 ) ;
#18125=CARTESIAN_POINT ( 'NONE',  ( 57.65577537092158877, -11.00103590902891249, 248.9926560891072143 ) ) ;
#18127=DIRECTION ( 'NONE',  ( 0.1390141521205912056, -0.9902903945359629034, 0.000000000000000000 ) ) ;
#18128=DIRECTION ( 'NONE',  ( 1.000000000000000000, 0.000000000000000000, 0.000000000000000000 ) ) ;
#18130=ORIENTED_EDGE ( 'NONE', *, *, #12105, .F. ) ;
#18132=EDGE_CURVE ( 'NONE', #15095, #6267, #4184, .T. ) ;
#18134=EDGE_CURVE ( 'NONE', #2090, #9172, #8117, .T. ) ;
#18138=CARTESIAN_POINT ( 'NONE',  ( 41.02350267428969488, 44.79940644582669051, 293.5832628385307999 ) ) ;
#18139=CARTESIAN_POINT ( 'NONE',  ( 0.000000000000000000, 0.000000000000000000, 283.5832628385307999 ) ) ;
#18142=ORIENTED_EDGE ( 'NONE', *, *, #4601, .T. ) ;
#18143=CYLINDRICAL_SURFACE ( 'NONE', #20221, 60.74260934110282051 ) ;
#18146=CARTESIAN_POINT ( 'NONE',  ( 51.23821591265094355, 28.63313560863489471, 248.9926560891072143 ) ) ;
#18147=DIRECTION ( 'NONE',  ( -0.000000000000000000, -0.000000000000000000, 1.000000000000000000 ) ) ;
#18148=VECTOR ( 'NONE', #200, 1000.000000000000000 ) ;
#18149=FACE_OUTER_BOUND ( 'NONE', #5768, .T. ) ;
#18152=VERTEX_POINT ( 'NONE', #19730 ) ;
#18157=VERTEX_POINT ( 'NONE', #5624 ) ;
#18160=CIRCLE ( 'NONE', #14533, 60.74260934110282051 ) ;
#18161=CARTESIAN_POINT ( 'NONE',  ( 56.50329132715945235, -22.30005961346246579, 293.5832628385307999 ) ) ;
#18162=CARTESIAN_POINT ( 'NONE',  ( 44.79787735033391272, -41.02212542604627288, 283.5832628385307999 ) ) ;
#18163=ORIENTED_EDGE ( 'NONE', *, *, #4898, .T. ) ;
#18165=DIRECTION ( 'NONE',  ( 1.000000000000000000, 0.000000000000000000, 0.000000000000000000 ) ) ;
#18166=EDGE_LOOP ( 'NONE', ( #4415, #12802 ) ) ;
#18167=CARTESIAN_POINT ( 'NONE',  ( -45.46712722958807973, 40.27908801170008957, 283.5832628385307999 ) ) ;
#18170=CARTESIAN_POINT ( 'NONE',  ( 5.111158570922285982, -2.605298826210321383, 293.5832628385307999 ) ) ;
#18173=CARTESIAN_POINT ( 'NONE',  ( 60.47951622432751151, 49.67518383744852883, 248.9926560891072143 ) ) ;
#18174=DIRECTION ( 'NONE',  ( 1.000000000000000000, 0.000000000000000000, 0.000000000000000000 ) ) ;
#18175=ORIENTED_EDGE ( 'NONE', *, *, #17268, .T. ) ;
#18179=ORIENTED_EDGE ( 'NONE', *, *, #705, .T. ) ;
#18181=DIRECTION ( 'NONE',  ( 1.000000000000000000, 0.000000000000000000, 0.000000000000000000 ) ) ;
#18182=ORIENTED_EDGE ( 'NONE', *, *, #10019, .T. ) ;
#18184=VECTOR ( 'NONE', #9594, 1000.000000000000000 ) ;
#18185=CARTESIAN_POINT ( 'NONE',  ( -17.50000000000001066, 2.143131898507869431E-15, 4.999999999999948486 ) ) ;
#18186=VECTOR ( 'NONE', #2669, 1000.000000000000227 ) ;
#18188=CARTESIAN_POINT ( 'NONE',  ( -13.12769224524071277, -59.30917539369501412, 293.5832628385307999 ) ) ;
#18190=LINE ( 'NONE', #5924, #2454 ) ;
#18191=EDGE_LOOP ( 'NONE', ( #19566, #9939, #8526, #17166 ) ) ;
#18194=LINE ( 'NONE', #15020, #8116 ) ;
#18195=PLANE ( 'NONE',  #17497 ) ;
#18196=ORIENTED_EDGE ( 'NONE', *, *, #7466, .T. ) ;
#18197=CARTESIAN_POINT ( 'NONE',  ( 59.58067424803626011, -20.21777810286696564, 293.5832628385307999 ) ) ;
#18201=CARTESIAN_POINT ( 'NONE',  ( 0.000000000000000000, 0.000000000000000000, 283.5832628385307999 ) ) ;
#18202=DIRECTION ( 'NONE',  ( 0.000000000000000000, 0.000000000000000000, 1.000000000000000000 ) ) ;
#18204=ORIENTED_EDGE ( 'NONE', *, *, #12850, .T. ) ;
#18205=CARTESIAN_POINT ( 'NONE',  ( 57.92709869106709419, 18.28567271940532990, 293.5832628385307999 ) ) ;
#18207=ORIENTED_EDGE ( 'NONE', *, *, #5226, .T. ) ;
#18208=ADVANCED_FACE ( 'NONE', ( #2557 ), #814, .T. ) ;
#18210=CARTESIAN_POINT ( 'NONE',  ( 30.09424155357379504, 27.05260723904837761, 248.9926560891072143 ) ) ;
#18213=CARTESIAN_POINT ( 'NONE',  ( -76.83212392882499842, -14.94814811854936210, 112.0427633081291816 ) ) ;
#18216=DIRECTION ( 'NONE',  ( 0.9396926207859092051, -0.3420201433256662704, 0.000000000000000000 ) ) ;
#18222=CARTESIAN_POINT ( 'NONE',  ( 0.000000000000000000, 0.000000000000000000, 132.4711112102474146 ) ) ;
#18223=PLANE ( 'NONE',  #18058 ) ;
#18224=ORIENTED_EDGE ( 'NONE', *, *, #19859, .F. ) ;
#18225=EDGE_CURVE ( 'NONE', #1059, #10466, #10511, .T. ) ;
#18227=DIRECTION ( 'NONE',  ( -0.9511061040868794558, -0.3088643371590157338, 0.000000000000000000 ) ) ;
#18228=VERTEX_POINT ( 'NONE', #4386 ) ;
#18230=VERTEX_POINT ( 'NONE', #10615 ) ;
#18238=CARTESIAN_POINT ( 'NONE',  ( -62.91215678473958661, 0.8220851292433132285, 132.4711112102474146 ) ) ;
#18240=DIRECTION ( 'NONE',  ( 0.9848077530122069101, 0.1736481776669374644, 0.000000000000000000 ) ) ;
#18249=VECTOR ( 'NONE', #4907, 1000.000000000000227 ) ;
#18250=ORIENTED_EDGE ( 'NONE', *, *, #13252, .F. ) ;
#18252=AXIS2_PLACEMENT_3D ( 'NONE', #19504, #11806, #687 ) ;
#18253=DIRECTION ( 'NONE',  ( 1.000000000000000000, 0.000000000000000000, -0.000000000000000000 ) ) ;
#18256=VERTEX_POINT ( 'NONE', #13581 ) ;
#18257=EDGE_CURVE ( 'NONE', #4516, #10035, #20137, .T. ) ;
#18260=AXIS2_PLACEMENT_3D ( 'NONE', #15640, #7853, #18819 ) ;
#18262=CIRCLE ( 'NONE', #10736, 17.50000000000001066 ) ;
#18265=ORIENTED_EDGE ( 'NONE', *, *, #9369, .F. ) ;
#18267=CARTESIAN_POINT ( 'NONE',  ( 56.12662799072089115, -23.22641211976269915, 293.5832628385307999 ) ) ;
#18270=CARTESIAN_POINT ( 'NONE',  ( -60.47951622432783125, -49.67518383744813804, 132.4711112102474146 ) ) ;
#18277=EDGE_CURVE ( 'NONE', #4586, #6529, #5842, .T. ) ;
#18278=DIRECTION ( 'NONE',  ( 0.9396926207859126468, -0.3420201433256568335, 0.000000000000000000 ) ) ;
#18280=AXIS2_PLACEMENT_3D ( 'NONE', #15337, #4293, #1115 ) ;
#18281=VECTOR ( 'NONE', #7615, 1000.000000000000000 ) ;
#18285=ORIENTED_EDGE ( 'NONE', *, *, #18418, .F. ) ;
#18287=CARTESIAN_POINT ( 'NONE',  ( 47.66508197439472383, -41.06890862491489003, 293.5832628385307999 ) ) ;
#18289=ORIENTED_EDGE ( 'NONE', *, *, #535, .F. ) ;
#18290=EDGE_LOOP ( 'NONE', ( #12620, #4388, #13532, #10678 ) ) ;
#18291=CARTESIAN_POINT ( 'NONE',  ( 10.11498556985160846, -62.09913334491126591, 293.5832628385307999 ) ) ;
#18295=LINE ( 'NONE', #4271, #8680 ) ;
#18297=ORIENTED_EDGE ( 'NONE', *, *, #370, .T. ) ;
#18299=DIRECTION ( 'NONE',  ( 1.000000000000000000, 0.000000000000000000, 0.000000000000000000 ) ) ;
#18301=CARTESIAN_POINT ( 'NONE',  ( -1.379293853801755176, 78.26059000578311498, 248.9926560891072143 ) ) ;
#18304=FACE_OUTER_BOUND ( 'NONE', #16294, .T. ) ;
#18306=ADVANCED_FACE ( 'NONE', ( #2519 ), #14889, .F. ) ;
#18307=ORIENTED_EDGE ( 'NONE', *, *, #17554, .F. ) ;
#18308=VECTOR ( 'NONE', #3783, 1000.000000000000000 ) ;
#18310=CARTESIAN_POINT ( 'NONE',  ( 78.26059000578312919, -0.8220851292427129309, 248.9926560891072143 ) ) ;
#18312=VERTEX_POINT ( 'NONE', #17979 ) ;
#18313=VECTOR ( 'NONE', #14937, 1000.000000000000114 ) ;
#18315=DIRECTION ( 'NONE',  ( 0.000000000000000000, 0.000000000000000000, 1.000000000000000000 ) ) ;
#18318=CARTESIAN_POINT ( 'NONE',  ( 5.693982670708940041, -0.7000608949449556029, 293.5832628385307999 ) ) ;
#18319=ORIENTED_EDGE ( 'NONE', *, *, #4627, .T. ) ;
#18321=FACE_OUTER_BOUND ( 'NONE', #15574, .T. ) ;
#18322=AXIS2_PLACEMENT_3D ( 'NONE', #9269, #4673, #4565 ) ;
#18325=FACE_OUTER_BOUND ( 'NONE', #8785, .T. ) ;
#18331=FACE_OUTER_BOUND ( 'NONE', #3943, .T. ) ;
#18333=ORIENTED_EDGE ( 'NONE', *, *, #8414, .T. ) ;
#18334=VECTOR ( 'NONE', #20055, 1000.000000000000114 ) ;
#18336=SHAPE_REPRESENTATION_RELATIONSHIP ( 'NONE' , 'NONE' ,  #13949, #16290 ) ;
#18337=ORIENTED_EDGE ( 'NONE', *, *, #1883, .T. ) ;
#18338=FACE_BOUND ( 'NONE', #7813, .T. ) ;
#18340=CARTESIAN_POINT ( 'NONE',  ( -36.99387960884162396, 48.17797692984176194, 283.5832628385307999 ) ) ;
#18343=DIRECTION ( 'NONE',  ( -0.4693298356057531429, 0.8830229359480288309, 0.000000000000000000 ) ) ;
#18347=CARTESIAN_POINT ( 'NONE',  ( -60.72073886220397299, 1.629865514042312613, 293.5832628385307999 ) ) ;
#18350=DIRECTION ( 'NONE',  ( -0.000000000000000000, -0.000000000000000000, 1.000000000000000000 ) ) ;
#18353=EDGE_CURVE ( 'NONE', #17702, #19638, #14665, .T. ) ;
#18356=ORIENTED_EDGE ( 'NONE', *, *, #2145, .T. ) ;
#18360=ORIENTED_EDGE ( 'NONE', *, *, #15787, .T. ) ;
#18361=EDGE_CURVE ( 'NONE', #12098, #274, #14796, .T. ) ;
#18366=DIRECTION ( 'NONE',  ( 0.9848077530122062440, 0.1736481776669404620, 0.000000000000000000 ) ) ;
#18367=ORIENTED_EDGE ( 'NONE', *, *, #18534, .F. ) ;
#18368=VECTOR ( 'NONE', #14177, 1000.000000000000114 ) ;
#18370=CARTESIAN_POINT ( 'NONE',  ( -73.25972925305609351, 27.53920554013712874, 248.9926560891072143 ) ) ;
#18372=FACE_OUTER_BOUND ( 'NONE', #9779, .T. ) ;
#18373=DIRECTION ( 'NONE',  ( 0.000000000000000000, 0.000000000000000000, 1.000000000000000000 ) ) ;
#18375=VECTOR ( 'NONE', #2758, 1000.000000000000000 ) ;
#18377=ADVANCED_FACE ( 'NONE', ( #13346 ), #974, .F. ) ;
#18379=DIRECTION ( 'NONE',  ( 0.000000000000000000, 0.000000000000000000, -1.000000000000000000 ) ) ;
#18381=VERTEX_POINT ( 'NONE', #5587 ) ;
#18382=CYLINDRICAL_SURFACE ( 'NONE', #7359, 62.91752772691707207 ) ;
#18383=VECTOR ( 'NONE', #11941, 1000.000000000000114 ) ;
#18384=VECTOR ( 'NONE', #14941, 1000.000000000000227 ) ;
#18385=VERTEX_POINT ( 'NONE', #16341 ) ;
#18387=PLANE ( 'NONE',  #1742 ) ;
#18389=EDGE_LOOP ( 'NONE', ( #4309, #11293, #341, #67 ) ) ;
#18390=EDGE_CURVE ( 'NONE', #3300, #19783, #5491, .T. ) ;
#18392=ADVANCED_FACE ( 'NONE', ( #15087 ), #10188, .T. ) ;
#18394=CARTESIAN_POINT ( 'NONE',  ( -39.84224160888947353, -67.36461649554519227, 110.9660488491356887 ) ) ;
#18395=DIRECTION ( 'NONE',  ( 1.000000000000000000, 0.000000000000000000, 0.000000000000000000 ) ) ;
#18396=ORIENTED_EDGE ( 'NONE', *, *, #8861, .T. ) ;
#18398=CARTESIAN_POINT ( 'NONE',  ( -59.51523122377251696, 12.14914984460740754, 293.5832628385307999 ) ) ;
#18400=CARTESIAN_POINT ( 'NONE',  ( 56.12853591711344592, -23.22718332831461652, 283.5832628385307999 ) ) ;
#18401=LINE ( 'NONE', #7344, #8763 ) ;
#18404=CARTESIAN_POINT ( 'NONE',  ( 7.948651060879040386, -60.22029172860440127, 283.5832628385307999 ) ) ;
#18405=EDGE_CURVE ( 'NONE', #17256, #13906, #2570, .T. ) ;
#18406=CARTESIAN_POINT ( 'NONE',  ( 68.46530598706794990, -37.93579148621486041, 110.9660488491357455 ) ) ;
#18407=CIRCLE ( 'NONE', #5343, 62.91752772691707207 ) ;
#18410=ORIENTED_EDGE ( 'NONE', *, *, #1659, .F. ) ;
#18413=ORIENTED_EDGE ( 'NONE', *, *, #15024, .F. ) ;
#18414=ORIENTED_EDGE ( 'NONE', *, *, #10494, .F. ) ;
#18416=AXIS2_PLACEMENT_3D ( 'NONE', #14414, #3467, #297 ) ;
#18417=EDGE_CURVE ( 'NONE', #2011, #18157, #13547, .T. ) ;
#18418=EDGE_CURVE ( 'NONE', #14186, #2886, #19797, .T. ) ;
#18419=ORIENTED_EDGE ( 'NONE', *, *, #18527, .F. ) ;
#18425=FACE_BOUND ( 'NONE', #10458, .T. ) ;
#18426=EDGE_CURVE ( 'NONE', #18461, #1479, #4249, .T. ) ;
#18427=EDGE_CURVE ( 'NONE', #11985, #11201, #16314, .T. ) ;
#18429=DIRECTION ( 'NONE',  ( -0.9396926207859046531, -0.3420201433256790380, 0.000000000000000000 ) ) ;
#18431=FACE_OUTER_BOUND ( 'NONE', #19394, .T. ) ;
#18432=CARTESIAN_POINT ( 'NONE',  ( -25.99419088092141550, 73.82206860051556419, 132.4711112102474146 ) ) ;
#18435=DIRECTION ( 'NONE',  ( -0.03505990758545895342, -0.9993852124581886764, 0.000000000000000000 ) ) ;
#18436=CARTESIAN_POINT ( 'NONE',  ( 40.27908801169993325, 45.46712722958823605, 293.5832628385307999 ) ) ;
#18438=VECTOR ( 'NONE', #13005, 1000.000000000000000 ) ;
#18440=ORIENTED_EDGE ( 'NONE', *, *, #18257, .T. ) ;
#18441=FACE_BOUND ( 'NONE', #5999, .T. ) ;
#18442=ORIENTED_EDGE ( 'NONE', *, *, #9134, .F. ) ;
#18443=DIRECTION ( 'NONE',  ( -0.000000000000000000, -0.000000000000000000, 1.000000000000000000 ) ) ;
#18446=VECTOR ( 'NONE', #4824, 1000.000000000000227 ) ;
#18448=ORIENTED_EDGE ( 'NONE', *, *, #16128, .F. ) ;
#18449=DIRECTION ( 'NONE',  ( 1.000000000000000000, 0.000000000000000000, 0.000000000000000000 ) ) ;
#18450=DIRECTION ( 'NONE',  ( -0.000000000000000000, -0.000000000000000000, 1.000000000000000000 ) ) ;
#18453=CARTESIAN_POINT ( 'NONE',  ( 76.83212392882491315, 14.94814811854985948, 132.4711112102474146 ) ) ;
#18455=ORIENTED_EDGE ( 'NONE', *, *, #13395, .T. ) ;
#18461=VERTEX_POINT ( 'NONE', #8947 ) ;
#18462=EDGE_CURVE ( 'NONE', #15722, #9575, #15606, .T. ) ;
#18463=CARTESIAN_POINT ( 'NONE',  ( 27.93373560431201241, 14.53487841505346445, 248.9926560891072143 ) ) ;
#18464=CARTESIAN_POINT ( 'NONE',  ( -21.51741588379869441, 55.08582882688753557, 248.9926560891072143 ) ) ;
#18465=ORIENTED_EDGE ( 'NONE', *, *, #12968, .F. ) ;
#18468=DIRECTION ( 'NONE',  ( 1.000000000000000000, 0.000000000000000000, 0.000000000000000000 ) ) ;
#18469=VERTEX_POINT ( 'NONE', #18579 ) ;
#18470=FACE_OUTER_BOUND ( 'NONE', #6621, .T. ) ;
#18471=DIRECTION ( 'NONE',  ( -0.000000000000000000, -0.000000000000000000, 1.000000000000000000 ) ) ;
#18475=ADVANCED_FACE ( 'NONE', ( #18470 ), #15191, .F. ) ;
#18477=CARTESIAN_POINT ( 'NONE',  ( 47.56244194535165093, 37.78198917157335757, 283.5832628385307999 ) ) ;
#18479=ORIENTED_EDGE ( 'NONE', *, *, #13026, .F. ) ;
#18483=ORIENTED_EDGE ( 'NONE', *, *, #5616, .T. ) ;
#18485=ORIENTED_EDGE ( 'NONE', *, *, #13074, .F. ) ;
#18486=CARTESIAN_POINT ( 'NONE',  ( 1.289614712049190981, -5.590028426173843101, 293.5832628385307999 ) ) ;
#18487=ORIENTED_EDGE ( 'NONE', *, *, #14342, .T. ) ;
#18489=EDGE_CURVE ( 'NONE', #5705, #3256, #12526, .T. ) ;
#18493=EDGE_LOOP ( 'NONE', ( #18485, #13583, #16977, #3350 ) ) ;
#18497=VERTEX_POINT ( 'NONE', #7618 ) ;
#18498=LINE ( 'NONE', #6334, #5443 ) ;
#18499=CARTESIAN_POINT ( 'NONE',  ( 8.833100819207578169, 58.03804081968171147, 132.4711112102474146 ) ) ;
#18500=DIRECTION ( 'NONE',  ( -0.000000000000000000, -0.000000000000000000, 1.000000000000000000 ) ) ;
#18507=ORIENTED_EDGE ( 'NONE', *, *, #6788, .T. ) ;
#18510=CARTESIAN_POINT ( 'NONE',  ( -5.281164089014709795, -2.240720816136031690, 283.5832628385307999 ) ) ;
#18512=VECTOR ( 'NONE', #13443, 999.9999999999998863 ) ;
#18513=ORIENTED_EDGE ( 'NONE', *, *, #6243, .F. ) ;
#18514=FACE_OUTER_BOUND ( 'NONE', #5627, .T. ) ;
#18515=ORIENTED_EDGE ( 'NONE', *, *, #10037, .F. ) ;
#18517=CONICAL_SURFACE ( 'NONE', #13608, 62.91752772691707207, 0.5206510040058940358 ) ;
#18518=ADVANCED_FACE ( 'NONE', ( #18372 ), #19998, .T. ) ;
#18519=DIRECTION ( 'NONE',  ( 0.000000000000000000, 0.000000000000000000, 1.000000000000000000 ) ) ;
#18522=LINE ( 'NONE', #4502, #7024 ) ;
#18524=FACE_OUTER_BOUND ( 'NONE', #19785, .T. ) ;
#18527=EDGE_CURVE ( 'NONE', #1, #13430, #6000, .T. ) ;
#18528=PLANE ( 'NONE',  #12959 ) ;
#18530=LINE ( 'NONE', #18641, #14777 ) ;
#18533=ORIENTED_EDGE ( 'NONE', *, *, #10321, .F. ) ;
#18534=EDGE_CURVE ( 'NONE', #1943, #13278, #8226, .T. ) ;
#18536=DIRECTION ( 'NONE',  ( -0.8479630283625698706, 0.5300553768524376430, 0.000000000000000000 ) ) ;
#18537=CARTESIAN_POINT ( 'NONE',  ( -77.31114765718486126, 12.23146955673672842, 248.9926560891072143 ) ) ;
#18538=ORIENTED_EDGE ( 'NONE', *, *, #7531, .T. ) ;
#18542=FACE_BOUND ( 'NONE', #16846, .T. ) ;
#18545=LINE ( 'NONE', #20177, #10246 ) ;
#18549=VECTOR ( 'NONE', #13609, 1000.000000000000000 ) ;
#18552=DIRECTION ( 'NONE',  ( 0.000000000000000000, 0.000000000000000000, -1.000000000000000000 ) ) ;
#18557=EDGE_CURVE ( 'NONE', #9538, #9804, #9439, .T. ) ;
#18558=CARTESIAN_POINT ( 'NONE',  ( -28.15057869795625578, -51.51682027493055216, 110.9660488491356887 ) ) ;
#18559=FACE_OUTER_BOUND ( 'NONE', #16230, .T. ) ;
#18561=ORIENTED_EDGE ( 'NONE', *, *, #15491, .T. ) ;
#18562=CARTESIAN_POINT ( 'NONE',  ( 0.000000000000000000, 0.000000000000000000, 132.4711112102474146 ) ) ;
#18568=ORIENTED_EDGE ( 'NONE', *, *, #14219, .T. ) ;
#18570=DIRECTION ( 'NONE',  ( -0.8660254037844363761, -0.5000000000000039968, -0.000000000000000000 ) ) ;
#18572=EDGE_LOOP ( 'NONE', ( #19588, #16638, #7756, #12332 ) ) ;
#18573=VECTOR ( 'NONE', #1019, 1000.000000000000114 ) ;
#18574=DIRECTION ( 'NONE',  ( 0.000000000000000000, 0.000000000000000000, 1.000000000000000000 ) ) ;
#18575=FACE_OUTER_BOUND ( 'NONE', #17987, .T. ) ;
#18578=ORIENTED_EDGE ( 'NONE', *, *, #1968, .T. ) ;
#18579=CARTESIAN_POINT ( 'NONE',  ( 55.16472960512370349, -30.25670013172234007, 132.4711112102474146 ) ) ;
#18581=PLANE ( 'NONE',  #3815 ) ;
#18584=FACE_OUTER_BOUND ( 'NONE', #9310, .T. ) ;
#18585=LINE ( 'NONE', #6414, #8101 ) ;
#18586=PLANE ( 'NONE',  #15233 ) ;
#18587=VERTEX_POINT ( 'NONE', #12931 ) ;
#18590=ORIENTED_EDGE ( 'NONE', *, *, #12515, .F. ) ;
#18592=CIRCLE ( 'NONE', #1952, 12.50000000000006750 ) ;
#18593=ORIENTED_EDGE ( 'NONE', *, *, #10607, .T. ) ;
#18594=PLANE ( 'NONE',  #8267 ) ;
#18595=VECTOR ( 'NONE', #14698, 1000.000000000000000 ) ;
#18597=VERTEX_POINT ( 'NONE', #462 ) ;
#18598=PLANE ( 'NONE',  #19875 ) ;
#18600=CARTESIAN_POINT ( 'NONE',  ( -5.729042578294540888, -0.2993243175132377365, 283.5832628385307999 ) ) ;
#18601=VERTEX_POINT ( 'NONE', #5077 ) ;
#18603=DIRECTION ( 'NONE',  ( 1.000000000000000000, 0.000000000000000000, 0.000000000000000000 ) ) ;
#18605=VERTEX_POINT ( 'NONE', #2002 ) ;
#18606=CARTESIAN_POINT ( 'NONE',  ( -45.48770046196285932, -37.09555676056982065, 248.9926560891072143 ) ) ;
#18607=DIRECTION ( 'NONE',  ( -0.000000000000000000, -0.000000000000000000, 1.000000000000000000 ) ) ;
#18608=AXIS2_PLACEMENT_3D ( 'NONE', #3536, #2005, #14475 ) ;
#18609=VECTOR ( 'NONE', #5893, 1000.000000000000000 ) ;
#18614=VERTEX_POINT ( 'NONE', #11406 ) ;
#18615=ADVANCED_FACE ( 'NONE', ( #3431 ), #14275, .T. ) ;
#18622=CARTESIAN_POINT ( 'NONE',  ( 0.000000000000000000, 0.000000000000000000, 283.5832628385307999 ) ) ;
#18623=EDGE_LOOP ( 'NONE', ( #14420, #7605, #13436, #7870 ) ) ;
#18626=CARTESIAN_POINT ( 'NONE',  ( 0.000000000000000000, 0.000000000000000000, 293.5832628385307999 ) ) ;
#18629=ORIENTED_EDGE ( 'NONE', *, *, #6418, .T. ) ;
#18630=EDGE_CURVE ( 'NONE', #18719, #10298, #15914, .T. ) ;
#18632=DIRECTION ( 'NONE',  ( -0.000000000000000000, -0.000000000000000000, 1.000000000000000000 ) ) ;
#18633=EDGE_CURVE ( 'NONE', #6205, #16766, #15711, .T. ) ;
#18635=FACE_OUTER_BOUND ( 'NONE', #2124, .T. ) ;
#18636=FACE_OUTER_BOUND ( 'NONE', #19708, .T. ) ;
#18637=ORIENTED_EDGE ( 'NONE', *, *, #9983, .F. ) ;
#18639=AXIS2_PLACEMENT_3D ( 'NONE', #8416, #18031, #13500 ) ;
#18640=DIRECTION ( 'NONE',  ( -0.000000000000000000, -0.000000000000000000, 1.000000000000000000 ) ) ;
#18641=CARTESIAN_POINT ( 'NONE',  ( -50.41613078340781584, 30.05702882063080494, 132.4711112102474146 ) ) ;
#18642=AXIS2_PLACEMENT_3D ( 'NONE', #7877, #3081, #9314 ) ;
#18644=ORIENTED_EDGE ( 'NONE', *, *, #15408, .T. ) ;
#18645=EDGE_CURVE ( 'NONE', #19334, #2821, #13033, .T. ) ;
#18647=DIRECTION ( 'NONE',  ( -0.9781142164131910732, 0.2080686897406944236, 0.000000000000000000 ) ) ;
#18653=FACE_BOUND ( 'NONE', #2296, .T. ) ;
#18654=VERTEX_POINT ( 'NONE', #13318 ) ;
#18656=VECTOR ( 'NONE', #17710, 1000.000000000000114 ) ;
#18658=DIRECTION ( 'NONE',  ( 1.000000000000000000, 0.000000000000000000, 0.000000000000000000 ) ) ;
#18659=CARTESIAN_POINT ( 'NONE',  ( 32.16802499836741447, 54.07248341783265033, 248.9926560891072143 ) ) ;
#18664=DIRECTION ( 'NONE',  ( -0.000000000000000000, -0.000000000000000000, 1.000000000000000000 ) ) ;
#18665=DIRECTION ( 'NONE',  ( 0.000000000000000000, 0.000000000000000000, 1.000000000000000000 ) ) ;
#18666=FACE_OUTER_BOUND ( 'NONE', #6773, .T. ) ;
#18669=DIRECTION ( 'NONE',  ( -0.000000000000000000, -0.000000000000000000, 1.000000000000000000 ) ) ;
#18673=EDGE_CURVE ( 'NONE', #7733, #1943, #16418, .T. ) ;
#18674=CARTESIAN_POINT ( 'NONE',  ( -0.8220851292435327196, -78.26059000578311498, 112.7772637782949943 ) ) ;
#18677=ORIENTED_EDGE ( 'NONE', *, *, #7772, .T. ) ;
#18681=EDGE_CURVE ( 'NONE', #12139, #9304, #11498, .T. ) ;
#18682=CARTESIAN_POINT ( 'NONE',  ( 4.811834253409010387, 3.123743752084098269, 293.5832628385307999 ) ) ;
#18683=CARTESIAN_POINT ( 'NONE',  ( 0.000000000000000000, 0.000000000000000000, 283.5832628385307999 ) ) ;
#18685=CARTESIAN_POINT ( 'NONE',  ( 60.22029172860436574, 7.948651060879242003, 283.5832628385307999 ) ) ;
#18686=CARTESIAN_POINT ( 'NONE',  ( 45.46865632508072963, -40.28046525994365368, 293.5832628385307999 ) ) ;
#18689=CARTESIAN_POINT ( 'NONE',  ( 59.51523122377253117, -12.14914984460739156, 283.5832628385307999 ) ) ;
#18692=CARTESIAN_POINT ( 'NONE',  ( -20.84572577951200500, -54.86954475316249358, 111.4180192758973931 ) ) ;
#18696=VERTEX_POINT ( 'NONE', #17753 ) ;
#18702=DIRECTION ( 'NONE',  ( 0.9396926207859092051, -0.3420201433256662704, -0.000000000000000000 ) ) ;
#18704=CARTESIAN_POINT ( 'NONE',  ( -50.13752642112849855, -30.53958573130890741, 110.9660488491356887 ) ) ;
#18714=AXIS2_PLACEMENT_3D ( 'NONE', #10668, #3215, #9458 ) ;
#18717=DIRECTION ( 'NONE',  ( 0.000000000000000000, 0.000000000000000000, -1.000000000000000000 ) ) ;
#18719=VERTEX_POINT ( 'NONE', #5465 ) ;
#18720=CARTESIAN_POINT ( 'NONE',  ( 0.000000000000000000, 0.000000000000000000, 293.5832628385307999 ) ) ;
#18725=EDGE_LOOP ( 'NONE', ( #15447, #6873, #1037, #3893 ) ) ;
#18727=CARTESIAN_POINT ( 'NONE',  ( 6.445787855800395547E-13, 1.379293853801755176, 248.9926560891072143 ) ) ;
#18728=AXIS2_PLACEMENT_3D ( 'NONE', #10339, #5752, #18128 ) ;
#18732=CARTESIAN_POINT ( 'NONE',  ( -12.78021302872797449, 77.21438937758516374, 132.4711112102474146 ) ) ;
#18734=VECTOR ( 'NONE', #1185, 1000.000000000000000 ) ;
#18736=CARTESIAN_POINT ( 'NONE',  ( -48.72193424476478896, -39.80940113486003185, 132.4711112102474146 ) ) ;
#18737=ORIENTED_EDGE ( 'NONE', *, *, #1272, .T. ) ;
#18740=PLANE ( 'NONE',  #561 ) ;
#18741=DIRECTION ( 'NONE',  ( -0.000000000000000000, -0.000000000000000000, 1.000000000000000000 ) ) ;
#18747=ADVANCED_FACE ( 'NONE', ( #5273 ), #952, .T. ) ;
#18748=ORIENTED_EDGE ( 'NONE', *, *, #19162, .T. ) ;
#18749=ORIENTED_EDGE ( 'NONE', *, *, #4802, .F. ) ;
#18750=ADVANCED_FACE ( 'NONE', ( #10260 ), #16517, .F. ) ;
#18753=CIRCLE ( 'NONE', #5357, 62.91752772691707207 ) ;
#18755=CARTESIAN_POINT ( 'NONE',  ( 0.000000000000000000, 0.000000000000000000, 248.9926560891072143 ) ) ;
#18756=FACE_BOUND ( 'NONE', #7090, .T. ) ;
#18757=AXIS2_PLACEMENT_3D ( 'NONE', #5122, #14422, #19132 ) ;
#18758=VERTEX_POINT ( 'NONE', #16321 ) ;
#18760=CARTESIAN_POINT ( 'NONE',  ( -74.01264520835138683, 25.47058595421627913, 248.9926560891072143 ) ) ;
#18762=ADVANCED_FACE ( 'NONE', ( #19673 ), #18143, .F. ) ;
#18766=LINE ( 'NONE', #1984, #16089 ) ;
#18767=AXIS2_PLACEMENT_3D ( 'NONE', #9949, #9743, #14656 ) ;
#18771=ORIENTED_EDGE ( 'NONE', *, *, #11268, .T. ) ;
#18772=EDGE_CURVE ( 'NONE', #8175, #4586, #2305, .T. ) ;
#18773=CARTESIAN_POINT ( 'NONE',  ( 22.81000261549368346, -58.63718168490493099, 293.5832628385307999 ) ) ;
#18774=VECTOR ( 'NONE', #17352, 1000.000000000000000 ) ;
#18776=EDGE_CURVE ( 'NONE', #3219, #14755, #2696, .T. ) ;
#18778=ORIENTED_EDGE ( 'NONE', *, *, #18004, .T. ) ;
#18779=ORIENTED_EDGE ( 'NONE', *, *, #6786, .T. ) ;
#18782=ADVANCED_FACE ( 'NONE', ( #3110 ), #16812, .F. ) ;
#18783=PLANE ( 'NONE',  #19104 ) ;
#18786=CARTESIAN_POINT ( 'NONE',  ( -0.2993243175131981570, 5.729042578294444077, 293.5832628385307999 ) ) ;
#18789=FACE_OUTER_BOUND ( 'NONE', #2346, .T. ) ;
#18790=VECTOR ( 'NONE', #16041, 1000.000000000000000 ) ;
#18791=DIRECTION ( 'NONE',  ( 0.9848077530122062440, 0.1736481776669404620, 0.000000000000000000 ) ) ;
#18792=EDGE_LOOP ( 'NONE', ( #8318, #15956, #5236 ) ) ;
#18796=DIRECTION ( 'NONE',  ( -0.9781142164131917394, 0.2080686897406911207, 0.000000000000000000 ) ) ;
#18798=EDGE_LOOP ( 'NONE', ( #19839, #2530, #5884, #16229 ) ) ;
#18799=ORIENTED_EDGE ( 'NONE', *, *, #17902, .T. ) ;
#18802=ORIENTED_EDGE ( 'NONE', *, *, #16160, .T. ) ;
#18803=DIRECTION ( 'NONE',  ( 0.5000000000000069944, -0.8660254037844344888, 0.000000000000000000 ) ) ;
#18805=ORIENTED_EDGE ( 'NONE', *, *, #5628, .F. ) ;
#18807=VECTOR ( 'NONE', #1196, 1000.000000000000000 ) ;
#18808=FACE_OUTER_BOUND ( 'NONE', #16881, .T. ) ;
#18811=EDGE_CURVE ( 'NONE', #4702, #14163, #17983, .T. ) ;
#18812=CARTESIAN_POINT ( 'NONE',  ( 7.948937137877743808, -60.22232964560488000, 283.5832628385307999 ) ) ;
#18815=CARTESIAN_POINT ( 'NONE',  ( -28.43859219408707872, 46.49849886828685896, 248.9926560891072143 ) ) ;
#18819=DIRECTION ( 'NONE',  ( 1.000000000000000000, 0.000000000000000000, -0.000000000000000000 ) ) ;
#18822=CARTESIAN_POINT ( 'NONE',  ( 8.938941455415006843, -60.08127757648380651, 283.5832628385307999 ) ) ;
#18823=CARTESIAN_POINT ( 'NONE',  ( 60.72073886220397299, -1.629865514042299734, 283.5832628385307999 ) ) ;
#18828=EDGE_CURVE ( 'NONE', #19621, #14853, #13731, .T. ) ;
#18829=VERTEX_POINT ( 'NONE', #16916 ) ;
#18832=VECTOR ( 'NONE', #607, 1000.000000000000000 ) ;
#18835=ORIENTED_EDGE ( 'NONE', *, *, #16443, .T. ) ;
#18837=LINE ( 'NONE', #18732, #1800 ) ;
#18838=VECTOR ( 'NONE', #201, 1000.000000000000000 ) ;
#18839=CARTESIAN_POINT ( 'NONE',  ( 51.77251465595239921, -31.77296517111717478, 293.5832628385307999 ) ) ;
#18840=CARTESIAN_POINT ( 'NONE',  ( -54.67896814532655725, -21.36933070621745046, 132.4711112102474146 ) ) ;
#18843=CARTESIAN_POINT ( 'NONE',  ( 0.000000000000000000, 0.000000000000000000, 283.5832628385307999 ) ) ;
#18846=ORIENTED_EDGE ( 'NONE', *, *, #15723, .F. ) ;
#18847=CARTESIAN_POINT ( 'NONE',  ( -7.948651060879021735, 60.22029172860445101, 283.5832628385307999 ) ) ;
#18849=VERTEX_POINT ( 'NONE', #19872 ) ;
#18850=EDGE_CURVE ( 'NONE', #7238, #4761, #6883, .T. ) ;
#18851=ORIENTED_EDGE ( 'NONE', *, *, #18919, .F. ) ;
#18854=VERTEX_POINT ( 'NONE', #18347 ) ;
#18856=DIRECTION ( 'NONE',  ( 0.9396926207859069846, 0.3420201433256726542, 0.000000000000000000 ) ) ;
#18857=ORIENTED_EDGE ( 'NONE', *, *, #14116, .F. ) ;
#18859=CARTESIAN_POINT ( 'NONE',  ( 8.939227532413712041, -60.08331549348429235, 283.5832628385307999 ) ) ;
#18862=VECTOR ( 'NONE', #8405, 1000.000000000000000 ) ;
#18863=EDGE_CURVE ( 'NONE', #1487, #17498, #9340, .T. ) ;
#18867=DIRECTION ( 'NONE',  ( 0.7660444431189858960, -0.6427876096865300370, 0.000000000000000000 ) ) ;
#18868=AXIS2_PLACEMENT_3D ( 'NONE', #8287, #15972, #13 ) ;
#18870=FACE_OUTER_BOUND ( 'NONE', #6275, .T. ) ;
#18871=CARTESIAN_POINT ( 'NONE',  ( 0.000000000000000000, 0.000000000000000000, 283.5832628385307999 ) ) ;
#18873=ORIENTED_EDGE ( 'NONE', *, *, #11954, .T. ) ;
#18875=ADVANCED_FACE ( 'NONE', ( #19976 ), #15586, .F. ) ;
#18879=AXIS2_PLACEMENT_3D ( 'NONE', #16668, #2656, #16971 ) ;
#18883=CARTESIAN_POINT ( 'NONE',  ( 0.000000000000000000, 0.000000000000000000, 293.5832628385307999 ) ) ;
#18885=CYLINDRICAL_SURFACE ( 'NONE', #4848, 62.91752772691707207 ) ;
#18888=EDGE_CURVE ( 'NONE', #1786, #14795, #10445, .T. ) ;
#18890=FACE_OUTER_BOUND ( 'NONE', #14594, .T. ) ;
#18893=DIRECTION ( 'NONE',  ( 1.000000000000000000, 0.000000000000000000, 0.000000000000000000 ) ) ;
#18894=CONICAL_SURFACE ( 'NONE', #12670, 62.91752772691707207, 0.5206510040058940358 ) ;
#18895=EDGE_LOOP ( 'NONE', ( #4385, #1159, #14333, #4311 ) ) ;
#18896=AXIS2_PLACEMENT_3D ( 'NONE', #12175, #7375, #18435 ) ;
#18898=CARTESIAN_POINT ( 'NONE',  ( 0.000000000000000000, 0.000000000000000000, 248.9926560891072143 ) ) ;
#18899=VERTEX_POINT ( 'NONE', #20079 ) ;
#18902=VERTEX_POINT ( 'NONE', #20184 ) ;
#18905=VERTEX_POINT ( 'NONE', #6185 ) ;
#18906=DIRECTION ( 'NONE',  ( -0.9993852124581887875, 0.03505990758545896036, 0.000000000000000000 ) ) ;
#18907=VECTOR ( 'NONE', #7866, 1000.000000000000000 ) ;
#18910=VECTOR ( 'NONE', #6673, 1000.000000000000114 ) ;
#18912=ORIENTED_EDGE ( 'NONE', *, *, #9887, .F. ) ;
#18913=EDGE_CURVE ( 'NONE', #20227, #7659, #332, .T. ) ;
#18914=CARTESIAN_POINT ( 'NONE',  ( -68.18670162478832708, -38.41834839689356329, 132.4711112102474146 ) ) ;
#18918=ORIENTED_EDGE ( 'NONE', *, *, #2364, .T. ) ;
#18919=EDGE_CURVE ( 'NONE', #3127, #7889, #15694, .T. ) ;
#18923=PLANE ( 'NONE',  #10599 ) ;
#18924=CIRCLE ( 'NONE', #17942, 62.91752772691707207 ) ;
#18928=AXIS2_PLACEMENT_3D ( 'NONE', #1465, #17120, #36 ) ;
#18931=DIRECTION ( 'NONE',  ( 0.1736481776669404620, -0.9848077530122062440, 0.000000000000000000 ) ) ;
#18932=EDGE_CURVE ( 'NONE', #12045, #13334, #5058, .T. ) ;
#18939=LINE ( 'NONE', #12569, #273 ) ;
#18940=CARTESIAN_POINT ( 'NONE',  ( 29.92423416078111487, 37.80811387934369350, 248.9926560891072143 ) ) ;
#18941=ORIENTED_EDGE ( 'NONE', *, *, #19494, .F. ) ;
#18943=LINE ( 'NONE', #6458, #7349 ) ;
#18945=CARTESIAN_POINT ( 'NONE',  ( 68.46530598706793569, -37.93579148621486041, 132.4711112102474146 ) ) ;
#18948=DIRECTION ( 'NONE',  ( 1.000000000000000000, 0.000000000000000000, 0.000000000000000000 ) ) ;
#18952=DIRECTION ( 'NONE',  ( -0.000000000000000000, -0.000000000000000000, 1.000000000000000000 ) ) ;
#18954=VERTEX_POINT ( 'NONE', #14147 ) ;
#18955=CARTESIAN_POINT ( 'NONE',  ( 0.000000000000000000, 0.000000000000000000, 293.5832628385307999 ) ) ;
#18958=VECTOR ( 'NONE', #11194, 1000.000000000000000 ) ;
#18959=VERTEX_POINT ( 'NONE', #11174 ) ;
#18960=ORIENTED_EDGE ( 'NONE', *, *, #14286, .T. ) ;
#18965=ORIENTED_EDGE ( 'NONE', *, *, #9444, .F. ) ;
#18967=CARTESIAN_POINT ( 'NONE',  ( -73.06915264522019982, -28.06281046684251024, 111.4180192758973931 ) ) ;
#18968=CARTESIAN_POINT ( 'NONE',  ( 50.13752642112827829, 30.53958573130925558, 132.4711112102474146 ) ) ;
#18970=CARTESIAN_POINT ( 'NONE',  ( 77.21438937758502163, 12.78021302872874010, 248.9926560891072143 ) ) ;
#18971=AXIS2_PLACEMENT_3D ( 'NONE', #15270, #9236, #13627 ) ;
#18976=CARTESIAN_POINT ( 'NONE',  ( 50.41613078340802190, -30.05702882063045678, 248.9926560891072143 ) ) ;
#18977=CARTESIAN_POINT ( 'NONE',  ( -2.605298826210328045, -5.111158570922265554, 293.5832628385307999 ) ) ;
#18981=VECTOR ( 'NONE', #13533, 1000.000000000000000 ) ;
#18986=ORIENTED_EDGE ( 'NONE', *, *, #2197, .T. ) ;
#18989=DIRECTION ( 'NONE',  ( 1.000000000000000000, 0.000000000000000000, -0.000000000000000000 ) ) ;
#18995=DIRECTION ( 'NONE',  ( 0.000000000000000000, 0.000000000000000000, 1.000000000000000000 ) ) ;
#18998=CYLINDRICAL_SURFACE ( 'NONE', #1889, 62.91752772691707207 ) ;
#18999=EDGE_LOOP ( 'NONE', ( #13611, #16803, #14880 ) ) ;
#19002=ORIENTED_EDGE ( 'NONE', *, *, #1508, .F. ) ;
#19005=ORIENTED_EDGE ( 'NONE', *, *, #14110, .F. ) ;
#19016=ORIENTED_EDGE ( 'NONE', *, *, #5112, .F. ) ;
#19018=CARTESIAN_POINT ( 'NONE',  ( -4.196299268919061021, -3.911853314815648908, 293.5832628385307999 ) ) ;
#19020=ORIENTED_EDGE ( 'NONE', *, *, #10006, .F. ) ;
#19022=DIRECTION ( 'NONE',  ( -0.000000000000000000, -0.000000000000000000, 1.000000000000000000 ) ) ;
#19024=CARTESIAN_POINT ( 'NONE',  ( 50.93469132750264095, 59.42266395395811429, 110.7293897666001214 ) ) ;
#19027=ORIENTED_EDGE ( 'NONE', *, *, #4018, .T. ) ;
#19028=CARTESIAN_POINT ( 'NONE',  ( 18.77710619359078947, 55.62246070845787216, 111.4180192758974499 ) ) ;
#19030=ORIENTED_EDGE ( 'NONE', *, *, #18681, .F. ) ;
#19036=ORIENTED_EDGE ( 'NONE', *, *, #7399, .F. ) ;
#19041=CARTESIAN_POINT ( 'NONE',  ( -59.42266395395758138, 50.93469132750324491, 248.9926560891072143 ) ) ;
#19042=ADVANCED_FACE ( 'NONE', ( #14556 ), #17932, .T. ) ;
#19046=PLANE ( 'NONE',  #18642 ) ;
#19048=ORIENTED_EDGE ( 'NONE', *, *, #1724, .F. ) ;
#19049=DIRECTION ( 'NONE',  ( -0.000000000000000000, -0.000000000000000000, 1.000000000000000000 ) ) ;
#19054=ORIENTED_EDGE ( 'NONE', *, *, #1354, .T. ) ;
#19055=LINE ( 'NONE', #1660, #8441 ) ;
#19057=EDGE_CURVE ( 'NONE', #7392, #19246, #5349, .T. ) ;
#19058=ORIENTED_EDGE ( 'NONE', *, *, #10379, .F. ) ;
#19060=ORIENTED_EDGE ( 'NONE', *, *, #14526, .T. ) ;
#19061=EDGE_LOOP ( 'NONE', ( #18629, #15052, #2871, #19637 ) ) ;
#19066=ADVANCED_FACE ( 'NONE', ( #7182 ), #10147, .F. ) ;
#19071=LINE ( 'NONE', #14647, #12866 ) ;
#19077=FACE_OUTER_BOUND ( 'NONE', #7455, .T. ) ;
#19079=VERTEX_POINT ( 'NONE', #19271 ) ;
#19084=ORIENTED_EDGE ( 'NONE', *, *, #4359, .F. ) ;
#19085=DIRECTION ( 'NONE',  ( -0.000000000000000000, -0.000000000000000000, 1.000000000000000000 ) ) ;
#19087=CARTESIAN_POINT ( 'NONE',  ( 0.000000000000000000, 0.000000000000000000, 283.5832628385307999 ) ) ;
#19088=VECTOR ( 'NONE', #15689, 1000.000000000000000 ) ;
#19089=DIRECTION ( 'NONE',  ( 1.000000000000000000, 0.000000000000000000, 0.000000000000000000 ) ) ;
#19092=FACE_OUTER_BOUND ( 'NONE', #3070, .T. ) ;
#19094=PLANE ( 'NONE',  #10689 ) ;
#19098=ORIENTED_EDGE ( 'NONE', *, *, #18110, .T. ) ;
#19100=ORIENTED_EDGE ( 'NONE', *, *, #4094, .T. ) ;
#19101=AXIS2_PLACEMENT_3D ( 'NONE', #4933, #11356, #18948 ) ;
#19104=AXIS2_PLACEMENT_3D ( 'NONE', #8123, #1585, #7820 ) ;
#19106=CARTESIAN_POINT ( 'NONE',  ( -62.91215678473957240, 0.8220851292433130064, 248.9926560891072143 ) ) ;
#19108=DIRECTION ( 'NONE',  ( -0.5000000000000039968, 0.8660254037844363761, 0.000000000000000000 ) ) ;
#19111=LINE ( 'NONE', #17684, #18790 ) ;
#19113=ORIENTED_EDGE ( 'NONE', *, *, #5759, .F. ) ;
#19115=DIRECTION ( 'NONE',  ( 0.7660444431189707970, 0.6427876096865481337, 0.000000000000000000 ) ) ;
#19116=PLANE ( 'NONE',  #4890 ) ;
#19118=PLANE ( 'NONE',  #14724 ) ;
#19119=EDGE_CURVE ( 'NONE', #13730, #17, #11578, .T. ) ;
#19123=CARTESIAN_POINT ( 'NONE',  ( 0.000000000000000000, 0.000000000000000000, 248.9926560891072143 ) ) ;
#19125=DIRECTION ( 'NONE',  ( 0.3420201433256568335, 0.9396926207859127578, 0.000000000000000000 ) ) ;
#19129=CARTESIAN_POINT ( 'NONE',  ( 0.000000000000000000, 0.000000000000000000, 293.5832628385307999 ) ) ;
#19132=DIRECTION ( 'NONE',  ( 0.9902903945359623483, 0.1390141521205945918, 0.000000000000000000 ) ) ;
#19135=FACE_OUTER_BOUND ( 'NONE', #3083, .T. ) ;
#19142=DIRECTION ( 'NONE',  ( -0.9396926207859046531, -0.3420201433256790380, 0.000000000000000000 ) ) ;
#19144=FACE_OUTER_BOUND ( 'NONE', #10084, .T. ) ;
#19147=VERTEX_POINT ( 'NONE', #10527 ) ;
#19148=DIRECTION ( 'NONE',  ( -0.9271237148521547233, 0.3747554100459928872, 0.000000000000000000 ) ) ;
#19150=VERTEX_POINT ( 'NONE', #12272 ) ;
#19153=ORIENTED_EDGE ( 'NONE', *, *, #6787, .T. ) ;
#19154=ADVANCED_FACE ( 'NONE', ( #18635 ), #16786, .F. ) ;
#19156=EDGE_CURVE ( 'NONE', #5836, #14900, #4299, .T. ) ;
#19162=EDGE_CURVE ( 'NONE', #9602, #10934, #12167, .T. ) ;
#19164=VECTOR ( 'NONE', #8847, 1000.000000000000114 ) ;
#19169=CARTESIAN_POINT ( 'NONE',  ( -50.13752642112849855, -30.53958573130890741, 132.4711112102474146 ) ) ;
#19172=DIRECTION ( 'NONE',  ( 1.000000000000000000, 0.000000000000000000, 0.000000000000000000 ) ) ;
#19175=ORIENTED_EDGE ( 'NONE', *, *, #1523, .T. ) ;
#19179=AXIS2_PLACEMENT_3D ( 'NONE', #7029, #19505, #5493 ) ;
#19180=EDGE_LOOP ( 'NONE', ( #16156, #8148, #10048, #19450 ) ) ;
#19181=VECTOR ( 'NONE', #13188, 1000.000000000000000 ) ;
#19182=ORIENTED_EDGE ( 'NONE', *, *, #4808, .F. ) ;
#19187=ADVANCED_FACE ( 'NONE', ( #12885 ), #6260, .T. ) ;
#19191=CARTESIAN_POINT ( 'NONE',  ( 56.50329132715945235, -22.30005961346246579, 293.5832628385307999 ) ) ;
#19192=DIRECTION ( 'NONE',  ( 0.000000000000000000, 0.000000000000000000, 1.000000000000000000 ) ) ;
#19193=DIRECTION ( 'NONE',  ( 1.000000000000000000, 0.000000000000000000, 0.000000000000000000 ) ) ;
#19194=CARTESIAN_POINT ( 'NONE',  ( -17.50000000000001066, 2.143131898507869431E-15, 293.5832628385307999 ) ) ;
#19195=ADVANCED_FACE ( 'NONE', ( #15967 ), #19046, .F. ) ;
#19196=ORIENTED_EDGE ( 'NONE', *, *, #16886, .F. ) ;
#19198=VERTEX_POINT ( 'NONE', #1845 ) ;
#19200=ORIENTED_EDGE ( 'NONE', *, *, #2349, .F. ) ;
#19201=VECTOR ( 'NONE', #18669, 1000.000000000000000 ) ;
#19203=ORIENTED_EDGE ( 'NONE', *, *, #12777, .T. ) ;
#19204=DIRECTION ( 'NONE',  ( -0.000000000000000000, -0.000000000000000000, 1.000000000000000000 ) ) ;
#19205=ORIENTED_EDGE ( 'NONE', *, *, #492, .F. ) ;
#19206=LINE ( 'NONE', #2020, #12619 ) ;
#19208=CARTESIAN_POINT ( 'NONE',  ( -18.28503710798546678, 57.92514141135458772, 293.5832628385307999 ) ) ;
#19209=DIRECTION ( 'NONE',  ( 0.000000000000000000, 0.000000000000000000, 1.000000000000000000 ) ) ;
#19210=ORIENTED_EDGE ( 'NONE', *, *, #12390, .F. ) ;
#19212=DIRECTION ( 'NONE',  ( 0.9848077530122062440, 0.1736481776669404620, 0.000000000000000000 ) ) ;
#19216=LINE ( 'NONE', #8254, #6105 ) ;
#19220=CARTESIAN_POINT ( 'NONE',  ( -68.18670162478832708, -38.41834839689356329, 110.9660488491356887 ) ) ;
#19225=DIRECTION ( 'NONE',  ( -0.8479630283625716469, 0.5300553768524345344, 0.000000000000000000 ) ) ;
#19226=ORIENTED_EDGE ( 'NONE', *, *, #10634, .T. ) ;
#19227=AXIS2_PLACEMENT_3D ( 'NONE', #5789, #2715, #7610 ) ;
#19230=AXIS2_PLACEMENT_3D ( 'NONE', #8396, #4081, #16575 ) ;
#19233=CARTESIAN_POINT ( 'NONE',  ( 60.22232964560483737, 7.948937137877944537, 283.5832628385307999 ) ) ;
#19238=CYLINDRICAL_SURFACE ( 'NONE', #1592, 60.74260934110282051 ) ;
#19240=VECTOR ( 'NONE', #2396, 1000.000000000000227 ) ;
#19241=VECTOR ( 'NONE', #9292, 1000.000000000000000 ) ;
#19242=ADVANCED_FACE ( 'NONE', ( #3183 ), #12576, .F. ) ;
#19244=LINE ( 'NONE', #12788, #13199 ) ;
#19246=VERTEX_POINT ( 'NONE', #17408 ) ;
#19249=CARTESIAN_POINT ( 'NONE',  ( -76.83212392882499842, -14.94814811854936565, 248.9926560891072143 ) ) ;
#19250=PLANE ( 'NONE',  #2063 ) ;
#19260=VECTOR ( 'NONE', #15402, 1000.000000000000000 ) ;
#19261=ORIENTED_EDGE ( 'NONE', *, *, #16634, .F. ) ;
#19264=DIRECTION ( 'NONE',  ( 0.5000000000000069944, -0.8660254037844344888, 0.000000000000000000 ) ) ;
#19266=DIRECTION ( 'NONE',  ( 0.3420201433256568335, 0.9396926207859126468, 0.000000000000000000 ) ) ;
#19267=DIRECTION ( 'NONE',  ( 1.000000000000000000, 0.000000000000000000, 0.000000000000000000 ) ) ;
#19270=EDGE_CURVE ( 'NONE', #11697, #10402, #203, .T. ) ;
#19271=CARTESIAN_POINT ( 'NONE',  ( -41.02212542604613787, -44.79787735033403351, 293.5832628385307999 ) ) ;
#19273=DIRECTION ( 'NONE',  ( -0.8660254037844432595, 0.4999999999999919509, -0.000000000000000000 ) ) ;
#19274=LINE ( 'NONE', #18977, #17036 ) ;
#19277=AXIS2_PLACEMENT_3D ( 'NONE', #7000, #13417, #13625 ) ;
#19279=LINE ( 'NONE', #12614, #14771 ) ;
#19280=VERTEX_POINT ( 'NONE', #6665 ) ;
#19281=EDGE_CURVE ( 'NONE', #19327, #5832, #9714, .T. ) ;
#19282=EDGE_CURVE ( 'NONE', #9602, #11122, #10834, .T. ) ;
#19288=DIRECTION ( 'NONE',  ( 0.5000000000000009992, -0.8660254037844380415, 0.000000000000000000 ) ) ;
#19290=CARTESIAN_POINT ( 'NONE',  ( -59.42266395395758138, 50.93469132750324491, 110.7293897666001214 ) ) ;
#19292=DIRECTION ( 'NONE',  ( 0.000000000000000000, 0.000000000000000000, -1.000000000000000000 ) ) ;
#19293=DIRECTION ( 'NONE',  ( 0.9396926207859046531, 0.3420201433256790380, 0.000000000000000000 ) ) ;
#19296=ORIENTED_EDGE ( 'NONE', *, *, #247, .T. ) ;
#19299=VERTEX_POINT ( 'NONE', #15867 ) ;
#19300=VERTEX_POINT ( 'NONE', #6565 ) ;
#19302=EDGE_CURVE ( 'NONE', #11985, #11567, #12787, .T. ) ;
#19304=EDGE_LOOP ( 'NONE', ( #14104, #5216, #11709, #9605 ) ) ;
#19305=DIRECTION ( 'NONE',  ( 0.000000000000000000, -0.000000000000000000, 1.000000000000000000 ) ) ;
#19307=EDGE_CURVE ( 'NONE', #15836, #15975, #19439, .T. ) ;
#19308=DIRECTION ( 'NONE',  ( -0.9396926207859092051, 0.3420201433256662704, 0.000000000000000000 ) ) ;
#19309=DIRECTION ( 'NONE',  ( 0.8660254037844449249, -0.4999999999999888978, 0.000000000000000000 ) ) ;
#19311=ORIENTED_EDGE ( 'NONE', *, *, #19958, .F. ) ;
#19313=LINE ( 'NONE', #14695, #12926 ) ;
#19314=CARTESIAN_POINT ( 'NONE',  ( 62.91215678473958661, -0.8220851292428736912, 293.5832628385307999 ) ) ;
#19315=ORIENTED_EDGE ( 'NONE', *, *, #14538, .T. ) ;
#19316=LINE ( 'NONE', #12860, #18184 ) ;
#19320=CARTESIAN_POINT ( 'NONE',  ( -23.22718332831480481, -56.12853591711337486, 283.5832628385307999 ) ) ;
#19322=ORIENTED_EDGE ( 'NONE', *, *, #13214, .F. ) ;
#19326=AXIS2_PLACEMENT_3D ( 'NONE', #6693, #16097, #19172 ) ;
#19327=VERTEX_POINT ( 'NONE', #905 ) ;
#19331=FACE_OUTER_BOUND ( 'NONE', #13538, .T. ) ;
#19333=FACE_OUTER_BOUND ( 'NONE', #11562, .T. ) ;
#19334=VERTEX_POINT ( 'NONE', #13271 ) ;
#19337=DIRECTION ( 'NONE',  ( 0.2080686897406943681, 0.9781142164131909622, 0.000000000000000000 ) ) ;
#19339=EDGE_LOOP ( 'NONE', ( #12422, #7400, #11462 ) ) ;
#19342=LINE ( 'NONE', #17812, #18308 ) ;
#19344=EDGE_LOOP ( 'NONE', ( #3175, #7731, #1884, #6378 ) ) ;
#19345=CARTESIAN_POINT ( 'NONE',  ( 44.79940644582654841, -41.02350267428983699, 293.5832628385307999 ) ) ;
#19348=ORIENTED_EDGE ( 'NONE', *, *, #11528, .T. ) ;
#19349=ORIENTED_EDGE ( 'NONE', *, *, #18277, .F. ) ;
#19351=ADVANCED_FACE ( 'NONE', ( #11648 ), #3777, .F. ) ;
#19352=DIRECTION ( 'NONE',  ( 0.000000000000000000, 0.000000000000000000, -1.000000000000000000 ) ) ;
#19354=ORIENTED_EDGE ( 'NONE', *, *, #5846, .F. ) ;
#19355=AXIS2_PLACEMENT_3D ( 'NONE', #4879, #11094, #17357 ) ;
#19361=CARTESIAN_POINT ( 'NONE',  ( 50.41613078340802190, -30.05702882063045678, 110.9660488491357455 ) ) ;
#19362=EDGE_CURVE ( 'NONE', #3773, #8985, #3586, .T. ) ;
#19363=LINE ( 'NONE', #5350, #18384 ) ;
#19368=EDGE_LOOP ( 'NONE', ( #19016, #19772, #10040, #20013 ) ) ;
#19369=EDGE_CURVE ( 'NONE', #1965, #3545, #13078, .T. ) ;
#19371=CIRCLE ( 'NONE', #1049, 62.91752772691707207 ) ;
#19372=VECTOR ( 'NONE', #2162, 1000.000000000000227 ) ;
#19374=ORIENTED_EDGE ( 'NONE', *, *, #3143, .F. ) ;
#19377=DIRECTION ( 'NONE',  ( 0.6427876096865481337, -0.7660444431189707970, 0.000000000000000000 ) ) ;
#19378=DIRECTION ( 'NONE',  ( -1.000000000000000000, -1.047444401652940007E-14, -0.000000000000000000 ) ) ;
#19379=AXIS2_PLACEMENT_3D ( 'NONE', #1237, #6272, #1554 ) ;
#19380=DIRECTION ( 'NONE',  ( 0.4999999999999978906, 0.8660254037844397068, 0.000000000000000000 ) ) ;
#19382=CARTESIAN_POINT ( 'NONE',  ( 3.453261854573465683, 4.581103194070611728, 293.5832628385307999 ) ) ;
#19383=DIRECTION ( 'NONE',  ( 0.1736481776669241417, 0.9848077530122091305, 0.000000000000000000 ) ) ;
#19387=EDGE_CURVE ( 'NONE', #18385, #14947, #5423, .T. ) ;
#19388=LINE ( 'NONE', #7103, #11183 ) ;
#19389=EDGE_CURVE ( 'NONE', #15308, #5361, #17610, .T. ) ;
#19392=CARTESIAN_POINT ( 'NONE',  ( 8.939227532413712041, -60.08331549348429235, 293.5832628385307999 ) ) ;
#19394=EDGE_LOOP ( 'NONE', ( #11644, #18851, #12368, #15622 ) ) ;
#19395=VERTEX_POINT ( 'NONE', #11554 ) ;
#19396=AXIS2_PLACEMENT_3D ( 'NONE', #20138, #5828, #4186 ) ;
#19397=ORIENTED_EDGE ( 'NONE', *, *, #1653, .F. ) ;
#19398=ORIENTED_EDGE ( 'NONE', *, *, #6650, .T. ) ;
#19399=LINE ( 'NONE', #11609, #9921 ) ;
#19400=EDGE_CURVE ( 'NONE', #13334, #7829, #17807, .T. ) ;
#19401=ORIENTED_EDGE ( 'NONE', *, *, #3037, .F. ) ;
#19403=DIRECTION ( 'NONE',  ( 0.000000000000000000, 0.000000000000000000, 1.000000000000000000 ) ) ;
#19407=VERTEX_POINT ( 'NONE', #10123 ) ;
#19408=FACE_OUTER_BOUND ( 'NONE', #9976, .T. ) ;
#19409=CARTESIAN_POINT ( 'NONE',  ( 47.56244194535165093, 37.78198917157335757, 283.5832628385307999 ) ) ;
#19414=CIRCLE ( 'NONE', #784, 60.74260934110282051 ) ;
#19417=LINE ( 'NONE', #15843, #16055 ) ;
#19418=EDGE_CURVE ( 'NONE', #12841, #15923, #16040, .T. ) ;
#19420=AXIS2_PLACEMENT_3D ( 'NONE', #4958, #15893, #11175 ) ;
#19421=CARTESIAN_POINT ( 'NONE',  ( 0.000000000000000000, 0.000000000000000000, 283.5832628385307999 ) ) ;
#19428=ORIENTED_EDGE ( 'NONE', *, *, #14259, .F. ) ;
#19432=PLANE ( 'NONE',  #4704 ) ;
#19434=DIRECTION ( 'NONE',  ( -0.6427876096865430267, 0.7660444431189749048, 0.000000000000000000 ) ) ;
#19437=DIRECTION ( 'NONE',  ( -0.3088643371590125697, 0.9511061040868803440, 0.000000000000000000 ) ) ;
#19439=LINE ( 'NONE', #6952, #11135 ) ;
#19440=DIRECTION ( 'NONE',  ( 0.3420201433256602197, 0.9396926207859115365, 0.000000000000000000 ) ) ;
#19442=LINE ( 'NONE', #10216, #6454 ) ;
#19449=DIRECTION ( 'NONE',  ( -0.4693298356057531429, 0.8830229359480288309, 0.000000000000000000 ) ) ;
#19450=ORIENTED_EDGE ( 'NONE', *, *, #18353, .T. ) ;
#19452=ORIENTED_EDGE ( 'NONE', *, *, #17519, .T. ) ;
#19453=ORIENTED_EDGE ( 'NONE', *, *, #2012, .T. ) ;
#19454=CARTESIAN_POINT ( 'NONE',  ( -76.92888220842476699, 14.39940464655786201, 132.4711112102474146 ) ) ;
#19455=ORIENTED_EDGE ( 'NONE', *, *, #18132, .T. ) ;
#19460=CARTESIAN_POINT ( 'NONE',  ( 67.08601213326538470, 40.32479851956839667, 110.9660488491356887 ) ) ;
#19464=CARTESIAN_POINT ( 'NONE',  ( -5.693982670708919613, 0.7000608949449674823, 293.5832628385307999 ) ) ;
#19465=DIRECTION ( 'NONE',  ( -3.491481338843133355E-15, 1.000000000000000000, 0.000000000000000000 ) ) ;
#19466=CARTESIAN_POINT ( 'NONE',  ( 49.67518383744835120, -60.47951622432767493, 248.9926560891072143 ) ) ;
#19467=EDGE_CURVE ( 'NONE', #10138, #10141, #14722, .T. ) ;
#19471=VECTOR ( 'NONE', #10427, 999.9999999999998863 ) ;
#19472=ORIENTED_EDGE ( 'NONE', *, *, #10019, .F. ) ;
#19473=ORIENTED_EDGE ( 'NONE', *, *, #5875, .T. ) ;
#19474=EDGE_CURVE ( 'NONE', #1414, #6346, #13173, .T. ) ;
#19479=FACE_OUTER_BOUND ( 'NONE', #7012, .T. ) ;
#19482=LINE ( 'NONE', #17754, #4780 ) ;
#19483=CARTESIAN_POINT ( 'NONE',  ( 53.78543575132128751, 32.64570716507559212, 293.5832628385307999 ) ) ;
#19492=ORIENTED_EDGE ( 'NONE', *, *, #6918, .T. ) ;
#19493=AXIS2_PLACEMENT_3D ( 'NONE', #16946, #15407, #3139 ) ;
#19494=EDGE_CURVE ( 'NONE', #18829, #9325, #14071, .T. ) ;
#19495=ORIENTED_EDGE ( 'NONE', *, *, #13395, .F. ) ;
#19498=CARTESIAN_POINT ( 'NONE',  ( 60.22232964560483737, 7.948937137877944537, 293.5832628385307999 ) ) ;
#19501=DIRECTION ( 'NONE',  ( -0.000000000000000000, -0.000000000000000000, 1.000000000000000000 ) ) ;
#19503=VERTEX_POINT ( 'NONE', #6103 ) ;
#19504=CARTESIAN_POINT ( 'NONE',  ( 19.30071112029679625, -55.43188410062176530, 111.4180192758973362 ) ) ;
#19505=DIRECTION ( 'NONE',  ( 0.7430374143461900838, -0.6692498792541753394, 0.000000000000000000 ) ) ;
#19506=LINE ( 'NONE', #5494, #627 ) ;
#19507=DIRECTION ( 'NONE',  ( -0.1736481776669340227, 0.9848077530122073542, 0.000000000000000000 ) ) ;
#19508=AXIS2_PLACEMENT_3D ( 'NONE', #3591, #9718, #3187 ) ;
#19510=CARTESIAN_POINT ( 'NONE',  ( 0.000000000000000000, 0.000000000000000000, 132.4711112102474146 ) ) ;
#19511=CARTESIAN_POINT ( 'NONE',  ( 36.99514631729018532, -48.17959877923561862, 283.5832628385307999 ) ) ;
#19512=ORIENTED_EDGE ( 'NONE', *, *, #6119, .F. ) ;
#19514=VERTEX_POINT ( 'NONE', #12319 ) ;
#19518=EDGE_CURVE ( 'NONE', #11442, #14900, #2313, .T. ) ;
#19519=VECTOR ( 'NONE', #11324, 1000.000000000000000 ) ;
#19522=VECTOR ( 'NONE', #2755, 1000.000000000000000 ) ;
#19524=DIRECTION ( 'NONE',  ( 0.000000000000000000, 0.000000000000000000, -1.000000000000000000 ) ) ;
#19530=CARTESIAN_POINT ( 'NONE',  ( 0.000000000000000000, 0.000000000000000000, 293.5832628385307999 ) ) ;
#19533=EDGE_CURVE ( 'NONE', #4430, #8683, #9472, .T. ) ;
#19537=AXIS2_PLACEMENT_3D ( 'NONE', #5484, #2514, #17974 ) ;
#19540=DIRECTION ( 'NONE',  ( -0.03505990758545545621, -0.9993852124581888985, 0.000000000000000000 ) ) ;
#19541=CARTESIAN_POINT ( 'NONE',  ( 23.22641211976290876, 56.12662799072082720, 283.5832628385307999 ) ) ;
#19542=EDGE_LOOP ( 'NONE', ( #1064, #7914, #3864, #963 ) ) ;
#19545=CARTESIAN_POINT ( 'NONE',  ( 0.000000000000000000, 0.000000000000000000, 283.5832628385307999 ) ) ;
#19550=VECTOR ( 'NONE', #14916, 1000.000000000000227 ) ;
#19552=AXIS2_PLACEMENT_3D ( 'NONE', #13382, #8688, #3891 ) ;
#19555=DIRECTION ( 'NONE',  ( 0.4999999999999888978, 0.8660254037844449249, 0.000000000000000000 ) ) ;
#19557=CARTESIAN_POINT ( 'NONE',  ( 0.000000000000000000, 0.000000000000000000, 248.9926560891072143 ) ) ;
#19561=VECTOR ( 'NONE', #5927, 1000.000000000000000 ) ;
#19562=AXIS2_PLACEMENT_3D ( 'NONE', #7127, #7223, #5692 ) ;
#19563=VERTEX_POINT ( 'NONE', #9161 ) ;
#19566=ORIENTED_EDGE ( 'NONE', *, *, #8971, .F. ) ;
#19568=VECTOR ( 'NONE', #17733, 1000.000000000000000 ) ;
#19572=DIRECTION ( 'NONE',  ( -0.9993852124581887875, 0.03505990758545896036, 0.000000000000000000 ) ) ;
#19574=VECTOR ( 'NONE', #8455, 1000.000000000000000 ) ;
#19579=CARTESIAN_POINT ( 'NONE',  ( 10.11498556985161024, -62.09913334491128012, 248.9926560891072143 ) ) ;
#19580=CARTESIAN_POINT ( 'NONE',  ( 60.08331549348424971, 8.939227532413909216, 293.5832628385307999 ) ) ;
#19583=EDGE_LOOP ( 'NONE', ( #18099, #11611, #19428, #3765 ) ) ;
#19586=VECTOR ( 'NONE', #10449, 1000.000000000000000 ) ;
#19587=ORIENTED_EDGE ( 'NONE', *, *, #6746, .F. ) ;
#19588=ORIENTED_EDGE ( 'NONE', *, *, #3602, .F. ) ;
#19589=EDGE_CURVE ( 'NONE', #19198, #3495, #4672, .T. ) ;
#19590=DIRECTION ( 'NONE',  ( 0.9848077530122085754, -0.1736481776669273336, 0.000000000000000000 ) ) ;
#19591=DIRECTION ( 'NONE',  ( -0.6427876096865300370, -0.7660444431189858960, 0.000000000000000000 ) ) ;
#19594=CARTESIAN_POINT ( 'NONE',  ( -62.18629025319808790, 9.564549117045718418, 132.4711112102474146 ) ) ;
#19596=ADVANCED_FACE ( 'NONE', ( #11931 ), #16943, .T. ) ;
#19597=DIRECTION ( 'NONE',  ( 1.000000000000000000, 0.000000000000000000, 0.000000000000000000 ) ) ;
#19598=DIRECTION ( 'NONE',  ( 0.000000000000000000, 0.000000000000000000, -1.000000000000000000 ) ) ;
#19599=CARTESIAN_POINT ( 'NONE',  ( 3.911853314815638694, -4.196299268919047698, 293.5832628385307999 ) ) ;
#19603=EDGE_CURVE ( 'NONE', #20212, #5133, #12530, .T. ) ;
#19606=CARTESIAN_POINT ( 'NONE',  ( -77.21438937758512111, -12.78021302872824094, 132.4711112102474146 ) ) ;
#19607=ORIENTED_EDGE ( 'NONE', *, *, #17778, .T. ) ;
#19608=EDGE_CURVE ( 'NONE', #18849, #15505, #18097, .T. ) ;
#19610=VERTEX_POINT ( 'NONE', #7827 ) ;
#19611=EDGE_LOOP ( 'NONE', ( #19182, #17760, #10917, #4083 ) ) ;
#19612=CARTESIAN_POINT ( 'NONE',  ( 30.74413178637192701, -54.89456854707552935, 293.5832628385307999 ) ) ;
#19615=AXIS2_PLACEMENT_3D ( 'NONE', #8382, #709, #5230 ) ;
#19616=ADVANCED_FACE ( 'NONE', ( #18789 ), #11834, .T. ) ;
#19617=FACE_OUTER_BOUND ( 'NONE', #17263, .T. ) ;
#19618=CARTESIAN_POINT ( 'NONE',  ( -5.111158570922240685, 2.605298826210305840, 293.5832628385307999 ) ) ;
#19620=LINE ( 'NONE', #16660, #15523 ) ;
#19621=VERTEX_POINT ( 'NONE', #16119 ) ;
#19622=LINE ( 'NONE', #18094, #16242 ) ;
#19627=EDGE_LOOP ( 'NONE', ( #14464, #6845, #5803, #15593 ) ) ;
#19628=LINE ( 'NONE', #13082, #7730 ) ;
#19632=PLANE ( 'NONE',  #17080 ) ;
#19635=DIRECTION ( 'NONE',  ( 0.000000000000000000, 0.000000000000000000, 1.000000000000000000 ) ) ;
#19637=ORIENTED_EDGE ( 'NONE', *, *, #9659, .T. ) ;
#19638=VERTEX_POINT ( 'NONE', #6712 ) ;
#19640=VERTEX_POINT ( 'NONE', #357 ) ;
#19642=AXIS2_PLACEMENT_3D ( 'NONE', #2776, #16992, #9104 ) ;
#19644=DIRECTION ( 'NONE',  ( 1.000000000000000000, 0.000000000000000000, 0.000000000000000000 ) ) ;
#19647=CARTESIAN_POINT ( 'NONE',  ( 2.629250726500717672, 60.68567895461850270, 293.5832628385307999 ) ) ;
#19652=CARTESIAN_POINT ( 'NONE',  ( -60.83768308848344475, 49.24833719034248958, 248.9926560891072143 ) ) ;
#19654=ADVANCED_FACE ( 'NONE', ( #14278 ), #12096, .T. ) ;
#19655=EDGE_LOOP ( 'NONE', ( #8650, #299, #16378, #8470 ) ) ;
#19656=LINE ( 'NONE', #15053, #5492 ) ;
#19663=LINE ( 'NONE', #8717, #3161 ) ;
#19666=DIRECTION ( 'NONE',  ( -0.4999999999999950040, -0.8660254037844415942, 0.000000000000000000 ) ) ;
#19667=DIRECTION ( 'NONE',  ( 0.000000000000000000, 0.000000000000000000, 1.000000000000000000 ) ) ;
#19673=FACE_OUTER_BOUND ( 'NONE', #1219, .T. ) ;
#19676=VECTOR ( 'NONE', #9750, 1000.000000000000114 ) ;
#19677=AXIS2_PLACEMENT_3D ( 'NONE', #17514, #14019, #1746 ) ;
#19678=FACE_OUTER_BOUND ( 'NONE', #4916, .T. ) ;
#19680=ORIENTED_EDGE ( 'NONE', *, *, #4212, .F. ) ;
#19683=VERTEX_POINT ( 'NONE', #1899 ) ;
#19686=AXIS2_PLACEMENT_3D ( 'NONE', #1357, #18443, #4422 ) ;
#19689=DIRECTION ( 'NONE',  ( 0.000000000000000000, 0.000000000000000000, -1.000000000000000000 ) ) ;
#19691=VECTOR ( 'NONE', #18803, 1000.000000000000227 ) ;
#19692=CYLINDRICAL_SURFACE ( 'NONE', #11625, 62.91752772691707207 ) ;
#19693=DIRECTION ( 'NONE',  ( 1.000000000000000000, 0.000000000000000000, 0.000000000000000000 ) ) ;
#19694=ORIENTED_EDGE ( 'NONE', *, *, #2142, .F. ) ;
#19695=DIRECTION ( 'NONE',  ( -0.000000000000000000, -0.000000000000000000, 1.000000000000000000 ) ) ;
#19698=DIRECTION ( 'NONE',  ( -0.7430374143461878633, 0.6692498792541777819, 0.000000000000000000 ) ) ;
#19700=VERTEX_POINT ( 'NONE', #4881 ) ;
#19705=ORIENTED_EDGE ( 'NONE', *, *, #17560, .T. ) ;
#19706=CARTESIAN_POINT ( 'NONE',  ( 28.06680738835026290, -53.87178215532764369, 283.5832628385307999 ) ) ;
#19707=AXIS2_PLACEMENT_3D ( 'NONE', #177, #9685, #6228 ) ;
#19708=EDGE_LOOP ( 'NONE', ( #10843, #18513, #18487, #11841 ) ) ;
#19709=ORIENTED_EDGE ( 'NONE', *, *, #3956, .F. ) ;
#19712=DIRECTION ( 'NONE',  ( 0.3420201433256631063, 0.9396926207859105373, 0.000000000000000000 ) ) ;
#19714=CARTESIAN_POINT ( 'NONE',  ( 0.000000000000000000, 0.000000000000000000, 248.9926560891072143 ) ) ;
#19719=FACE_OUTER_BOUND ( 'NONE', #16239, .T. ) ;
#19720=VECTOR ( 'NONE', #329, 1000.000000000000114 ) ;
#19722=CARTESIAN_POINT ( 'NONE',  ( -51.36153797460868731, 59.06449708980215263, 110.7293897666001214 ) ) ;
#19723=ORIENTED_EDGE ( 'NONE', *, *, #3840, .T. ) ;
#19724=VECTOR ( 'NONE', #8741, 1000.000000000000114 ) ;
#19730=CARTESIAN_POINT ( 'NONE',  ( -12.14914984460759761, -59.51523122377249564, 293.5832628385307999 ) ) ;
#19738=ADVANCED_FACE ( 'NONE', ( #7104 ), #17960, .F. ) ;
#19739=LINE ( 'NONE', #19454, #11960 ) ;
#19745=ADVANCED_FACE ( 'NONE', ( #2604 ), #10265, .T. ) ;
#19748=DIRECTION ( 'NONE',  ( -0.000000000000000000, -0.000000000000000000, 1.000000000000000000 ) ) ;
#19749=LINE ( 'NONE', #13398, #15827 ) ;
#19750=CARTESIAN_POINT ( 'NONE',  ( 44.79940644582654841, -41.02350267428983699, 283.5832628385307999 ) ) ;
#19752=CARTESIAN_POINT ( 'NONE',  ( -50.93469132750304595, -59.42266395395774481, 110.7293897666001214 ) ) ;
#19753=ORIENTED_EDGE ( 'NONE', *, *, #1201, .T. ) ;
#19757=EDGE_LOOP ( 'NONE', ( #19761, #8982, #4465, #8866 ) ) ;
#19761=ORIENTED_EDGE ( 'NONE', *, *, #493, .F. ) ;
#19763=VERTEX_POINT ( 'NONE', #13224 ) ;
#19767=EDGE_CURVE ( 'NONE', #13329, #18614, #17373, .T. ) ;
#19768=CARTESIAN_POINT ( 'NONE',  ( 28.94983032429829350, -53.40245231972188833, 283.5832628385307999 ) ) ;
#19770=CARTESIAN_POINT ( 'NONE',  ( -5.729042578294415655, -0.2993243175132198064, 293.5832628385307999 ) ) ;
#19771=DIRECTION ( 'NONE',  ( -0.9511061040868794558, -0.3088643371590157338, 0.000000000000000000 ) ) ;
#19772=ORIENTED_EDGE ( 'NONE', *, *, #506, .T. ) ;
#19776=DIRECTION ( 'NONE',  ( 1.000000000000000000, 0.000000000000000000, 0.000000000000000000 ) ) ;
#19781=LINE ( 'NONE', #1055, #7579 ) ;
#19782=ORIENTED_EDGE ( 'NONE', *, *, #1426, .F. ) ;
#19783=VERTEX_POINT ( 'NONE', #19579 ) ;
#19785=EDGE_LOOP ( 'NONE', ( #13638, #12126, #19705, #16742 ) ) ;
#19788=CARTESIAN_POINT ( 'NONE',  ( -1.379293853801755176, 62.90240729679781850, 248.9926560891072143 ) ) ;
#19791=CARTESIAN_POINT ( 'NONE',  ( 60.08331549348424971, 8.939227532413909216, 293.5832628385307999 ) ) ;
#19793=DIRECTION ( 'NONE',  ( -0.9396926207859114255, 0.3420201433256601087, -0.000000000000000000 ) ) ;
#19797=LINE ( 'NONE', #5794, #7160 ) ;
#19798=FACE_OUTER_BOUND ( 'NONE', #12991, .T. ) ;
#19803=FACE_OUTER_BOUND ( 'NONE', #18389, .T. ) ;
#19805=VECTOR ( 'NONE', #18796, 1000.000000000000114 ) ;
#19807=ORIENTED_EDGE ( 'NONE', *, *, #17991, .F. ) ;
#19808=ORIENTED_EDGE ( 'NONE', *, *, #12902, .F. ) ;
#19809=CARTESIAN_POINT ( 'NONE',  ( 51.24071425735604635, -32.61983739937743110, 293.5832628385307999 ) ) ;
#19810=ORIENTED_EDGE ( 'NONE', *, *, #10467, .F. ) ;
#19813=VECTOR ( 'NONE', #15780, 1000.000000000000114 ) ;
#19814=CARTESIAN_POINT ( 'NONE',  ( 14.94814811854963210, -76.83212392882498420, 132.4711112102474146 ) ) ;
#19815=CARTESIAN_POINT ( 'NONE',  ( -48.17797692984161984, -36.99387960884178028, 283.5832628385307999 ) ) ;
#19817=CARTESIAN_POINT ( 'NONE',  ( 56.50138340076688337, -22.29928840491054132, 293.5832628385307999 ) ) ;
#19821=LINE ( 'NONE', #8579, #4812 ) ;
#19822=CYLINDRICAL_SURFACE ( 'NONE', #9754, 62.91752772691707207 ) ;
#19824=ORIENTED_EDGE ( 'NONE', *, *, #498, .T. ) ;
#19828=ORIENTED_EDGE ( 'NONE', *, *, #12850, .F. ) ;
#19830=PLANE ( 'NONE',  #12519 ) ;
#19831=ORIENTED_EDGE ( 'NONE', *, *, #20235, .T. ) ;
#19836=ORIENTED_EDGE ( 'NONE', *, *, #15723, .T. ) ;
#19837=CARTESIAN_POINT ( 'NONE',  ( 51.77251465595239921, -31.77296517111717478, 293.5832628385307999 ) ) ;
#19839=ORIENTED_EDGE ( 'NONE', *, *, #7875, .T. ) ;
#19841=DIRECTION ( 'NONE',  ( -0.000000000000000000, -0.000000000000000000, 1.000000000000000000 ) ) ;
#19842=ADVANCED_FACE ( 'NONE', ( #19678 ), #2500, .F. ) ;
#19846=PLANE ( 'NONE',  #19642 ) ;
#19847=CYLINDRICAL_SURFACE ( 'NONE', #13186, 79.75827554147308263 ) ;
#19851=DIRECTION ( 'NONE',  ( -0.3420201433256757628, 0.9396926207859058744, 0.000000000000000000 ) ) ;
#19853=ORIENTED_EDGE ( 'NONE', *, *, #12390, .T. ) ;
#19854=EDGE_CURVE ( 'NONE', #14032, #9758, #5934, .T. ) ;
#19855=CARTESIAN_POINT ( 'NONE',  ( -79.75827554147308263, 9.767571684737763671E-15, 293.5832628385307999 ) ) ;
#19856=LINE ( 'NONE', #10749, #17087 ) ;
#19858=ORIENTED_EDGE ( 'NONE', *, *, #10582, .F. ) ;
#19859=EDGE_CURVE ( 'NONE', #18228, #12122, #11473, .T. ) ;
#19860=ORIENTED_EDGE ( 'NONE', *, *, #15480, .F. ) ;
#19864=ORIENTED_EDGE ( 'NONE', *, *, #4347, .F. ) ;
#19868=DIRECTION ( 'NONE',  ( -0.000000000000000000, -0.000000000000000000, 1.000000000000000000 ) ) ;
#19871=EDGE_LOOP ( 'NONE', ( #8881, #13612, #18590, #6916 ) ) ;
#19872=CARTESIAN_POINT ( 'NONE',  ( -22.29928840491073316, -56.50138340076681231, 283.5832628385307999 ) ) ;
#19875=AXIS2_PLACEMENT_3D ( 'NONE', #3052, #9068, #10911 ) ;
#19878=VECTOR ( 'NONE', #4021, 1000.000000000000000 ) ;
#19882=AXIS2_PLACEMENT_3D ( 'NONE', #4349, #10577, #1287 ) ;
#19884=EDGE_CURVE ( 'NONE', #8089, #2316, #15485, .T. ) ;
#19886=ORIENTED_EDGE ( 'NONE', *, *, #12870, .T. ) ;
#19887=EDGE_CURVE ( 'NONE', #6652, #6960, #13735, .T. ) ;
#19888=ORIENTED_EDGE ( 'NONE', *, *, #19156, .F. ) ;
#19889=ORIENTED_EDGE ( 'NONE', *, *, #7749, .T. ) ;
#19890=ORIENTED_EDGE ( 'NONE', *, *, #11146, .F. ) ;
#19892=VECTOR ( 'NONE', #1819, 1000.000000000000000 ) ;
#19895=LINE ( 'NONE', #19791, #13651 ) ;
#19896=ORIENTED_EDGE ( 'NONE', *, *, #11164, .F. ) ;
#19898=DIRECTION ( 'NONE',  ( 1.000000000000000000, 0.000000000000000000, 0.000000000000000000 ) ) ;
#19899=ORIENTED_EDGE ( 'NONE', *, *, #3384, .T. ) ;
#19901=DIRECTION ( 'NONE',  ( 0.6155349844899687950, -0.7881095627315619634, 0.000000000000000000 ) ) ;
#19913=LINE ( 'NONE', #18287, #18734 ) ;
#19914=EDGE_LOOP ( 'NONE', ( #18846, #10755, #1995, #2732 ) ) ;
#19916=LINE ( 'NONE', #4369, #10083 ) ;
#19921=DIRECTION ( 'NONE',  ( -0.000000000000000000, -0.000000000000000000, 1.000000000000000000 ) ) ;
#19922=CARTESIAN_POINT ( 'NONE',  ( 54.07248341783254375, -32.16802499836760632, 132.4711112102474146 ) ) ;
#19925=PLANE ( 'NONE',  #4198 ) ;
#19928=FACE_OUTER_BOUND ( 'NONE', #2748, .T. ) ;
#19932=VECTOR ( 'NONE', #16375, 1000.000000000000000 ) ;
#19936=ORIENTED_EDGE ( 'NONE', *, *, #14984, .T. ) ;
#19937=VECTOR ( 'NONE', #11072, 1000.000000000000114 ) ;
#19939=CARTESIAN_POINT ( 'NONE',  ( -28.06281046684226155, 73.06915264522029929, 111.4180192758973931 ) ) ;
#19941=CARTESIAN_POINT ( 'NONE',  ( -3.911853314815648908, 4.196299268919088554, 293.5832628385307999 ) ) ;
#19942=PLANE ( 'NONE',  #1747 ) ;
#19943=EDGE_LOOP ( 'NONE', ( #17989, #14263, #7095, #11313 ) ) ;
#19945=CARTESIAN_POINT ( 'NONE',  ( 0.000000000000000000, 17.50000000000001066, 83.57543755549745867 ) ) ;
#19946=VECTOR ( 'NONE', #19698, 1000.000000000000114 ) ;
#19947=VECTOR ( 'NONE', #6759, 1000.000000000000114 ) ;
#19949=CARTESIAN_POINT ( 'NONE',  ( 0.000000000000000000, 0.000000000000000000, 293.5832628385307999 ) ) ;
#19954=ORIENTED_EDGE ( 'NONE', *, *, #10775, .F. ) ;
#19956=CARTESIAN_POINT ( 'NONE',  ( -61.70726652483826058, -12.28122767885825084, 293.5832628385307999 ) ) ;
#19958=EDGE_CURVE ( 'NONE', #4164, #12652, #3113, .T. ) ;
#19959=AXIS2_PLACEMENT_3D ( 'NONE', #16069, #9918, #16169 ) ;
#19962=VECTOR ( 'NONE', #18350, 1000.000000000000000 ) ;
#19963=ORIENTED_EDGE ( 'NONE', *, *, #14156, .T. ) ;
#19964=FACE_BOUND ( 'NONE', #16531, .T. ) ;
#19965=ORIENTED_EDGE ( 'NONE', *, *, #18772, .F. ) ;
#19966=DIRECTION ( 'NONE',  ( 0.000000000000000000, 0.000000000000000000, 1.000000000000000000 ) ) ;
#19967=CARTESIAN_POINT ( 'NONE',  ( 28.63313560863472063, -51.23821591265105013, 132.4711112102474146 ) ) ;
#19969=EDGE_CURVE ( 'NONE', #3588, #9534, #6291, .T. ) ;
#19971=ADVANCED_FACE ( 'NONE', ( #4327 ), #10664, .T. ) ;
#19972=DIRECTION ( 'NONE',  ( -0.1736481776669207000, -0.9848077530122097967, 0.000000000000000000 ) ) ;
#19973=CYLINDRICAL_SURFACE ( 'NONE', #18928, 17.50000000000001066 ) ;
#19974=ORIENTED_EDGE ( 'NONE', *, *, #601, .F. ) ;
#19975=EDGE_CURVE ( 'NONE', #6026, #18385, #5978, .T. ) ;
#19976=FACE_OUTER_BOUND ( 'NONE', #19655, .T. ) ;
#19979=DIRECTION ( 'NONE',  ( -0.4999999999999950040, -0.8660254037844415942, 0.000000000000000000 ) ) ;
#19983=EDGE_CURVE ( 'NONE', #4216, #19621, #16815, .T. ) ;
#19984=ORIENTED_EDGE ( 'NONE', *, *, #6874, .T. ) ;
#19985=ORIENTED_EDGE ( 'NONE', *, *, #17241, .T. ) ;
#19986=ORIENTED_EDGE ( 'NONE', *, *, #16637, .T. ) ;
#19988=EDGE_CURVE ( 'NONE', #18469, #1901, #1574, .T. ) ;
#19991=EDGE_LOOP ( 'NONE', ( #20049, #11098, #13882, #15719 ) ) ;
#19992=VECTOR ( 'NONE', #256, 1000.000000000000000 ) ;
#19995=DIRECTION ( 'NONE',  ( -0.03505990758545545621, -0.9993852124581888985, 0.000000000000000000 ) ) ;
#19998=CYLINDRICAL_SURFACE ( 'NONE', #19882, 62.91752772691707207 ) ;
#20001=AXIS2_PLACEMENT_3D ( 'NONE', #8788, #10130, #16279 ) ;
#20002=LINE ( 'NONE', #12223, #17028 ) ;
#20003=AXIS2_PLACEMENT_3D ( 'NONE', #18222, #8902, #15456 ) ;
#20006=ORIENTED_EDGE ( 'NONE', *, *, #12516, .F. ) ;
#20007=ORIENTED_EDGE ( 'NONE', *, *, #14234, .F. ) ;
#20011=VECTOR ( 'NONE', #20057, 1000.000000000000000 ) ;
#20013=ORIENTED_EDGE ( 'NONE', *, *, #4154, .F. ) ;
#20014=CARTESIAN_POINT ( 'NONE',  ( -73.25972925305609351, 27.53920554013712874, 111.4180192758973931 ) ) ;
#20018=FACE_OUTER_BOUND ( 'NONE', #18999, .T. ) ;
#20019=CYLINDRICAL_SURFACE ( 'NONE', #5677, 60.74260934110282051 ) ;
#20021=ORIENTED_EDGE ( 'NONE', *, *, #4288, .F. ) ;
#20022=EDGE_CURVE ( 'NONE', #15118, #17837, #17127, .T. ) ;
#20023=ADVANCED_FACE ( 'NONE', ( #7499 ), #12301, .F. ) ;
#20025=LINE ( 'NONE', #4904, #17306 ) ;
#20026=ADVANCED_FACE ( 'NONE', ( #18870 ), #12813, .F. ) ;
#20027=ORIENTED_EDGE ( 'NONE', *, *, #8274, .F. ) ;
#20031=AXIS2_PLACEMENT_3D ( 'NONE', #13896, #16870, #12255 ) ;
#20033=LINE ( 'NONE', #18404, #5399 ) ;
#20035=VECTOR ( 'NONE', #1251, 999.9999999999998863 ) ;
#20038=ORIENTED_EDGE ( 'NONE', *, *, #12976, .T. ) ;
#20040=FACE_OUTER_BOUND ( 'NONE', #9350, .T. ) ;
#20049=ORIENTED_EDGE ( 'NONE', *, *, #2417, .F. ) ;
#20052=CARTESIAN_POINT ( 'NONE',  ( 0.000000000000000000, 0.000000000000000000, 283.5832628385307999 ) ) ;
#20055=DIRECTION ( 'NONE',  ( -0.3420201433256757073, 0.9396926207859057634, 0.000000000000000000 ) ) ;
#20056=LINE ( 'NONE', #16993, #11581 ) ;
#20057=DIRECTION ( 'NONE',  ( 0.000000000000000000, 0.000000000000000000, -1.000000000000000000 ) ) ;
#20063=LINE ( 'NONE', #19956, #10869 ) ;
#20065=AXIS2_PLACEMENT_3D ( 'NONE', #14224, #17611, #3386 ) ;
#20066=VERTEX_POINT ( 'NONE', #9845 ) ;
#20067=VECTOR ( 'NONE', #9465, 1000.000000000000000 ) ;
#20071=CARTESIAN_POINT ( 'NONE',  ( -39.37628763770455009, -49.07263256785938665, 132.4711112102474146 ) ) ;
#20073=DIRECTION ( 'NONE',  ( 0.5060387318153625191, 6.197187131622696351E-17, -0.8625107546591518348 ) ) ;
#20075=AXIS2_PLACEMENT_3D ( 'NONE', #5520, #17808, #3778 ) ;
#20076=FACE_OUTER_BOUND ( 'NONE', #13190, .T. ) ;
#20077=CARTESIAN_POINT ( 'NONE',  ( 0.000000000000000000, 0.000000000000000000, 248.9926560891072143 ) ) ;
#20078=ADVANCED_FACE ( 'NONE', ( #14456 ), #17444, .T. ) ;
#20079=CARTESIAN_POINT ( 'NONE',  ( -20.21777810286715749, -59.58067424803620327, 132.4711112102474146 ) ) ;
#20086=PLANE ( 'NONE',  #18714 ) ;
#20088=ADVANCED_FACE ( 'NONE', ( #9647 ), #238, .F. ) ;
#20090=CIRCLE ( 'NONE', #6057, 62.91752772691707207 ) ;
#20091=ORIENTED_EDGE ( 'NONE', *, *, #8638, .F. ) ;
#20093=CARTESIAN_POINT ( 'NONE',  ( -9.564549117045517690, -62.18629025319811632, 132.4711112102474146 ) ) ;
#20094=LINE ( 'NONE', #15080, #8634 ) ;
#20097=AXIS2_PLACEMENT_3D ( 'NONE', #13908, #6151, #7770 ) ;
#20106=FACE_OUTER_BOUND ( 'NONE', #14514, .T. ) ;
#20108=CARTESIAN_POINT ( 'NONE',  ( 37.78325588002174840, -47.56406379474564972, 293.5832628385307999 ) ) ;
#20110=EDGE_LOOP ( 'NONE', ( #7283, #2484, #12578, #10269 ) ) ;
#20111=ADVANCED_FACE ( 'NONE', ( #15896 ), #16376, .T. ) ;
#20113=AXIS2_PLACEMENT_3D ( 'NONE', #10498, #15316, #16752 ) ;
#20114=VERTEX_POINT ( 'NONE', #6592 ) ;
#20115=EDGE_CURVE ( 'NONE', #1303, #9432, #337, .T. ) ;
#20116=DIRECTION ( 'NONE',  ( 0.000000000000000000, 0.000000000000000000, -1.000000000000000000 ) ) ;
#20119=DIRECTION ( 'NONE',  ( 1.000000000000000000, 0.000000000000000000, -0.000000000000000000 ) ) ;
#20120=CARTESIAN_POINT ( 'NONE',  ( 19.30071112029679625, -55.43188410062176530, 248.9926560891072143 ) ) ;
#20122=EDGE_LOOP ( 'NONE', ( #18080, #5089, #5610, #5442 ) ) ;
#20123=DIRECTION ( 'NONE',  ( 1.000000000000000000, 0.000000000000000000, 0.000000000000000000 ) ) ;
#20124=CARTESIAN_POINT ( 'NONE',  ( -76.92888220842476699, 14.39940464655785313, 132.4711112102474146 ) ) ;
#20126=EDGE_LOOP ( 'NONE', ( #11466, #12244, #18360, #16662 ) ) ;
#20130=CARTESIAN_POINT ( 'NONE',  ( 53.87178215532755132, 28.06680738835045119, 283.5832628385307999 ) ) ;
#20131=CARTESIAN_POINT ( 'NONE',  ( 7.948651060879040386, -60.22029172860440127, 293.5832628385307999 ) ) ;
#20132=VECTOR ( 'NONE', #18379, 1000.000000000000000 ) ;
#20134=FACE_OUTER_BOUND ( 'NONE', #3791, .T. ) ;
#20137=LINE ( 'NONE', #12254, #12336 ) ;
#20138=CARTESIAN_POINT ( 'NONE',  ( 0.000000000000000000, 79.75827554147308263, 132.4711112102474146 ) ) ;
#20139=EDGE_LOOP ( 'NONE', ( #11423, #3091, #7530, #16457 ) ) ;
#20144=EDGE_CURVE ( 'NONE', #12002, #937, #15998, .T. ) ;
#20147=AXIS2_PLACEMENT_3D ( 'NONE', #19545, #6876, #920 ) ;
#20148=ORIENTED_EDGE ( 'NONE', *, *, #5394, .F. ) ;
#20150=DIRECTION ( 'NONE',  ( 0.000000000000000000, 0.000000000000000000, 1.000000000000000000 ) ) ;
#20153=CARTESIAN_POINT ( 'NONE',  ( 62.91215678473958661, -0.8220851292428736912, 132.4711112102474146 ) ) ;
#20154=ADVANCED_FACE ( 'NONE', ( #1985 ), #5256, .F. ) ;
#20155=ADVANCED_FACE ( 'NONE', ( #7905 ), #14152, .F. ) ;
#20158=VERTEX_POINT ( 'NONE', #8708 ) ;
#20159=PLANE ( 'NONE',  #9221 ) ;
#20163=ORIENTED_EDGE ( 'NONE', *, *, #1389, .F. ) ;
#20164=VECTOR ( 'NONE', #11228, 1000.000000000000114 ) ;
#20165=DIRECTION ( 'NONE',  ( 0.000000000000000000, 0.000000000000000000, 1.000000000000000000 ) ) ;
#20166=DIRECTION ( 'NONE',  ( -0.6427876096865353661, -0.7660444431189813441, -0.000000000000000000 ) ) ;
#20167=EDGE_CURVE ( 'NONE', #19300, #858, #11582, .T. ) ;
#20171=ORIENTED_EDGE ( 'NONE', *, *, #10775, .T. ) ;
#20174=LINE ( 'NONE', #9440, #4457 ) ;
#20175=EDGE_LOOP ( 'NONE', ( #4213, #1283, #11699, #6501 ) ) ;
#20176=LINE ( 'NONE', #9333, #2074 ) ;
#20177=CARTESIAN_POINT ( 'NONE',  ( 62.91752772691707207, 0.000000000000000000, 83.57543755549745867 ) ) ;
#20179=CIRCLE ( 'NONE', #5808, 60.74260934110282051 ) ;
#20180=AXIS2_PLACEMENT_3D ( 'NONE', #19510, #6738, #9998 ) ;
#20182=CARTESIAN_POINT ( 'NONE',  ( 37.78325588002174840, -47.56406379474564972, 293.5832628385307999 ) ) ;
#20183=CARTESIAN_POINT ( 'NONE',  ( 0.000000000000000000, 0.000000000000000000, 293.5832628385307999 ) ) ;
#20184=CARTESIAN_POINT ( 'NONE',  ( 47.66508197439472383, -41.06890862491489003, 248.9926560891072143 ) ) ;
#20187=DIRECTION ( 'NONE',  ( 0.8660254037844432595, -0.4999999999999919509, 0.000000000000000000 ) ) ;
#20198=CARTESIAN_POINT ( 'NONE',  ( 60.22232964560483737, 7.948937137877944537, 293.5832628385307999 ) ) ;
#20199=VERTEX_POINT ( 'NONE', #16497 ) ;
#20201=DIRECTION ( 'NONE',  ( -0.6692498792541753394, -0.7430374143461900838, 0.000000000000000000 ) ) ;
#20202=AXIS2_PLACEMENT_3D ( 'NONE', #4481, #10712, #16966 ) ;
#20203=ORIENTED_EDGE ( 'NONE', *, *, #6134, .F. ) ;
#20209=DIRECTION ( 'NONE',  ( -0.9511061040868804550, -0.3088643371590125697, 0.000000000000000000 ) ) ;
#20210=LINE ( 'NONE', #3138, #13966 ) ;
#20212=VERTEX_POINT ( 'NONE', #19464 ) ;
#20213=VERTEX_POINT ( 'NONE', #16590 ) ;
#20214=ORIENTED_EDGE ( 'NONE', *, *, #6635, .F. ) ;
#20215=AXIS2_PLACEMENT_3D ( 'NONE', #17097, #19851, #3086 ) ;
#20216=VECTOR ( 'NONE', #15713, 1000.000000000000000 ) ;
#20219=EDGE_CURVE ( 'NONE', #1302, #3145, #17833, .T. ) ;
#20221=AXIS2_PLACEMENT_3D ( 'NONE', #8433, #662, #13119 ) ;
#20222=ORIENTED_EDGE ( 'NONE', *, *, #10036, .T. ) ;
#20227=VERTEX_POINT ( 'NONE', #10240 ) ;
#20230=ORIENTED_EDGE ( 'NONE', *, *, #12630, .T. ) ;
#20232=EDGE_CURVE ( 'NONE', #347, #1021, #2575, .T. ) ;
#20233=LINE ( 'NONE', #18606, #9690 ) ;
#20234=CARTESIAN_POINT ( 'NONE',  ( 0.000000000000000000, 0.000000000000000000, 293.5832628385307999 ) ) ;
#20235=EDGE_CURVE ( 'NONE', #4517, #4430, #16201, .T. ) ;
#20240=CARTESIAN_POINT ( 'NONE',  ( 57.61823435390807902, 19.23677882349220880, 293.5832628385307999 ) ) ;
#20241=CARTESIAN_POINT ( 'NONE',  ( 0.000000000000000000, 0.000000000000000000, 248.9926560891072143 ) ) ;
ENDSEC;
END-ISO-10303-21;
